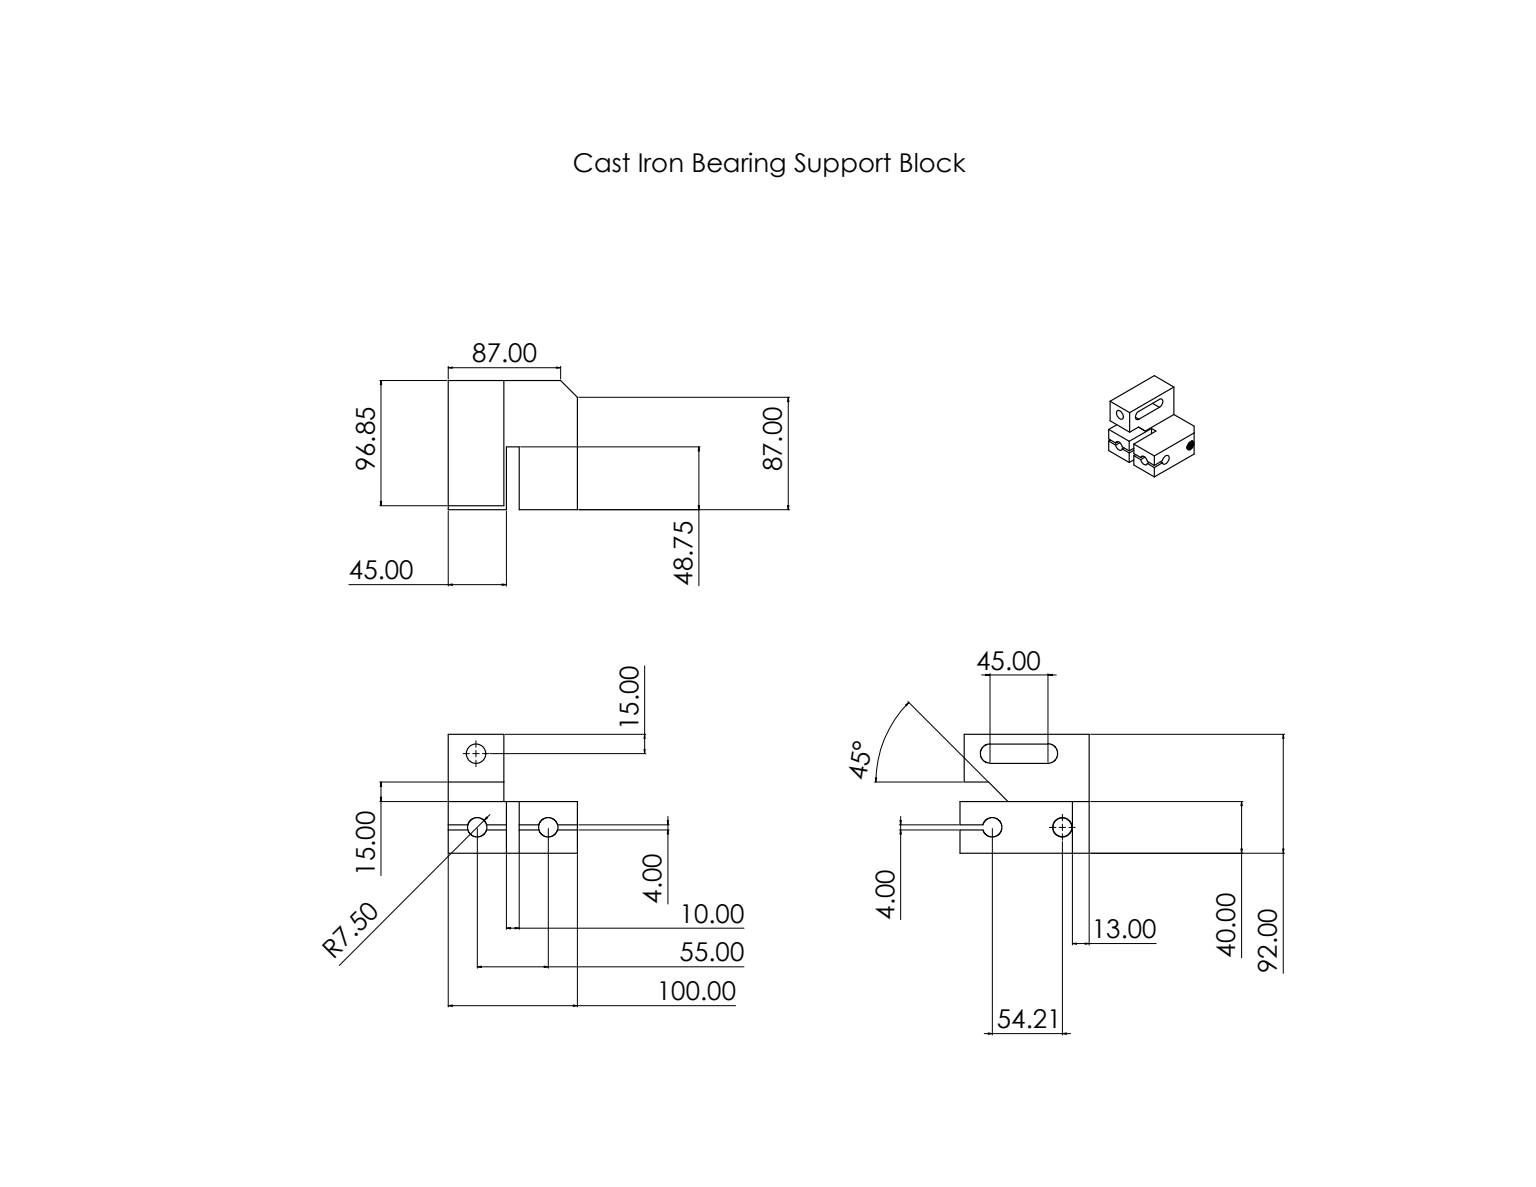
ISO-10303-21;
HEADER;
FILE_DESCRIPTION (('STEP AP214'),
    '1' );
FILE_NAME ('Cast Iron Bearing Support Block.step',
    '2026-10-19T17:36:30',
    ( '' ),
    ( '' ),
    'SwSTEP 2.0',
    'SolidWorks 2025',
    '' );
FILE_SCHEMA (( 'AUTOMOTIVE_DESIGN' ));
ENDSEC;

DATA;
#1=CARTESIAN_POINT ( 'NONE',  ( 38.97500000054622404, 24.28113015263587471, 84.90069139318163138 ) ) ;
#2=CARTESIAN_POINT ( 'NONE',  ( 27.17500000054621978, 26.19570976099943493, 86.29171490190961435 ) ) ;
#3=CARTESIAN_POINT ( 'NONE',  ( 23.09999999999998721, 22.43689772174679575, 83.29316153445363113 ) ) ;
#4=CARTESIAN_POINT ( 'NONE',  ( 19.93750000027310421, 20.00000000000000355, 98.18490835945361539 ) ) ;
#5=CARTESIAN_POINT ( 'NONE',  ( 32.97500000054622404, 24.28113015263587471, 84.90069139318163138 ) ) ;
#6=ORIENTED_EDGE ( 'NONE', *, *, #525, .T. ) ;
#10=VERTEX_POINT ( 'NONE', #4037 ) ;
#11=CARTESIAN_POINT ( 'NONE',  ( 49.45000000109246940, 24.40838939219354842, 96.86078899226572503 ) ) ;
#13=CARTESIAN_POINT ( 'NONE',  ( 43.29999999999999005, 26.37988106264029398, 86.15790661882942914 ) ) ;
#16=CARTESIAN_POINT ( 'NONE',  ( 43.67500000054621978, 24.28113015263587116, 96.68563167572563088 ) ) ;
#19=CARTESIAN_POINT ( 'NONE',  ( -50.00000000000001421, 18.00000000000000355, 188.4007504869563263 ) ) ;
#20=CARTESIAN_POINT ( 'NONE',  ( 46.77500000054622831, 17.63344945572770328, 83.50966788445364841 ) ) ;
#21=CARTESIAN_POINT ( 'NONE',  ( 48.49999999999999289, 12.11403331821300533, 90.79316153445363113 ) ) ;
#22=DIRECTION ( 'NONE',  ( -1.000000000000000000, -9.251858538542971828E-16, 0.000000000000000000 ) ) ;
#23=CARTESIAN_POINT ( 'NONE',  ( 44.29999999999999005, 13.62011893735970958, 95.42841645007781892 ) ) ;
#24=ORIENTED_EDGE ( 'NONE', *, *, #11626, .T. ) ;
#25=CARTESIAN_POINT ( 'NONE',  ( 31.75000000109246656, 17.56310227825320425, 98.29316153445363113 ) ) ;
#27=ORIENTED_EDGE ( 'NONE', *, *, #5795, .F. ) ;
#31=CARTESIAN_POINT ( 'NONE',  ( -27.49999999999999645, 20.00000000000000355, 169.9999999999999716 ) ) ;
#33=CARTESIAN_POINT ( 'NONE',  ( -2.000000000000015543, 20.00000000000000355, 83.29316153445364534 ) ) ;
#34=CARTESIAN_POINT ( 'NONE',  ( 36.27500000054623541, 12.34168156654572535, 90.79316153445363113 ) ) ;
#35=CARTESIAN_POINT ( 'NONE',  ( 34.77500000054622831, 17.63344945572770328, 83.50966788445364841 ) ) ;
#37=CARTESIAN_POINT ( 'NONE',  ( 35.55000000109245661, 22.43689772174678154, 98.29316153445364534 ) ) ;
#40=ORIENTED_EDGE ( 'NONE', *, *, #1850, .F. ) ;
#41=CARTESIAN_POINT ( 'NONE',  ( 48.57500000054622546, 13.80429023900056684, 86.29171490190961435 ) ) ;
#44=DIRECTION ( 'NONE',  ( 0.000000000000000000, 0.000000000000000000, -1.000000000000000000 ) ) ;
#45=DIRECTION ( 'NONE',  ( -1.000000000000000000, 0.000000000000000000, -0.000000000000000000 ) ) ;
#48=CARTESIAN_POINT ( 'NONE',  ( 43.05000000109246372, 27.13292387221364876, 88.47553407664153724 ) ) ;
#51=CARTESIAN_POINT ( 'NONE',  ( 6.614339767079327359, 27.50003396314175674, 91.05027562884485803 ) ) ;
#52=CARTESIAN_POINT ( 'NONE',  ( 37.79999999999998295, 24.40838939219354842, 96.86078899226572503 ) ) ;
#53=VECTOR ( 'NONE', #12398, 999.9999999999998863 ) ;
#54=CARTESIAN_POINT ( 'NONE',  ( 49.99999999999998579, 22.00000000000000000, 169.9999999999999716 ) ) ;
#58=VERTEX_POINT ( 'NONE', #304 ) ;
#59=CARTESIAN_POINT ( 'NONE',  ( 37.25000000109246656, 27.13292387221364876, 93.11078899226573924 ) ) ;
#61=CARTESIAN_POINT ( 'NONE',  ( 23.07500000054622546, 24.28113015263587471, 84.90069139318163138 ) ) ;
#62=CARTESIAN_POINT ( 'NONE',  ( 23.85000000109246443, 15.59161060780645691, 96.86078899226572503 ) ) ;
#63=VECTOR ( 'NONE', #11751, 1000.000000000000000 ) ;
#64=CARTESIAN_POINT ( 'NONE',  ( 37.57500000054622546, 24.28113015263587116, 96.68563167572563088 ) ) ;
#65=CARTESIAN_POINT ( 'NONE',  ( 21.57500000054622546, 26.19570976099943493, 95.29460816699764791 ) ) ;
#66=CARTESIAN_POINT ( 'NONE',  ( 21.49999999999998224, 27.88596668178699645, 90.79316153445363113 ) ) ;
#68=CARTESIAN_POINT ( 'NONE',  ( 31.47500000054623115, 26.19570976099943493, 95.29460816699764791 ) ) ;
#69=ORIENTED_EDGE ( 'NONE', *, *, #4429, .F. ) ;
#70=LINE ( 'NONE', #9907, #9738 ) ;
#73=EDGE_LOOP ( 'NONE', ( #2091, #4719, #3113, #69, #4677 ) ) ;
#77=DIRECTION ( 'NONE',  ( 1.000000000000000000, -0.000000000000000000, -0.000000000000000000 ) ) ;
#79=CARTESIAN_POINT ( 'NONE',  ( -2.000000000000015543, 20.00000000000000355, 90.79316153445363113 ) ) ;
#80=CARTESIAN_POINT ( 'NONE',  ( 44.17500000054621978, 13.80429023900056507, 95.29460816699764791 ) ) ;
#81=CARTESIAN_POINT ( 'NONE',  ( 39.95000000109245519, 13.62011893735970958, 95.42841645007781892 ) ) ;
#82=DIRECTION ( 'NONE',  ( 0.000000000000000000, 0.000000000000000000, -1.000000000000000000 ) ) ;
#83=CARTESIAN_POINT ( 'NONE',  ( 45.47500000054622404, 26.92701409722686634, 93.04388485072563242 ) ) ;
#84=CARTESIAN_POINT ( 'NONE',  ( 45.29999999999999005, 26.37988106264029398, 86.15790661882942914 ) ) ;
#87=CARTESIAN_POINT ( 'NONE',  ( 44.99999999999999289, 20.00000000000000355, 83.29316153445364534 ) ) ;
#88=CARTESIAN_POINT ( 'NONE',  ( 44.09999999999999432, 17.56310227825318648, 98.29316153445363113 ) ) ;
#91=CARTESIAN_POINT ( 'NONE',  ( 31.65000000109246514, 20.00000000000000355, 98.29316153445363113 ) ) ;
#92=DIRECTION ( 'NONE',  ( -1.000000000000000000, 0.000000000000000000, 0.000000000000000000 ) ) ;
#93=EDGE_LOOP ( 'NONE', ( #11616, #6758, #10652, #3781, #4940 ) ) ;
#94=EDGE_CURVE ( 'NONE', #11777, #315, #4411, .T. ) ;
#95=ORIENTED_EDGE ( 'NONE', *, *, #9864, .T. ) ;
#96=DIRECTION ( 'NONE',  ( 1.000000000000000000, -0.000000000000000000, -0.000000000000000000 ) ) ;
#101=CARTESIAN_POINT ( 'NONE',  ( 38.37500000054622973, 13.07298590277314432, 88.54243821818161564 ) ) ;
#102=CARTESIAN_POINT ( 'NONE',  ( 31.17500000054621978, 26.19570976099943493, 86.29171490190961435 ) ) ;
#103=CARTESIAN_POINT ( 'NONE',  ( 34.65000000109246514, 20.00000000000000355, 83.29316153445364534 ) ) ;
#107=CARTESIAN_POINT ( 'NONE',  ( 49.77500000054621410, 22.36655054427230027, 98.07665518445361386 ) ) ;
#109=LINE ( 'NONE', #11712, #6790 ) ;
#110=VERTEX_POINT ( 'NONE', #7455 ) ;
#111=CARTESIAN_POINT ( 'NONE',  ( 31.89339828220178674, 12.50000000000000888, 140.6066017177982133 ) ) ;
#113=VERTEX_POINT ( 'NONE', #8411 ) ;
#114=EDGE_LOOP ( 'NONE', ( #10765, #3378, #1409, #9629, #7659 ) ) ;
#116=CARTESIAN_POINT ( 'NONE',  ( -34.72841614740048044, 22.00000000000000000, 152.2284161474004520 ) ) ;
#118=CARTESIAN_POINT ( 'NONE',  ( 6.732665147703623454, 27.39438278699427087, 92.07235497779568334 ) ) ;
#123=CARTESIAN_POINT ( 'NONE',  ( 43.27500000054623541, 27.65831843345427998, 90.79316153445363113 ) ) ;
#125=CARTESIAN_POINT ( 'NONE',  ( 27.49999999999999645, 20.00000000000000355, 169.9999999999999716 ) ) ;
#129=CARTESIAN_POINT ( 'NONE',  ( 46.19999999999998863, 15.59161060780645691, 96.86078899226572503 ) ) ;
#131=CARTESIAN_POINT ( 'NONE',  ( 30.37500000054622973, 13.07298590277314432, 88.54243821818161564 ) ) ;
#132=CARTESIAN_POINT ( 'NONE',  ( 22.17500000054622333, 13.80429023900056507, 95.29460816699764791 ) ) ;
#133=CARTESIAN_POINT ( 'NONE',  ( 24.89999999999999147, 17.56310227825321135, 83.29316153445363113 ) ) ;
#135=CARTESIAN_POINT ( 'NONE',  ( 33.07500000054623257, 26.19570976099943493, 86.29171490190961435 ) ) ;
#136=VERTEX_POINT ( 'NONE', #11263 ) ;
#137=DIRECTION ( 'NONE',  ( 0.000000000000000000, -0.000000000000000000, 1.000000000000000000 ) ) ;
#140=DIRECTION ( 'NONE',  ( 1.000000000000000000, -0.000000000000000000, -0.000000000000000000 ) ) ;
#146=CARTESIAN_POINT ( 'NONE',  ( 38.17500000054622689, 13.80429023900056507, 95.29460816699764791 ) ) ;
#148=CARTESIAN_POINT ( 'NONE',  ( 26.79999999999998650, 15.59161060780646046, 84.72553407664153724 ) ) ;
#149=CARTESIAN_POINT ( 'NONE',  ( 42.07500000054622546, 15.71886984736413417, 96.68563167572563088 ) ) ;
#150=CARTESIAN_POINT ( 'NONE',  ( 43.89999999999999147, 22.43689772174679575, 98.29316153445363113 ) ) ;
#152=LINE ( 'NONE', #11692, #6762 ) ;
#154=ORIENTED_EDGE ( 'NONE', *, *, #8754, .F. ) ;
#155=CARTESIAN_POINT ( 'NONE',  ( 33.65000000109246514, 20.00000000000000355, 98.29316153445363113 ) ) ;
#159=CARTESIAN_POINT ( 'NONE',  ( 25.65000000109246514, 20.00000000000000355, 98.29316153445363113 ) ) ;
#162=DIRECTION ( 'NONE',  ( 1.000000000000000000, -0.000000000000000000, -0.000000000000000000 ) ) ;
#163=CARTESIAN_POINT ( 'NONE',  ( 48.09999999999999432, 17.56310227825322556, 98.29316153445364534 ) ) ;
#164=CARTESIAN_POINT ( 'NONE',  ( 32.87500000054622973, 22.36655054427230382, 83.50966788445364841 ) ) ;
#165=CARTESIAN_POINT ( 'NONE',  ( 29.87500000054622618, 20.00000000000000355, 98.07665518445361386 ) ) ;
#167=CARTESIAN_POINT ( 'NONE',  ( 44.05000000109246372, 12.86707612778636012, 93.11078899226572503 ) ) ;
#171=CARTESIAN_POINT ( 'NONE',  ( 21.99999999999998934, 20.00000000000000355, 98.29316153445363113 ) ) ;
#172=ORIENTED_EDGE ( 'NONE', *, *, #1724, .F. ) ;
#176=ORIENTED_EDGE ( 'NONE', *, *, #7484, .F. ) ;
#179=EDGE_CURVE ( 'NONE', #6763, #7138, #1054, .T. ) ;
#180=CARTESIAN_POINT ( 'NONE',  ( 9.920725400334921673, 21.28151498972171751, 98.18721253656565295 ) ) ;
#181=LINE ( 'NONE', #4040, #1401 ) ;
#186=CARTESIAN_POINT ( 'NONE',  ( 40.67500000054623399, 17.63344945572770328, 83.50966788445364841 ) ) ;
#187=DIRECTION ( 'NONE',  ( 0.000000000000000000, 0.000000000000000000, 1.000000000000000000 ) ) ;
#189=EDGE_CURVE ( 'NONE', #5728, #3198, #1007, .T. ) ;
#193=CARTESIAN_POINT ( 'NONE',  ( 20.47500000054622404, 13.07298590277314432, 88.54243821818161564 ) ) ;
#195=CARTESIAN_POINT ( 'NONE',  ( 32.57500000054623257, 15.71886984736413773, 84.90069139318163138 ) ) ;
#198=CARTESIAN_POINT ( 'NONE',  ( 23.79999999999998650, 24.40838939219354842, 96.86078899226572503 ) ) ;
#199=CARTESIAN_POINT ( 'NONE',  ( 4.999999999999997335, 20.00000000000000000, 145.0000000000000000 ) ) ;
#200=CARTESIAN_POINT ( 'NONE',  ( 32.27500000054622831, 12.34168156654572535, 90.79316153445363113 ) ) ;
#201=ORIENTED_EDGE ( 'NONE', *, *, #4123, .F. ) ;
#207=DIRECTION ( 'NONE',  ( 1.000000000000000000, 0.000000000000000000, 0.000000000000000000 ) ) ;
#210=CARTESIAN_POINT ( 'NONE',  ( 39.07500000054622546, 24.28113015263587471, 84.90069139318163138 ) ) ;
#211=CARTESIAN_POINT ( 'NONE',  ( 40.35000000109246088, 13.62011893735970958, 86.15790661882942914 ) ) ;
#212=ADVANCED_FACE ( 'NONE', ( #2945 ), #5804, .F. ) ;
#214=CARTESIAN_POINT ( 'NONE',  ( 42.17500000054623399, 13.80429023900056507, 95.29460816699764791 ) ) ;
#215=CARTESIAN_POINT ( 'NONE',  ( 43.79999999999999005, 24.40838939219354842, 96.86078899226572503 ) ) ;
#217=CARTESIAN_POINT ( 'NONE',  ( 39.59999999999998721, 27.13292387221364876, 93.11078899226573924 ) ) ;
#218=CARTESIAN_POINT ( 'NONE',  ( -20.00000000000000355, 15.60660171779822569, 137.5000000000000000 ) ) ;
#220=CARTESIAN_POINT ( 'NONE',  ( 30.85000000109246443, 24.40838939219355197, 84.72553407664153724 ) ) ;
#223=VERTEX_POINT ( 'NONE', #1985 ) ;
#225=CYLINDRICAL_SURFACE ( 'NONE', #7691, 7.499999999999992895 ) ;
#227=CARTESIAN_POINT ( 'NONE',  ( -34.72841614740048044, 22.00000000000000000, 169.9999999999999716 ) ) ;
#228=PLANE ( 'NONE',  #9406 ) ;
#229=CARTESIAN_POINT ( 'NONE',  ( 27.97500000054623115, 15.71886984736413417, 96.68563167572563088 ) ) ;
#230=CARTESIAN_POINT ( 'NONE',  ( 33.87500000054622262, 20.00000000000000355, 98.07665518445361386 ) ) ;
#232=CARTESIAN_POINT ( 'NONE',  ( 31.89339828220179385, 27.49999999999999645, 140.6066017177982133 ) ) ;
#234=AXIS2_PLACEMENT_3D ( 'NONE', #11522, #6698, #10625 ) ;
#236=CARTESIAN_POINT ( 'NONE',  ( 49.65000000109246514, 20.00000000000000355, 98.29316153445363113 ) ) ;
#237=LINE ( 'NONE', #8918, #9432 ) ;
#238=ORIENTED_EDGE ( 'NONE', *, *, #11054, .T. ) ;
#241=CARTESIAN_POINT ( 'NONE',  ( -27.49999999999999645, 12.50000000000001066, 145.0000000000000000 ) ) ;
#244=DIRECTION ( 'NONE',  ( 0.000000000000000000, 0.000000000000000000, 1.000000000000000000 ) ) ;
#246=CARTESIAN_POINT ( 'NONE',  ( 9.617918704988914769, 22.74817246778840385, 83.81039675207235007 ) ) ;
#249=DIRECTION ( 'NONE',  ( 1.000000000000000000, -0.000000000000000000, -0.000000000000000000 ) ) ;
#251=CARTESIAN_POINT ( 'NONE',  ( 44.67500000054623399, 17.63344945572770328, 83.50966788445364841 ) ) ;
#253=ORIENTED_EDGE ( 'NONE', *, *, #2837, .F. ) ;
#257=CARTESIAN_POINT ( 'NONE',  ( 21.87500000054622618, 20.00000000000000355, 98.07665518445361386 ) ) ;
#259=CARTESIAN_POINT ( 'NONE',  ( 31.27500000054622831, 27.65831843345427998, 90.79316153445363113 ) ) ;
#260=( BOUNDED_CURVE ( )  B_SPLINE_CURVE ( 2, ( #4396, #8213, #3321, #10235, #5421, #7127, #353, #8339, #12082, #5358, #12143 ),
 .UNSPECIFIED., .F., .F. ) 
 B_SPLINE_CURVE_WITH_KNOTS ( ( 3, 2, 2, 2, 2, 3 ),
 ( 0.4333333333333334592, 0.4400000000000000577, 0.4466666666666667118, 0.4533333333333333104, 0.4600000000000000200, 0.4666666666666666186 ),
 .UNSPECIFIED. ) 
 CURVE ( )  GEOMETRIC_REPRESENTATION_ITEM ( )  RATIONAL_B_SPLINE_CURVE ( ( 0.9999999999999992228, 0.9510565162951543083, 1.000000000000000000, 0.9510565162951535312, 1.000000000000000000, 0.9510565162951535312, 1.000000000000000000, 0.9510565162951535312, 1.000000000000000000, 0.9510565162951539753, 0.9999999999999995559 ) ) 
 REPRESENTATION_ITEM ( '' )  );
#261=EDGE_CURVE ( 'NONE', #12355, #6453, #10609, .T. ) ;
#262=CARTESIAN_POINT ( 'NONE',  ( 22.97500000054622049, 22.36655054427230382, 83.50966788445364841 ) ) ;
#263=CARTESIAN_POINT ( 'NONE',  ( 23.19999999999998863, 24.40838939219355197, 84.72553407664153724 ) ) ;
#264=LINE ( 'NONE', #9078, #7887 ) ;
#265=CARTESIAN_POINT ( 'NONE',  ( 24.47500000054623115, 13.80429023900056684, 86.29171490190961435 ) ) ;
#266=EDGE_LOOP ( 'NONE', ( #3910, #10160, #3333, #10971 ) ) ;
#271=DIRECTION ( 'NONE',  ( 0.000000000000000000, 1.000000000000000000, 0.000000000000000000 ) ) ;
#272=VECTOR ( 'NONE', #1470, 1000.000000000000000 ) ;
#273=CARTESIAN_POINT ( 'NONE',  ( 40.87500000054622262, 20.00000000000000355, 83.50966788445364841 ) ) ;
#274=DIRECTION ( 'NONE',  ( 0.000000000000000000, 0.000000000000000000, -1.000000000000000000 ) ) ;
#276=CARTESIAN_POINT ( 'NONE',  ( 41.69999999999998863, 26.37988106264029398, 95.42841645007781892 ) ) ;
#277=CARTESIAN_POINT ( 'NONE',  ( 45.77500000054622831, 20.00000000000000355, 98.07665518445361386 ) ) ;
#280=CARTESIAN_POINT ( 'NONE',  ( 28.65000000109246514, 20.00000000000000355, 83.29316153445364534 ) ) ;
#283=PLANE ( 'NONE',  #2263 ) ;
#288=VECTOR ( 'NONE', #6310, 1000.000000000000000 ) ;
#290=CARTESIAN_POINT ( 'NONE',  ( 31.57500000054622902, 24.28113015263587116, 96.68563167572563088 ) ) ;
#291=CARTESIAN_POINT ( 'NONE',  ( 28.77500000054622831, 17.63344945572770328, 83.50966788445364841 ) ) ;
#294=CARTESIAN_POINT ( 'NONE',  ( 20.00000000000003908, 20.00000000000000000, 137.5000000000000000 ) ) ;
#297=CARTESIAN_POINT ( 'NONE',  ( 48.77500000054623541, 17.63344945572770328, 83.50966788445364841 ) ) ;
#300=CARTESIAN_POINT ( 'NONE',  ( -50.00000000000001421, 84.49999999999998579, 146.8533255156881978 ) ) ;
#301=ORIENTED_EDGE ( 'NONE', *, *, #8138, .T. ) ;
#304=CARTESIAN_POINT ( 'NONE',  ( 30.65000000109246514, 20.00000000000000355, 83.29316153445364534 ) ) ;
#307=CARTESIAN_POINT ( 'NONE',  ( 8.247655429682051675, 25.65770512295588901, 95.72222997683927304 ) ) ;
#308=DIRECTION ( 'NONE',  ( 0.000000000000000000, 0.000000000000000000, -1.000000000000000000 ) ) ;
#309=( GEOMETRIC_REPRESENTATION_CONTEXT ( 3 ) GLOBAL_UNCERTAINTY_ASSIGNED_CONTEXT ( ( #9884 ) ) GLOBAL_UNIT_ASSIGNED_CONTEXT ( ( #2929, #7943, #11807 ) ) REPRESENTATION_CONTEXT ( 'NONE', 'WORKASPACE' ) );
#313=CARTESIAN_POINT ( 'NONE',  ( 45.37500000054622973, 26.92701409722686634, 93.04388485072563242 ) ) ;
#315=VERTEX_POINT ( 'NONE', #6684 ) ;
#320=CARTESIAN_POINT ( 'NONE',  ( 19.87500000054622262, 20.00000000000000355, 98.07665518445361386 ) ) ;
#321=CARTESIAN_POINT ( 'NONE',  ( 43.57500000054623257, 26.19570976099943493, 95.29460816699764791 ) ) ;
#322=CARTESIAN_POINT ( 'NONE',  ( 31.17500000054622689, 26.92701409722686634, 88.54243821818162985 ) ) ;
#323=CARTESIAN_POINT ( 'NONE',  ( 20.07500000054622546, 15.71886984736413417, 96.68563167572563088 ) ) ;
#326=CARTESIAN_POINT ( 'NONE',  ( 27.37500000054622973, 26.92701409722686634, 93.04388485072563242 ) ) ;
#327=ORIENTED_EDGE ( 'NONE', *, *, #6078, .F. ) ;
#330=ORIENTED_EDGE ( 'NONE', *, *, #8043, .T. ) ;
#331=CARTESIAN_POINT ( 'NONE',  ( 38.69999999999998863, 13.62011893735970958, 86.15790661882942914 ) ) ;
#336=( BOUNDED_CURVE ( )  B_SPLINE_CURVE ( 2, ( #10274, #1591, #10398, #642, #4505, #8380, #11296, #10334, #1651, #701, #4568 ),
 .UNSPECIFIED., .F., .F. ) 
 B_SPLINE_CURVE_WITH_KNOTS ( ( 3, 2, 2, 2, 2, 3 ),
 ( 0.7333333333333332815, 0.7399999999999999911, 0.7466666666666667007, 0.7533333333333331883, 0.7599999999999998979, 0.7666666666666666075 ),
 .UNSPECIFIED. ) 
 CURVE ( )  GEOMETRIC_REPRESENTATION_ITEM ( )  RATIONAL_B_SPLINE_CURVE ( ( 1.000000000000000000, 0.9510565162951535312, 1.000000000000000000, 0.9510565162951535312, 1.000000000000000000, 0.9510565162951535312, 1.000000000000000000, 0.9510565162951535312, 1.000000000000000000, 0.9510565162951543083, 0.9999999999999992228 ) ) 
 REPRESENTATION_ITEM ( '' )  );
#337=CARTESIAN_POINT ( 'NONE',  ( 39.27500000054622831, 26.92701409722686634, 88.54243821818162985 ) ) ;
#341=CARTESIAN_POINT ( 'NONE',  ( 38.17500000054622689, 13.80429023900056507, 95.29460816699764791 ) ) ;
#342=CARTESIAN_POINT ( 'NONE',  ( 41.09999999999999432, 22.43689772174679575, 83.29316153445363113 ) ) ;
#344=CARTESIAN_POINT ( 'NONE',  ( 48.27500000054622120, 12.34168156654572535, 90.79316153445363113 ) ) ;
#346=CARTESIAN_POINT ( 'NONE',  ( 23.15000000109246514, 27.88596668178699645, 90.79316153445363113 ) ) ;
#353=CARTESIAN_POINT ( 'NONE',  ( 36.05000000109246372, 12.86707612778636012, 93.11078899226572503 ) ) ;
#354=CARTESIAN_POINT ( 'NONE',  ( 48.19999999999998863, 15.59161060780645691, 96.86078899226572503 ) ) ;
#356=CARTESIAN_POINT ( 'NONE',  ( 30.47500000054622404, 13.80429023900056684, 86.29171490190961435 ) ) ;
#357=CARTESIAN_POINT ( 'NONE',  ( 29.27500000054622475, 26.92701409722686634, 88.54243821818162985 ) ) ;
#359=CARTESIAN_POINT ( 'NONE',  ( 21.85000000109246443, 15.59161060780645691, 96.86078899226572503 ) ) ;
#361=CARTESIAN_POINT ( 'NONE',  ( 45.95000000109245519, 13.62011893735971135, 95.42841645007781892 ) ) ;
#363=ORIENTED_EDGE ( 'NONE', *, *, #6657, .F. ) ;
#365=ADVANCED_FACE ( 'NONE', ( #7062 ), #4979, .F. ) ;
#372=ADVANCED_FACE ( 'NONE', ( #11955 ), #8150, .F. ) ;
#382=CARTESIAN_POINT ( 'NONE',  ( 44.77500000054622831, 17.63344945572770328, 83.50966788445364841 ) ) ;
#383=CARTESIAN_POINT ( 'NONE',  ( 33.77500000054622831, 20.00000000000000355, 98.07665518445361386 ) ) ;
#385=CARTESIAN_POINT ( 'NONE',  ( 8.252517838734652500, 14.33883749563042720, 95.73505295065133680 ) ) ;
#387=CYLINDRICAL_SURFACE ( 'NONE', #2812, 7.499999999999992895 ) ;
#388=CARTESIAN_POINT ( 'NONE',  ( 23.67500000054622333, 22.36655054427230027, 98.07665518445361386 ) ) ;
#390=AXIS2_PLACEMENT_3D ( 'NONE', #10424, #8591, #2756 ) ;
#391=EDGE_CURVE ( 'NONE', #3772, #2249, #5044, .T. ) ;
#392=DIRECTION ( 'NONE',  ( 0.000000000000000000, 0.000000000000000000, -1.000000000000000000 ) ) ;
#396=EDGE_CURVE ( 'NONE', #10590, #5728, #12016, .T. ) ;
#397=CARTESIAN_POINT ( 'NONE',  ( 39.77500000054621410, 22.36655054427230027, 98.07665518445361386 ) ) ;
#400=CARTESIAN_POINT ( 'NONE',  ( 37.77500000054622120, 22.36655054427230027, 98.07665518445361386 ) ) ;
#401=CARTESIAN_POINT ( 'NONE',  ( 34.29999999999996874, 13.62011893735971135, 95.42841645007781892 ) ) ;
#402=CARTESIAN_POINT ( 'NONE',  ( 47.77500000054622831, 20.00000000000000355, 98.07665518445361386 ) ) ;
#403=ORIENTED_EDGE ( 'NONE', *, *, #1195, .F. ) ;
#405=CARTESIAN_POINT ( 'NONE',  ( 25.45000000109246230, 24.40838939219354842, 96.86078899226572503 ) ) ;
#410=CARTESIAN_POINT ( 'NONE',  ( 25.05000000109246727, 27.13292387221364876, 88.47553407664153724 ) ) ;
#411=ADVANCED_FACE ( 'NONE', ( #5172 ), #225, .F. ) ;
#412=CARTESIAN_POINT ( 'NONE',  ( 41.45000000109246940, 24.40838939219354842, 96.86078899226572503 ) ) ;
#414=DIRECTION ( 'NONE',  ( -0.000000000000000000, -1.000000000000000000, -0.000000000000000000 ) ) ;
#415=CARTESIAN_POINT ( 'NONE',  ( 33.27500000054621410, 27.65831843345427998, 90.79316153445363113 ) ) ;
#416=CARTESIAN_POINT ( 'NONE',  ( 24.07500000054622546, 15.71886984736413417, 96.68563167572563088 ) ) ;
#418=EDGE_CURVE ( 'NONE', #8662, #3301, #11169, .T. ) ;
#419=CARTESIAN_POINT ( 'NONE',  ( -2.000000000000015543, 20.00000000000000355, 98.29316153445363113 ) ) ;
#421=CARTESIAN_POINT ( 'NONE',  ( 44.95000000109246940, 26.37988106264029398, 86.15790661882942914 ) ) ;
#423=ORIENTED_EDGE ( 'NONE', *, *, #10684, .T. ) ;
#424=CYLINDRICAL_SURFACE ( 'NONE', #1548, 7.499999999999992895 ) ;
#432=CARTESIAN_POINT ( 'NONE',  ( -50.00000000000001421, 77.00000000000000000, 101.8533255156881978 ) ) ;
#433=DIRECTION ( 'NONE',  ( 1.000000000000000000, -0.000000000000000000, -0.000000000000000000 ) ) ;
#434=CARTESIAN_POINT ( 'NONE',  ( 42.49999999999998579, 12.11403331821300533, 90.79316153445363113 ) ) ;
#437=CARTESIAN_POINT ( 'NONE',  ( 24.65000000109246514, 20.00000000000000355, 83.29316153445364534 ) ) ;
#439=VECTOR ( 'NONE', #5468, 1000.000000000000000 ) ;
#443=CARTESIAN_POINT ( 'NONE',  ( 45.17500000054621978, 26.19570976099943493, 86.29171490190961435 ) ) ;
#444=CARTESIAN_POINT ( 'NONE',  ( 25.07500000054622902, 26.19570976099943849, 86.29171490190961435 ) ) ;
#445=CARTESIAN_POINT ( 'NONE',  ( 9.148278039838693587, 15.95559529756309836, 84.47248762917537590 ) ) ;
#446=LINE ( 'NONE', #12178, #6529 ) ;
#449=CARTESIAN_POINT ( 'NONE',  ( 25.67500000054623044, 22.36655054427230027, 98.07665518445361386 ) ) ;
#450=EDGE_LOOP ( 'NONE', ( #10994, #8391, #10133, #605, #8071 ) ) ;
#451=CARTESIAN_POINT ( 'NONE',  ( 33.65000000109246514, 20.00000000000000355, 98.29316153445363113 ) ) ;
#452=ORIENTED_EDGE ( 'NONE', *, *, #9229, .T. ) ;
#453=( BOUNDED_CURVE ( )  B_SPLINE_CURVE ( 2, ( #5462, #5522, #10208, #12119, #6464, #693, #8432, #7289, #4309, #6522, #8188 ),
 .UNSPECIFIED., .F., .F. ) 
 B_SPLINE_CURVE_WITH_KNOTS ( ( 3, 2, 2, 2, 2, 3 ),
 ( 0.5333333333333333259, 0.5400000000000000355, 0.5466666666666666341, 0.5533333333333333437, 0.5600000000000000533, 0.5666666666666666519 ),
 .UNSPECIFIED. ) 
 CURVE ( )  GEOMETRIC_REPRESENTATION_ITEM ( )  RATIONAL_B_SPLINE_CURVE ( ( 1.000000000000000000, 0.9510565162951535312, 1.000000000000000000, 0.9510565162951535312, 1.000000000000000000, 0.9510565162951535312, 1.000000000000000000, 0.9510565162951535312, 1.000000000000000000, 0.9510565162951535312, 1.000000000000000000 ) ) 
 REPRESENTATION_ITEM ( '' )  );
#454=DIRECTION ( 'NONE',  ( 1.000000000000000000, -0.000000000000000000, -0.000000000000000000 ) ) ;
#456=EDGE_CURVE ( 'NONE', #3312, #5229, #7002, .T. ) ;
#458=CARTESIAN_POINT ( 'NONE',  ( 29.27500000054622475, 26.92701409722686634, 88.54243821818162985 ) ) ;
#460=CARTESIAN_POINT ( 'NONE',  ( 47.07500000054621836, 26.19570976099943849, 86.29171490190961435 ) ) ;
#461=CARTESIAN_POINT ( 'NONE',  ( 34.17500000054622689, 13.80429023900056507, 95.29460816699764791 ) ) ;
#462=CARTESIAN_POINT ( 'NONE',  ( 38.19999999999998863, 15.59161060780645691, 96.86078899226572503 ) ) ;
#463=CARTESIAN_POINT ( 'NONE',  ( 45.07500000054621836, 26.19570976099943493, 86.29171490190961435 ) ) ;
#464=ORIENTED_EDGE ( 'NONE', *, *, #8533, .T. ) ;
#465=CARTESIAN_POINT ( 'NONE',  ( 24.05000000109246372, 12.86707612778636012, 93.11078899226572503 ) ) ;
#476=CARTESIAN_POINT ( 'NONE',  ( 24.57500000054622902, 15.71886984736413773, 84.90069139318163138 ) ) ;
#477=CARTESIAN_POINT ( 'NONE',  ( 26.97500000054622049, 22.36655054427230382, 83.50966788445364841 ) ) ;
#480=LINE ( 'NONE', #419, #10100 ) ;
#482=EDGE_CURVE ( 'NONE', #3396, #3276, #2495, .T. ) ;
#483=CARTESIAN_POINT ( 'NONE',  ( 41.95000000109246230, 13.62011893735971135, 95.42841645007781892 ) ) ;
#485=EDGE_LOOP ( 'NONE', ( #8313, #8253, #1494, #12322 ) ) ;
#487=ORIENTED_EDGE ( 'NONE', *, *, #5188, .T. ) ;
#490=EDGE_CURVE ( 'NONE', #5212, #9224, #8457, .T. ) ;
#492=CARTESIAN_POINT ( 'NONE',  ( 29.49999999999998934, 27.88596668178699645, 90.79316153445363113 ) ) ;
#496=AXIS2_PLACEMENT_3D ( 'NONE', #5549, #658, #12392 ) ;
#503=ORIENTED_EDGE ( 'NONE', *, *, #3690, .F. ) ;
#508=CARTESIAN_POINT ( 'NONE',  ( 43.07500000054622546, 24.28113015263587471, 84.90069139318163138 ) ) ;
#509=CARTESIAN_POINT ( 'NONE',  ( 23.77500000054622831, 20.00000000000000355, 98.07665518445361386 ) ) ;
#511=DIRECTION ( 'NONE',  ( 0.000000000000000000, -1.000000000000000000, 0.000000000000000000 ) ) ;
#512=CARTESIAN_POINT ( 'NONE',  ( 35.79999999999998295, 24.40838939219354842, 96.86078899226572503 ) ) ;
#513=VERTEX_POINT ( 'NONE', #656 ) ;
#514=CYLINDRICAL_SURFACE ( 'NONE', #5694, 7.499999999999992895 ) ;
#515=ORIENTED_EDGE ( 'NONE', *, *, #5886, .T. ) ;
#519=CARTESIAN_POINT ( 'NONE',  ( 31.47500000054622404, 26.92701409722686634, 93.04388485072563242 ) ) ;
#521=CARTESIAN_POINT ( 'NONE',  ( 44.97500000054623115, 24.28113015263587471, 84.90069139318163138 ) ) ;
#522=CARTESIAN_POINT ( 'NONE',  ( 33.17500000054622689, 26.19570976099943493, 86.29171490190961435 ) ) ;
#523=CARTESIAN_POINT ( 'NONE',  ( 35.29999999999998295, 26.37988106264029398, 86.15790661882942914 ) ) ;
#525=EDGE_CURVE ( 'NONE', #6104, #2798, #9416, .T. ) ;
#526=CARTESIAN_POINT ( 'NONE',  ( 44.57500000054622546, 15.71886984736413773, 84.90069139318163138 ) ) ;
#527=VERTEX_POINT ( 'NONE', #11245 ) ;
#528=CARTESIAN_POINT ( 'NONE',  ( 25.05000000109246727, 27.13292387221364876, 88.47553407664153724 ) ) ;
#530=ORIENTED_EDGE ( 'NONE', *, *, #11604, .T. ) ;
#532=EDGE_LOOP ( 'NONE', ( #1378, #12293, #3921, #6914, #8507 ) ) ;
#533=PLANE ( 'NONE',  #4547 ) ;
#537=CARTESIAN_POINT ( 'NONE',  ( 22.07500000054622546, 13.80429023900056507, 95.29460816699764791 ) ) ;
#538=CARTESIAN_POINT ( 'NONE',  ( 24.87500000054622262, 20.00000000000000355, 83.50966788445364841 ) ) ;
#542=CARTESIAN_POINT ( 'NONE',  ( 46.85000000109246798, 24.40838939219355197, 84.72553407664153724 ) ) ;
#545=CARTESIAN_POINT ( 'NONE',  ( 29.85000000109246443, 15.59161060780645691, 96.86078899226572503 ) ) ;
#547=ORIENTED_EDGE ( 'NONE', *, *, #2008, .F. ) ;
#551=DIRECTION ( 'NONE',  ( 1.000000000000000000, 0.000000000000000000, 0.000000000000000000 ) ) ;
#554=CARTESIAN_POINT ( 'NONE',  ( 42.39999999999998437, 12.86707612778636012, 93.11078899226572503 ) ) ;
#556=DIRECTION ( 'NONE',  ( -1.000000000000000000, -0.000000000000000000, 0.000000000000000000 ) ) ;
#559=ORIENTED_EDGE ( 'NONE', *, *, #3887, .F. ) ;
#561=EDGE_CURVE ( 'NONE', #8548, #852, #3785, .T. ) ;
#563=LINE ( 'NONE', #626, #4184 ) ;
#564=CARTESIAN_POINT ( 'NONE',  ( 41.17500000054621978, 26.19570976099943493, 86.29171490190961435 ) ) ;
#565=CARTESIAN_POINT ( 'NONE',  ( 29.97500000054622760, 15.71886984736413417, 96.68563167572563088 ) ) ;
#566=CARTESIAN_POINT ( 'NONE',  ( 8.667493610547218452, 14.99723978859658935, 85.18566974208211207 ) ) ;
#567=CARTESIAN_POINT ( 'NONE',  ( 0.000000000000000000, 18.00000000000000355, 169.9999999999999716 ) ) ;
#569=CARTESIAN_POINT ( 'NONE',  ( -6.999999999999999112, 34.57333724215600768, 127.4266627578445679 ) ) ;
#571=AXIS2_PLACEMENT_3D ( 'NONE', #4157, #3457, #6315 ) ;
#572=ORIENTED_EDGE ( 'NONE', *, *, #5822, .T. ) ;
#574=VERTEX_POINT ( 'NONE', #3382 ) ;
#579=CARTESIAN_POINT ( 'NONE',  ( 31.87500000054622262, 20.00000000000000355, 98.07665518445361386 ) ) ;
#581=CARTESIAN_POINT ( 'NONE',  ( 45.37500000054622973, 26.92701409722686634, 93.04388485072563242 ) ) ;
#582=CARTESIAN_POINT ( 'NONE',  ( 31.47500000054622404, 26.92701409722686634, 93.04388485072563242 ) ) ;
#583=CARTESIAN_POINT ( 'NONE',  ( 33.19999999999998863, 24.40838939219355197, 84.72553407664153724 ) ) ;
#585=CARTESIAN_POINT ( 'NONE',  ( 40.87500000054623683, 22.36655054427230382, 83.50966788445364841 ) ) ;
#586=ORIENTED_EDGE ( 'NONE', *, *, #10084, .T. ) ;
#587=CARTESIAN_POINT ( 'NONE',  ( 46.07500000054623257, 13.80429023900056507, 95.29460816699764791 ) ) ;
#589=VERTEX_POINT ( 'NONE', #2552 ) ;
#596=DIRECTION ( 'NONE',  ( -1.000000000000000000, 0.000000000000000000, 0.000000000000000000 ) ) ;
#598=EDGE_CURVE ( 'NONE', #3966, #5275, #11124, .T. ) ;
#599=CARTESIAN_POINT ( 'NONE',  ( 32.05000000109247082, 12.86707612778636012, 93.11078899226572503 ) ) ;
#600=CARTESIAN_POINT ( 'NONE',  ( 21.47500000054622760, 26.19570976099943493, 95.29460816699764791 ) ) ;
#601=CARTESIAN_POINT ( 'NONE',  ( 27.37500000054622262, 27.65831843345427998, 90.79316153445363113 ) ) ;
#605=ORIENTED_EDGE ( 'NONE', *, *, #1416, .T. ) ;
#606=CARTESIAN_POINT ( 'NONE',  ( 42.25000000109246656, 12.86707612778636012, 88.47553407664152303 ) ) ;
#608=CARTESIAN_POINT ( 'NONE',  ( -2.000000000000015543, 20.00000000000000355, 90.79316153445363113 ) ) ;
#609=EDGE_LOOP ( 'NONE', ( #745, #2763, #10847, #363, #6595 ) ) ;
#613=FACE_OUTER_BOUND ( 'NONE', #1110, .T. ) ;
#615=ADVANCED_FACE ( 'NONE', ( #3449 ), #7315, .F. ) ;
#624=CIRCLE ( 'NONE', #3462, 7.500000000000000000 ) ;
#625=DIRECTION ( 'NONE',  ( 1.000000000000000000, 0.000000000000000000, 0.000000000000000000 ) ) ;
#626=CARTESIAN_POINT ( 'NONE',  ( -2.000000000000015543, 20.00000000000000355, 98.29316153445363113 ) ) ;
#627=CARTESIAN_POINT ( 'NONE',  ( 36.07500000054622546, 15.71886984736413417, 96.68563167572563088 ) ) ;
#628=CARTESIAN_POINT ( 'NONE',  ( 25.67500000054623044, 22.36655054427230027, 98.07665518445361386 ) ) ;
#629=CARTESIAN_POINT ( 'NONE',  ( 7.061248332739769040, 12.91833545835538288, 88.31103790290751476 ) ) ;
#632=DIRECTION ( 'NONE',  ( 0.000000000000000000, 0.000000000000000000, -1.000000000000000000 ) ) ;
#636=DIRECTION ( 'NONE',  ( 0.000000000000000000, 0.000000000000000000, -1.000000000000000000 ) ) ;
#638=FACE_BOUND ( 'NONE', #9288, .T. ) ;
#639=ADVANCED_FACE ( 'NONE', ( #11621 ), #4645, .F. ) ;
#641=CARTESIAN_POINT ( 'NONE',  ( 32.57500000054622546, 13.80429023900056684, 86.29171490190961435 ) ) ;
#642=CARTESIAN_POINT ( 'NONE',  ( 27.35000000109246443, 26.37988106264029398, 95.42841645007781892 ) ) ;
#643=CARTESIAN_POINT ( 'NONE',  ( 47.77500000054622831, 20.00000000000000355, 98.07665518445361386 ) ) ;
#644=CARTESIAN_POINT ( 'NONE',  ( 35.67500000054622689, 24.28113015263587116, 96.68563167572563088 ) ) ;
#645=CARTESIAN_POINT ( 'NONE',  ( 38.49999999999999289, 12.11403331821300533, 90.79316153445363113 ) ) ;
#647=EDGE_CURVE ( 'NONE', #5544, #10865, #2369, .T. ) ;
#648=CARTESIAN_POINT ( 'NONE',  ( 37.37500000054622973, 26.92701409722686634, 93.04388485072563242 ) ) ;
#650=CARTESIAN_POINT ( 'NONE',  ( 48.17500000054623399, 13.07298590277314254, 93.04388485072563242 ) ) ;
#652=VERTEX_POINT ( 'NONE', #11434 ) ;
#654=ORIENTED_EDGE ( 'NONE', *, *, #179, .T. ) ;
#655=CARTESIAN_POINT ( 'NONE',  ( 41.65000000109246514, 20.00000000000000355, 98.29316153445363113 ) ) ;
#656=CARTESIAN_POINT ( 'NONE',  ( 37.99999999999999289, 20.00000000000000355, 98.29316153445363113 ) ) ;
#658=DIRECTION ( 'NONE',  ( 1.000000000000000000, -0.000000000000000000, -0.000000000000000000 ) ) ;
#659=CARTESIAN_POINT ( 'NONE',  ( 23.27500000054622120, 27.65831843345427998, 90.79316153445363113 ) ) ;
#660=CARTESIAN_POINT ( 'NONE',  ( 25.57500000054621836, 26.19570976099943493, 95.29460816699764791 ) ) ;
#661=FACE_OUTER_BOUND ( 'NONE', #1808, .T. ) ;
#662=( BOUNDED_CURVE ( )  B_SPLINE_CURVE ( 2, ( #4095, #9942, #12155, #4408, #11197, #8286, #1618, #7453, #545, #5432, #11137 ),
 .UNSPECIFIED., .F., .F. ) 
 B_SPLINE_CURVE_WITH_KNOTS ( ( 3, 2, 2, 2, 2, 3 ),
 ( 0.6333333333333333037, 0.6400000000000000133, 0.6466666666666666119, 0.6533333333333333215, 0.6600000000000000311, 0.6666666666666666297 ),
 .UNSPECIFIED. ) 
 CURVE ( )  GEOMETRIC_REPRESENTATION_ITEM ( )  RATIONAL_B_SPLINE_CURVE ( ( 1.000000000000000000, 0.9510565162951535312, 1.000000000000000000, 0.9510565162951535312, 1.000000000000000000, 0.9510565162951535312, 1.000000000000000000, 0.9510565162951535312, 1.000000000000000000, 0.9510565162951535312, 1.000000000000000000 ) ) 
 REPRESENTATION_ITEM ( '' )  );
#663=CARTESIAN_POINT ( 'NONE',  ( 44.89999999999998437, 17.56310227825322912, 83.29316153445361692 ) ) ;
#664=ORIENTED_EDGE ( 'NONE', *, *, #6410, .F. ) ;
#665=CARTESIAN_POINT ( 'NONE',  ( 39.15000000109246514, 27.88596668178699645, 90.79316153445363113 ) ) ;
#668=DIRECTION ( 'NONE',  ( 1.000000000000000000, -0.000000000000000000, -0.000000000000000000 ) ) ;
#675=DIRECTION ( 'NONE',  ( 1.000000000000000000, -0.000000000000000000, -0.000000000000000000 ) ) ;
#678=CARTESIAN_POINT ( 'NONE',  ( 29.87500000054622618, 17.63344945572769973, 98.07665518445361386 ) ) ;
#680=LINE ( 'NONE', #5511, #2953 ) ;
#686=CARTESIAN_POINT ( 'NONE',  ( 34.97500000054623115, 24.28113015263587471, 84.90069139318163138 ) ) ;
#687=CARTESIAN_POINT ( 'NONE',  ( 38.57500000054622546, 13.80429023900056684, 86.29171490190961435 ) ) ;
#689=CARTESIAN_POINT ( 'NONE',  ( 26.77500000054622831, 20.00000000000000355, 83.50966788445364841 ) ) ;
#690=DIRECTION ( 'NONE',  ( 0.000000000000000000, 0.000000000000000000, 1.000000000000000000 ) ) ;
#692=CIRCLE ( 'NONE', #8795, 7.499999999999992895 ) ;
#693=CARTESIAN_POINT ( 'NONE',  ( 33.49999999999998579, 27.88596668178699645, 90.79316153445363113 ) ) ;
#696=CARTESIAN_POINT ( 'NONE',  ( 27.49999999999999645, 20.00000000000000355, 170.0000119999999697 ) ) ;
#700=CARTESIAN_POINT ( 'NONE',  ( 27.47500000054622404, 26.92701409722686634, 93.04388485072563242 ) ) ;
#701=CARTESIAN_POINT ( 'NONE',  ( 26.75000000109246656, 22.43689772174683128, 83.29316153445365956 ) ) ;
#702=CARTESIAN_POINT ( 'NONE',  ( 49.17500000054622689, 26.92701409722686634, 88.54243821818162985 ) ) ;
#703=CARTESIAN_POINT ( 'NONE',  ( 32.97500000054621694, 22.36655054427230382, 83.50966788445364841 ) ) ;
#704=CARTESIAN_POINT ( 'NONE',  ( 32.19999999999999574, 15.59161060780645691, 96.86078899226572503 ) ) ;
#706=CARTESIAN_POINT ( 'NONE',  ( 36.87500000054622973, 22.36655054427230382, 83.50966788445364841 ) ) ;
#707=VERTEX_POINT ( 'NONE', #11558 ) ;
#710=CARTESIAN_POINT ( 'NONE',  ( 47.87500000054622973, 17.63344945572769973, 98.07665518445361386 ) ) ;
#712=ORIENTED_EDGE ( 'NONE', *, *, #2572, .T. ) ;
#713=ADVANCED_FACE ( 'NONE', ( #12510 ), #10472, .F. ) ;
#715=ORIENTED_EDGE ( 'NONE', *, *, #4970, .T. ) ;
#719=DIRECTION ( 'NONE',  ( 0.000000000000000000, 0.000000000000000000, -1.000000000000000000 ) ) ;
#720=EDGE_CURVE ( 'NONE', #5074, #10184, #8439, .T. ) ;
#721=CARTESIAN_POINT ( 'NONE',  ( 23.57500000054622902, 24.28113015263587116, 96.68563167572563088 ) ) ;
#722=CARTESIAN_POINT ( 'NONE',  ( 49.29999999999998295, 26.37988106264029398, 86.15790661882942914 ) ) ;
#725=AXIS2_PLACEMENT_3D ( 'NONE', #3592, #2392, #3529 ) ;
#726=CARTESIAN_POINT ( 'NONE',  ( 34.95000000109246940, 26.37988106264029398, 86.15790661882942914 ) ) ;
#727=ORIENTED_EDGE ( 'NONE', *, *, #7144, .F. ) ;
#729=EDGE_CURVE ( 'NONE', #3966, #852, #8760, .T. ) ;
#734=( BOUNDED_CURVE ( )  B_SPLINE_CURVE ( 2, ( #10941, #6123, #9991, #1304, #5174, #9043, #7835, #11704, #354, #163, #11643 ),
 .UNSPECIFIED., .F., .F. ) 
 B_SPLINE_CURVE_WITH_KNOTS ( ( 3, 2, 2, 2, 2, 3 ),
 ( 0.03333333333333336063, 0.04000000000000003553, 0.04666666666666670349, 0.05333333333333337839, 0.06000000000000005329, 0.06666666666666672125 ),
 .UNSPECIFIED. ) 
 CURVE ( )  GEOMETRIC_REPRESENTATION_ITEM ( )  RATIONAL_B_SPLINE_CURVE ( ( 0.9999999999999998890, 0.9510565162951537532, 1.000000000000000000, 0.9510565162951535312, 1.000000000000000000, 0.9510565162951535312, 1.000000000000000000, 0.9510565162951535312, 1.000000000000000000, 0.9510565162951530871, 1.000000000000000444 ) ) 
 REPRESENTATION_ITEM ( '' )  );
#737=EDGE_CURVE ( 'NONE', #5428, #8208, #5928, .T. ) ;
#739=CARTESIAN_POINT ( 'NONE',  ( 48.15000000109246514, 12.11403331821300533, 90.79316153445363113 ) ) ;
#740=CARTESIAN_POINT ( 'NONE',  ( 20.37500000054622618, 13.07298590277314432, 88.54243821818161564 ) ) ;
#742=CARTESIAN_POINT ( 'NONE',  ( 47.55000000109247082, 22.43689772174681707, 98.29316153445361692 ) ) ;
#744=AXIS2_PLACEMENT_3D ( 'NONE', #12233, #8244, #11213 ) ;
#745=ORIENTED_EDGE ( 'NONE', *, *, #3310, .F. ) ;
#749=CARTESIAN_POINT ( 'NONE',  ( 36.77500000054622831, 17.63344945572770328, 83.50966788445364841 ) ) ;
#751=CARTESIAN_POINT ( 'NONE',  ( 22.37500000054622973, 13.07298590277314432, 88.54243821818161564 ) ) ;
#755=DIRECTION ( 'NONE',  ( 0.000000000000000000, 1.000000000000000000, 0.000000000000000000 ) ) ;
#756=ADVANCED_FACE ( 'NONE', ( #9914, #7944 ), #2238, .T. ) ;
#761=CARTESIAN_POINT ( 'NONE',  ( 39.27500000054622120, 27.65831843345427998, 90.79316153445363113 ) ) ;
#762=CARTESIAN_POINT ( 'NONE',  ( 28.47500000054622404, 13.07298590277314432, 88.54243821818161564 ) ) ;
#763=CARTESIAN_POINT ( 'NONE',  ( 29.49999999999998934, 27.88596668178699645, 90.79316153445363113 ) ) ;
#764=EDGE_CURVE ( 'NONE', #9148, #8716, #2992, .T. ) ;
#766=CARTESIAN_POINT ( 'NONE',  ( 39.37500000054622973, 26.92701409722686634, 93.04388485072563242 ) ) ;
#768=CARTESIAN_POINT ( 'NONE',  ( 21.55000000109246017, 22.43689772174679575, 98.29316153445363113 ) ) ;
#774=AXIS2_PLACEMENT_3D ( 'NONE', #1994, #5875, #10884 ) ;
#777=( BOUNDED_CURVE ( )  B_SPLINE_CURVE ( 2, ( #7759, #3949, #2936, #6801, #10668, #1977, #6866, #10730, #2042, #8250, #5333 ),
 .UNSPECIFIED., .F., .F. ) 
 B_SPLINE_CURVE_WITH_KNOTS ( ( 3, 2, 2, 2, 2, 3 ),
 ( 0.2999999999999999889, 0.3066666666666666430, 0.3133333333333333526, 0.3200000000000000622, 0.3266666666666667163, 0.3333333333333333703 ),
 .UNSPECIFIED. ) 
 CURVE ( )  GEOMETRIC_REPRESENTATION_ITEM ( )  RATIONAL_B_SPLINE_CURVE ( ( 1.000000000000000000, 0.9510565162951535312, 1.000000000000000000, 0.9510565162951535312, 1.000000000000000000, 0.9510565162951535312, 1.000000000000000000, 0.9510565162951535312, 1.000000000000000000, 0.9510565162951530871, 1.000000000000000444 ) ) 
 REPRESENTATION_ITEM ( '' )  );
#779=CARTESIAN_POINT ( 'NONE',  ( 42.57500000054622546, 13.80429023900056684, 86.29171490190961435 ) ) ;
#781=CARTESIAN_POINT ( 'NONE',  ( 45.67500000054621978, 24.28113015263587116, 96.68563167572563088 ) ) ;
#782=CARTESIAN_POINT ( 'NONE',  ( 47.79999999999999005, 24.40838939219354842, 96.86078899226572503 ) ) ;
#784=CARTESIAN_POINT ( 'NONE',  ( 39.45000000109246230, 24.40838939219354842, 96.86078899226572503 ) ) ;
#787=CARTESIAN_POINT ( 'NONE',  ( 37.95000000109246940, 13.62011893735971135, 95.42841645007781892 ) ) ;
#788=LINE ( 'NONE', #11445, #53 ) ;
#790=CARTESIAN_POINT ( 'NONE',  ( 49.99999999999998579, 0.000000000000000000, 69.99999999999998579 ) ) ;
#793=CARTESIAN_POINT ( 'NONE',  ( -2.000000000000015543, 20.00000000000000355, 90.79316153445363113 ) ) ;
#799=LINE ( 'NONE', #9557, #1526 ) ;
#800=DIRECTION ( 'NONE',  ( 1.000000000000000000, 0.000000000000000000, 0.000000000000000000 ) ) ;
#802=CARTESIAN_POINT ( 'NONE',  ( -50.00000000000001421, 18.00000000000000355, 188.4007504869563263 ) ) ;
#803=FACE_OUTER_BOUND ( 'NONE', #8940, .T. ) ;
#804=CARTESIAN_POINT ( 'NONE',  ( 48.37500000054621552, 12.34168156654572535, 90.79316153445363113 ) ) ;
#805=LINE ( 'NONE', #4675, #5389 ) ;
#811=CARTESIAN_POINT ( 'NONE',  ( 19.77500000054622831, 20.00000000000000355, 98.07665518445361386 ) ) ;
#813=LINE ( 'NONE', #7161, #2327 ) ;
#816=LINE ( 'NONE', #11223, #3260 ) ;
#821=CARTESIAN_POINT ( 'NONE',  ( 24.27500000054622475, 13.07298590277314254, 93.04388485072563242 ) ) ;
#823=CARTESIAN_POINT ( 'NONE',  ( 36.77500000054622831, 20.00000000000000355, 83.50966788445364841 ) ) ;
#824=CARTESIAN_POINT ( 'NONE',  ( 29.67500000054622333, 24.28113015263587116, 96.68563167572563088 ) ) ;
#825=CARTESIAN_POINT ( 'NONE',  ( 31.49999999999998224, 27.88596668178699645, 90.79316153445363113 ) ) ;
#827=CARTESIAN_POINT ( 'NONE',  ( 30.79999999999998650, 15.59161060780646046, 84.72553407664153724 ) ) ;
#828=CARTESIAN_POINT ( 'NONE',  ( 38.77500000054622831, 20.00000000000000355, 83.50966788445364841 ) ) ;
#830=CARTESIAN_POINT ( 'NONE',  ( 48.87500000054622262, 22.36655054427230382, 83.50966788445364841 ) ) ;
#831=DIRECTION ( 'NONE',  ( -1.000000000000000000, 0.000000000000000000, 0.000000000000000000 ) ) ;
#832=ORIENTED_EDGE ( 'NONE', *, *, #8899, .T. ) ;
#837=CARTESIAN_POINT ( 'NONE',  ( 42.05000000109246372, 12.86707612778636012, 93.11078899226572503 ) ) ;
#840=CARTESIAN_POINT ( 'NONE',  ( 42.07500000054622546, 15.71886984736413417, 96.68563167572563088 ) ) ;
#841=FACE_OUTER_BOUND ( 'NONE', #8965, .T. ) ;
#843=CARTESIAN_POINT ( 'NONE',  ( 44.67500000054621978, 15.71886984736413773, 84.90069139318163138 ) ) ;
#844=CARTESIAN_POINT ( 'NONE',  ( 20.07500000054622546, 15.71886984736413417, 96.68563167572563088 ) ) ;
#848=CARTESIAN_POINT ( 'NONE',  ( 34.85000000109246798, 24.40838939219355197, 84.72553407664153724 ) ) ;
#852=VERTEX_POINT ( 'NONE', #5027 ) ;
#853=DIRECTION ( 'NONE',  ( -1.000000000000000000, -0.000000000000000000, -0.000000000000000000 ) ) ;
#854=EDGE_CURVE ( 'NONE', #10832, #3939, #5915, .T. ) ;
#857=ADVANCED_FACE ( 'NONE', ( #1095 ), #4961, .F. ) ;
#862=CARTESIAN_POINT ( 'NONE',  ( 48.05000000109247082, 12.86707612778636012, 93.11078899226572503 ) ) ;
#863=CARTESIAN_POINT ( 'NONE',  ( 49.77500000054621410, 22.36655054427230027, 98.07665518445361386 ) ) ;
#865=LINE ( 'NONE', #4866, #9443 ) ;
#867=ORIENTED_EDGE ( 'NONE', *, *, #4196, .T. ) ;
#876=AXIS2_PLACEMENT_3D ( 'NONE', #7275, #9190, #4239 ) ;
#879=EDGE_CURVE ( 'NONE', #7138, #8662, #3257, .T. ) ;
#880=CARTESIAN_POINT ( 'NONE',  ( -21.00000000000001066, 77.00000000000000000, 154.3533255156881978 ) ) ;
#881=DIRECTION ( 'NONE',  ( 1.000000000000000000, 0.000000000000000000, 0.000000000000000000 ) ) ;
#883=CARTESIAN_POINT ( 'NONE',  ( 19.71250000081934672, 20.00000000000000355, 98.18490835945361539 ) ) ;
#886=VECTOR ( 'NONE', #11565, 1000.000000000000000 ) ;
#887=CARTESIAN_POINT ( 'NONE',  ( 26.77500000054622120, 17.63344945572770328, 83.50966788445364841 ) ) ;
#889=CARTESIAN_POINT ( 'NONE',  ( 42.17500000054622689, 13.07298590277314254, 93.04388485072563242 ) ) ;
#890=CARTESIAN_POINT ( 'NONE',  ( 24.77500000054622475, 17.63344945572770328, 83.50966788445364841 ) ) ;
#891=CARTESIAN_POINT ( 'NONE',  ( 32.09999999999998721, 17.56310227825320425, 98.29316153445363113 ) ) ;
#893=CARTESIAN_POINT ( 'NONE',  ( 34.69999999999998863, 13.62011893735970958, 86.15790661882942914 ) ) ;
#894=CARTESIAN_POINT ( 'NONE',  ( 34.07500000054622546, 13.80429023900056507, 95.29460816699764791 ) ) ;
#896=CARTESIAN_POINT ( 'NONE',  ( 42.37500000054622262, 13.07298590277314432, 88.54243821818161564 ) ) ;
#897=CARTESIAN_POINT ( 'NONE',  ( 28.05000000109246372, 12.86707612778636012, 93.11078899226572503 ) ) ;
#903=CARTESIAN_POINT ( 'NONE',  ( 32.69999999999999574, 13.62011893735970958, 86.15790661882942914 ) ) ;
#906=CARTESIAN_POINT ( 'NONE',  ( 46.47500000054622404, 13.07298590277314432, 88.54243821818161564 ) ) ;
#908=EDGE_CURVE ( 'NONE', #10212, #10832, #6331, .T. ) ;
#910=CARTESIAN_POINT ( 'NONE',  ( 46.47500000054622404, 13.07298590277314432, 88.54243821818161564 ) ) ;
#911=CARTESIAN_POINT ( 'NONE',  ( 46.79999999999999005, 15.59161060780646046, 84.72553407664153724 ) ) ;
#912=AXIS2_PLACEMENT_3D ( 'NONE', #4671, #10433, #1744 ) ;
#913=CARTESIAN_POINT ( 'NONE',  ( 41.99999999999998579, 20.00000000000000355, 98.29316153445363113 ) ) ;
#914=CARTESIAN_POINT ( 'NONE',  ( 49.67500000054621978, 22.36655054427230027, 98.07665518445361386 ) ) ;
#915=ORIENTED_EDGE ( 'NONE', *, *, #1713, .F. ) ;
#916=CARTESIAN_POINT ( 'NONE',  ( 38.25000000109246656, 12.86707612778636012, 88.47553407664152303 ) ) ;
#926=CARTESIAN_POINT ( 'NONE',  ( 37.87500000054622262, 17.63344945572769973, 98.07665518445361386 ) ) ;
#928=LINE ( 'NONE', #8541, #7268 ) ;
#931=LINE ( 'NONE', #802, #8606 ) ;
#933=CARTESIAN_POINT ( 'NONE',  ( 21.17500000054623044, 26.92701409722686634, 88.54243821818162985 ) ) ;
#935=CARTESIAN_POINT ( 'NONE',  ( -31.89339828220177964, 27.49999999999999645, 140.6066017177982133 ) ) ;
#939=EDGE_CURVE ( 'NONE', #7259, #10526, #4687, .T. ) ;
#940=VECTOR ( 'NONE', #3877, 1000.000000000000000 ) ;
#943=CARTESIAN_POINT ( 'NONE',  ( 20.99999999999998579, 20.00000000000000355, 83.29316153445364534 ) ) ;
#947=AXIS2_PLACEMENT_3D ( 'NONE', #5391, #1577, #1335 ) ;
#949=VERTEX_POINT ( 'NONE', #12428 ) ;
#952=EDGE_CURVE ( 'NONE', #3847, #6680, #3726, .T. ) ;
#955=CARTESIAN_POINT ( 'NONE',  ( 24.97500000054622049, 22.36655054427230382, 83.50966788445364841 ) ) ;
#956=CARTESIAN_POINT ( 'NONE',  ( 47.67500000054622689, 24.28113015263587116, 96.68563167572563088 ) ) ;
#957=CARTESIAN_POINT ( 'NONE',  ( 41.97500000054623115, 15.71886984736413417, 96.68563167572563088 ) ) ;
#959=CARTESIAN_POINT ( 'NONE',  ( 29.77500000054622120, 22.36655054427230027, 98.07665518445361386 ) ) ;
#960=CARTESIAN_POINT ( 'NONE',  ( 27.59999999999999076, 27.13292387221364876, 93.11078899226573924 ) ) ;
#961=CARTESIAN_POINT ( 'NONE',  ( 34.49999999999998579, 12.11403331821300533, 90.79316153445363113 ) ) ;
#962=CARTESIAN_POINT ( 'NONE',  ( 31.97500000054623470, 15.71886984736413417, 96.68563167572563088 ) ) ;
#964=LINE ( 'NONE', #12503, #10330 ) ;
#965=VECTOR ( 'NONE', #5995, 1000.000000000000000 ) ;
#969=CARTESIAN_POINT ( 'NONE',  ( 43.79999999999999005, 24.40838939219354842, 96.86078899226572503 ) ) ;
#972=CARTESIAN_POINT ( 'NONE',  ( 47.47500000054622404, 26.92701409722686634, 93.04388485072563242 ) ) ;
#973=DIRECTION ( 'NONE',  ( 0.000000000000000000, 0.000000000000000000, -1.000000000000000000 ) ) ;
#975=FACE_OUTER_BOUND ( 'NONE', #8889, .T. ) ;
#976=CARTESIAN_POINT ( 'NONE',  ( 43.77500000054622120, 22.36655054427230027, 98.07665518445361386 ) ) ;
#977=CARTESIAN_POINT ( 'NONE',  ( 21.37500000054622262, 27.65831843345427998, 90.79316153445363113 ) ) ;
#981=CARTESIAN_POINT ( 'NONE',  ( 28.95000000109246585, 26.37988106264029398, 86.15790661882942914 ) ) ;
#984=EDGE_LOOP ( 'NONE', ( #6494, #547, #3522, #403 ) ) ;
#990=CARTESIAN_POINT ( 'NONE',  ( 39.07500000054621836, 26.19570976099943493, 86.29171490190961435 ) ) ;
#991=CARTESIAN_POINT ( 'NONE',  ( 35.77500000054622831, 22.36655054427230027, 98.07665518445361386 ) ) ;
#994=CARTESIAN_POINT ( 'NONE',  ( 34.99999999999998579, 20.00000000000000000, 137.5000000000000000 ) ) ;
#997=LINE ( 'NONE', #6568, #10826 ) ;
#999=ORIENTED_EDGE ( 'NONE', *, *, #11054, .F. ) ;
#1003=ORIENTED_EDGE ( 'NONE', *, *, #6685, .F. ) ;
#1005=STYLED_ITEM('',(#12584),#6058);
#1007=CIRCLE ( 'NONE', #1208, 7.500000000000000000 ) ;
#1009=CARTESIAN_POINT ( 'NONE',  ( 43.55000000109247082, 22.43689772174677088, 98.29316153445365956 ) ) ;
#1011=CARTESIAN_POINT ( 'NONE',  ( -50.00000000000001421, 22.00000000000000000, 152.2284161474004520 ) ) ;
#1022=AXIS2_PLACEMENT_3D ( 'NONE', #1034, #7809, #4955 ) ;
#1024=CARTESIAN_POINT ( 'NONE',  ( 20.57500000054622191, 13.80429023900056684, 86.29171490190961435 ) ) ;
#1025=CARTESIAN_POINT ( 'NONE',  ( 49.37500000054622973, 27.65831843345427998, 90.79316153445363113 ) ) ;
#1026=CARTESIAN_POINT ( 'NONE',  ( 37.37500000054622973, 26.92701409722686634, 93.04388485072563242 ) ) ;
#1027=CARTESIAN_POINT ( 'NONE',  ( 27.77500000054622475, 22.36655054427230027, 98.07665518445361386 ) ) ;
#1028=CARTESIAN_POINT ( 'NONE',  ( 26.49999999999998934, 12.11403331821300533, 90.79316153445363113 ) ) ;
#1030=CARTESIAN_POINT ( 'NONE',  ( 32.87500000054622973, 22.36655054427230382, 83.50966788445364841 ) ) ;
#1034=CARTESIAN_POINT ( 'NONE',  ( -5.000000000000000888, -3.000000000000002665, 218.7511230907454944 ) ) ;
#1035=VERTEX_POINT ( 'NONE', #3161 ) ;
#1037=ORIENTED_EDGE ( 'NONE', *, *, #3690, .T. ) ;
#1039=CARTESIAN_POINT ( 'NONE',  ( -2.000000000000015543, 20.00000000000000355, 83.29316153445364534 ) ) ;
#1041=VECTOR ( 'NONE', #11538, 1000.000000000000000 ) ;
#1042=CARTESIAN_POINT ( 'NONE',  ( 46.17500000054622689, 13.80429023900056507, 95.29460816699764791 ) ) ;
#1043=FACE_OUTER_BOUND ( 'NONE', #6289, .T. ) ;
#1045=CARTESIAN_POINT ( 'NONE',  ( 46.87500000054622262, 20.00000000000000355, 83.50966788445364841 ) ) ;
#1046=CARTESIAN_POINT ( 'NONE',  ( 43.09999999999998721, 22.43689772174679575, 83.29316153445363113 ) ) ;
#1047=CARTESIAN_POINT ( 'NONE',  ( 39.99999999999998579, 20.00000000000000355, 98.29316153445363113 ) ) ;
#1048=CARTESIAN_POINT ( 'NONE',  ( 43.99999999999999289, 20.00000000000000355, 98.29316153445363113 ) ) ;
#1049=ORIENTED_EDGE ( 'NONE', *, *, #3891, .T. ) ;
#1050=CARTESIAN_POINT ( 'NONE',  ( 29.95000000109246585, 13.62011893735971135, 95.42841645007781892 ) ) ;
#1052=ORIENTED_EDGE ( 'NONE', *, *, #3804, .T. ) ;
#1053=ORIENTED_EDGE ( 'NONE', *, *, #1765, .F. ) ;
#1054=LINE ( 'NONE', #12403, #3624 ) ;
#1057=CARTESIAN_POINT ( 'NONE',  ( 39.47500000054623115, 26.19570976099943493, 95.29460816699764791 ) ) ;
#1058=CARTESIAN_POINT ( 'NONE',  ( 31.37500000054622618, 27.65831843345427998, 90.79316153445363113 ) ) ;
#1060=CARTESIAN_POINT ( 'NONE',  ( 33.79382810696422013, 25.37779564132841159, 151.2938281069642130 ) ) ;
#1063=ORIENTED_EDGE ( 'NONE', *, *, #1474, .F. ) ;
#1064=CARTESIAN_POINT ( 'NONE',  ( -50.00000000000001421, 22.00000000000000000, 169.9999999999999716 ) ) ;
#1069=CARTESIAN_POINT ( 'NONE',  ( 7.054895033614133837, 27.09199502823383909, 88.30591582403000928 ) ) ;
#1073=( BOUNDED_SURFACE ( )  B_SPLINE_SURFACE ( 1, 2, ( 
 ( #236, #3902, #1190, #5055, #11837, #9940, #1248, #7780, #6822, #7905, #1997, #11711, #4093, #7014, #2197, #5119, #8984, #10748, #9750, #8851, #5939, #4159, #4029, #11774, #3079, #7197, #7135, #1313, #542, #8160, #1492, #2264, #11073, #7260, #1559, #9301, #11009, #361, #8346, #10128, #5369, #4405, #9114, #2440, #5242, #4467, #3392, #421, #2323, #12027, #11134, #3331, #6317, #3514, #2503, #10185, #6131, #5182, #5429, #2379, #6377, #4283, #1375, #6189, #6250, #5307, #8222, #11964, #10244, #10064, #1438, #3274, #9175, #9050, #606, #12212, #8283, #483, #7323, #4349, #3459, #12090, #9239, #7386, #12152, #4227, #10002, #8099, #3760, #5495, #12397, #11505, #3697, #6614, #7577, #2562, #1735, #9364, #4595, #2814, #5740, #1616, #6678, #8588, #3635, #665, #10547, #9550, #9487, #9608, #4531, #2691, #11383, #5614, #916, #12458, #12337, #787, #8466, #6434, #2754, #7513, #8406, #4784, #8649, #11321, #7640, #6495, #11255, #8525, #5555, #4656, #6555, #10298, #12521, #3826, #1858, #1795, #12278, #3575, #7450, #2628, #10359, #1673, #11444, #9425, #10484, #726, #848, #10422, #5680, #4717, #10671, #6928, #11569, #10604, #11758, #1980, #7763, #4911, #155, #8772, #4012, #8966, #7954, #3066, #7701, #6741, #6995, #3954, #4076, #9734, #6805, #11636, #7828, #10733, #1108, #4847, #11820, #25, #91, #8713, #5864, #1917, #3128, #2178, #9861, #3888, #220, #6870, #8902, #11696, #4974, #9923, #7889, #5800, #1232, #1050, #10866, #9672, #8836, #6050, #10797, #2110, #5987, #2877, #2045, #981, #3002, #5101, #280, #2940, #5925, #5037, #9797, #1175, #3443, #2423, #2365, #2483, #9984, #8144, #4268, #11058, #11180, #5350, #5227, #7181, #1360, #11888, #8206, #9097, #1294, #6360, #10227, #4209, #1477, #11950, #4143, #1421, #10995, #6236, #405, #8017, #1540, #5413, #528, #7245, #5167, #9222, #3194, #4388, #8266, #9034, #9160, #7055, #465, #9284, #6300, #10933, #12135, #2247, #7121, #3375, #6114, #346, #12074, #10050, #11117, #8082, #12010, #4328, #7307, #3254, #2305, #6174, #3314, #10110, #10170, #5289, #7433, #768, #3560, #2796, #1718, #10282, #12383, #9347, #11304, #10405, #3617, #4578, #4513, #3742, #4637, #4700, #1659, #6418, #11428, #9407, #8572 ),
 ( #2610, #7497, #10342, #11486, #8449, #5540, #1599, #8508, #6479, #830, #12318, #10528, #3681, #9532, #6596, #5598, #650, #7369, #12443, #710, #10464, #5480, #8389, #11367, #2674, #6537, #9470, #12258, #7559, #2739, #1775, #5659, #7623, #6659, #3497, #1840, #5722, #587, #4453, #8331, #12197, #11238, #2546, #4177, #313, #8632, #7859, #5072, #10020, #1141, #11855, #251, #4107, #9001, #3162, #11788, #1329, #2143, #9589, #11919, #1263, #8938, #9829, #3093, #10763, #123, #9957, #6145, #6019, #7027, #5134, #7088, #8053, #3227, #896, #7987, #10969, #2277, #4767, #3982, #10901, #2216, #11730, #3033, #6086, #6898, #2074, #5954, #5005, #8870, #9892, #186, #4045, #7922, #6961, #10830, #10615, #9743, #3961, #12234, #10381, #1636, #7473, #1057, #2586, #9681, #8781, #990, #3896, #4856, #3537, #11579, #6458, #1866, #101, #3010, #11279, #7837, #5871, #926, #10319, #11706, #6816, #6750, #6878, #5516, #12529, #8659, #2887, #10742, #4919, #9619, #1927, #5748, #7410, #34, #4794, #9384, #2053, #5933, #8427, #9806, #3597, #8365, #5808, #2653, #8721, #3837, #686, #1117, #4553, #12297, #11644, #11347, #6516, #7711, #7773, #2951, #10679, #1990, #8844, #9993, #10122, #7129, #2375, #415, #6244, #7961, #4220, #164, #7897, #9045, #10878, #8092, #4983, #1241, #1306, #4276, #12020, #9870, #3073, #11068, #290, #11958, #11003, #11829, #5176, #3137, #7191, #6125, #7008, #5049, #2189, #356, #6060, #3267, #4022, #5236, #2315, #11767, #6936, #8154, #5112, #1370, #9933, #4086, #8910, #8976, #8028, #10943, #2120, #9108, #1183, #4153, #5997, #11899, #10804, #3324, #229, #6184, #3204, #10059, #7066, #2256, #11190, #7379, #3630, #6430, #4342, #7507, #12146, #10178, #4400, #11249, #4462, #5424, #5362, #4588, #5490, #5550, #2496, #7254, #12271, #10238, #9419, #8461, #1486, #2684, #12330, #9359, #11128, #6490, #476, #10353, #11315, #2434, #10292, #5300, #1610, #6549, #3569, #11379, #721, #1433, #8277, #659, #9169, #8216, #4524, #7318, #8400, #12085, #1551, #7445, #3387, #6312, #9233, #537, #3454, #9295, #2622, #1668, #6371, #600, #8341, #12207, #2556, #3508, #5315, #12099, #7330, #7269, #11201, #3584, #2571, #10250, #2330, #1382, #1622, #6323, #11265 ) ),
 .UNSPECIFIED., .F., .F., .F. ) 
 B_SPLINE_SURFACE_WITH_KNOTS ( ( 2, 2 ),
 ( 3, 2, 2, 2, 2, 2, 2, 2, 2, 2, 2, 2, 2, 2, 2, 2, 2, 2, 2, 2, 2, 2, 2, 2, 2, 2, 2, 2, 2, 2, 2, 2, 2, 2, 2, 2, 2, 2, 2, 2, 2, 2, 2, 2, 2, 2, 2, 2, 2, 2, 2, 2, 2, 2, 2, 2, 2, 2, 2, 2, 2, 2, 2, 2, 2, 2, 2, 2, 2, 2, 2, 2, 2, 2, 2, 2, 2, 2, 2, 2, 2, 2, 2, 2, 2, 2, 2, 2, 2, 2, 2, 2, 2, 2, 2, 2, 2, 2, 2, 2, 2, 2, 2, 2, 2, 2, 2, 2, 2, 2, 2, 2, 2, 2, 2, 2, 2, 2, 2, 2, 2, 2, 2, 2, 2, 2, 2, 2, 2, 2, 2, 2, 2, 2, 2, 2, 2, 2, 2, 2, 2, 2, 2, 2, 2, 2, 2, 2, 2, 2, 3 ),
 ( 0.000000000000000000, 1.000000000000000000 ),
 ( 0.000000000000000000, 0.006666666666666667095, 0.01333333333333333419, 0.02000000000000000042, 0.02666666666666666838, 0.03333333333333333287, 0.04000000000000000083, 0.04666666666666666879, 0.05333333333333333676, 0.05999999999999999778, 0.06666666666666666574, 0.07333333333333333370, 0.08000000000000000167, 0.08666666666666666963, 0.09333333333333333759, 0.1000000000000000056, 0.1066666666666666735, 0.1133333333333333276, 0.1199999999999999956, 0.1266666666666666774, 0.1333333333333333315, 0.1400000000000000133, 0.1466666666666666674, 0.1533333333333333215, 0.1600000000000000033, 0.1666666666666666574, 0.1733333333333333393, 0.1799999999999999933, 0.1866666666666666752, 0.1933333333333333293, 0.2000000000000000111, 0.2066666666666666652, 0.2133333333333333470, 0.2200000000000000011, 0.2266666666666666552, 0.2333333333333333370, 0.2399999999999999911, 0.2466666666666666730, 0.2533333333333333548, 0.2600000000000000089, 0.2666666666666666630, 0.2733333333333333171, 0.2800000000000000266, 0.2866666666666666807, 0.2933333333333333348, 0.2999999999999999889, 0.3066666666666666430, 0.3133333333333333526, 0.3200000000000000067, 0.3266666666666666607, 0.3333333333333333148, 0.3400000000000000244, 0.3466666666666666785, 0.3533333333333333326, 0.3599999999999999867, 0.3666666666666666408, 0.3733333333333333504, 0.3800000000000000044, 0.3866666666666666585, 0.3933333333333333126, 0.4000000000000000222, 0.4066666666666666763, 0.4133333333333333304, 0.4199999999999999845, 0.4266666666666666941, 0.4333333333333333481, 0.4400000000000000022, 0.4466666666666666563, 0.4533333333333333104, 0.4600000000000000200, 0.4666666666666666741, 0.4733333333333333282, 0.4799999999999999822, 0.4866666666666666918, 0.4933333333333333459, 0.5000000000000000000, 0.5066666666666667096, 0.5133333333333333082, 0.5200000000000000178, 0.5266666666666666163, 0.5333333333333333259, 0.5400000000000000355, 0.5466666666666666341, 0.5533333333333333437, 0.5600000000000000533, 0.5666666666666666519, 0.5733333333333333615, 0.5799999999999999600, 0.5866666666666666696, 0.5933333333333333792, 0.5999999999999999778, 0.6066666666666666874, 0.6133333333333332860, 0.6199999999999999956, 0.6266666666666667052, 0.6333333333333333037, 0.6400000000000000133, 0.6466666666666666119, 0.6533333333333333215, 0.6600000000000000311, 0.6666666666666666297, 0.6733333333333333393, 0.6800000000000000488, 0.6866666666666666474, 0.6933333333333333570, 0.6999999999999999556, 0.7066666666666666652, 0.7133333333333333748, 0.7199999999999999734, 0.7266666666666666829, 0.7333333333333332815, 0.7399999999999999911, 0.7466666666666667007, 0.7533333333333332993, 0.7600000000000000089, 0.7666666666666667185, 0.7733333333333333171, 0.7800000000000000266, 0.7866666666666666252, 0.7933333333333333348, 0.8000000000000000444, 0.8066666666666666430, 0.8133333333333333526, 0.8199999999999999512, 0.8266666666666666607, 0.8333333333333333703, 0.8399999999999999689, 0.8466666666666666785, 0.8533333333333333881, 0.8599999999999999867, 0.8666666666666666963, 0.8733333333333332948, 0.8800000000000000044, 0.8866666666666667140, 0.8933333333333333126, 0.9000000000000000222, 0.9066666666666666208, 0.9133333333333333304, 0.9200000000000000400, 0.9266666666666666385, 0.9333333333333333481, 0.9399999999999999467, 0.9466666666666666563, 0.9533333333333333659, 0.9599999999999999645, 0.9666666666666666741, 0.9733333333333333837, 0.9799999999999999822, 0.9866666666666666918, 0.9933333333333332904, 1.000000000000000000 ),
 .UNSPECIFIED. ) 
 GEOMETRIC_REPRESENTATION_ITEM ( )  RATIONAL_B_SPLINE_SURFACE ( (
 ( 1.000000000000000000, 0.9510565162951535312, 1.000000000000000000, 0.9510565162951535312, 1.000000000000000000, 0.9510565162951535312, 1.000000000000000000, 0.9510565162951535312, 1.000000000000000000, 0.9510565162951535312, 1.000000000000000000, 0.9510565162951535312, 1.000000000000000000, 0.9510565162951535312, 1.000000000000000000, 0.9510565162951535312, 1.000000000000000000, 0.9510565162951535312, 1.000000000000000000, 0.9510565162951535312, 1.000000000000000000, 0.9510565162951535312, 1.000000000000000000, 0.9510565162951535312, 1.000000000000000000, 0.9510565162951535312, 1.000000000000000000, 0.9510565162951535312, 1.000000000000000000, 0.9510565162951535312, 1.000000000000000000, 0.9510565162951535312, 1.000000000000000000, 0.9510565162951535312, 1.000000000000000000, 0.9510565162951535312, 1.000000000000000000, 0.9510565162951535312, 1.000000000000000000, 0.9510565162951535312, 1.000000000000000000, 0.9510565162951535312, 1.000000000000000000, 0.9510565162951535312, 1.000000000000000000, 0.9510565162951535312, 1.000000000000000000, 0.9510565162951535312, 1.000000000000000000, 0.9510565162951535312, 1.000000000000000000, 0.9510565162951535312, 1.000000000000000000, 0.9510565162951535312, 1.000000000000000000, 0.9510565162951535312, 1.000000000000000000, 0.9510565162951535312, 1.000000000000000000, 0.9510565162951535312, 1.000000000000000000, 0.9510565162951535312, 1.000000000000000000, 0.9510565162951535312, 1.000000000000000000, 0.9510565162951535312, 1.000000000000000000, 0.9510565162951535312, 1.000000000000000000, 0.9510565162951535312, 1.000000000000000000, 0.9510565162951535312, 1.000000000000000000, 0.9510565162951535312, 1.000000000000000000, 0.9510565162951535312, 1.000000000000000000, 0.9510565162951535312, 1.000000000000000000, 0.9510565162951535312, 1.000000000000000000, 0.9510565162951535312, 1.000000000000000000, 0.9510565162951535312, 1.000000000000000000, 0.9510565162951535312, 1.000000000000000000, 0.9510565162951535312, 1.000000000000000000, 0.9510565162951535312, 1.000000000000000000, 0.9510565162951535312, 1.000000000000000000, 0.9510565162951535312, 1.000000000000000000, 0.9510565162951535312, 1.000000000000000000, 0.9510565162951535312, 1.000000000000000000, 0.9510565162951535312, 1.000000000000000000, 0.9510565162951535312, 1.000000000000000000, 0.9510565162951535312, 1.000000000000000000, 0.9510565162951535312, 1.000000000000000000, 0.9510565162951535312, 1.000000000000000000, 0.9510565162951535312, 1.000000000000000000, 0.9510565162951535312, 1.000000000000000000, 0.9510565162951535312, 1.000000000000000000, 0.9510565162951535312, 1.000000000000000000, 0.9510565162951535312, 1.000000000000000000, 0.9510565162951535312, 1.000000000000000000, 0.9510565162951535312, 1.000000000000000000, 0.9510565162951535312, 1.000000000000000000, 0.9510565162951535312, 1.000000000000000000, 0.9510565162951535312, 1.000000000000000000, 0.9510565162951535312, 1.000000000000000000, 0.9510565162951535312, 1.000000000000000000, 0.9510565162951535312, 1.000000000000000000, 0.9510565162951535312, 1.000000000000000000, 0.9510565162951535312, 1.000000000000000000, 0.9510565162951535312, 1.000000000000000000, 0.9510565162951535312, 1.000000000000000000, 0.9510565162951535312, 1.000000000000000000, 0.9510565162951535312, 1.000000000000000000, 0.9510565162951535312, 1.000000000000000000, 0.9510565162951535312, 1.000000000000000000, 0.9510565162951535312, 1.000000000000000000, 0.9510565162951535312, 1.000000000000000000, 0.9510565162951535312, 1.000000000000000000, 0.9510565162951535312, 1.000000000000000000, 0.9510565162951535312, 1.000000000000000000, 0.9510565162951535312, 1.000000000000000000, 0.9510565162951535312, 1.000000000000000000, 0.9510565162951535312, 1.000000000000000000, 0.9510565162951535312, 1.000000000000000000, 0.9510565162951535312, 1.000000000000000000, 0.9510565162951535312, 1.000000000000000000, 0.9510565162951535312, 1.000000000000000000, 0.9510565162951535312, 1.000000000000000000, 0.9510565162951535312, 1.000000000000000000, 0.9510565162951535312, 1.000000000000000000, 0.9510565162951535312, 1.000000000000000000, 0.9510565162951535312, 1.000000000000000000, 0.9510565162951535312, 1.000000000000000000, 0.9510565162951535312, 1.000000000000000000, 0.9510565162951535312, 1.000000000000000000, 0.9510565162951535312, 1.000000000000000000, 0.9510565162951535312, 1.000000000000000000, 0.9510565162951535312, 1.000000000000000000, 0.9510565162951535312, 1.000000000000000000, 0.9510565162951535312, 1.000000000000000000, 0.9510565162951535312, 1.000000000000000000, 0.9510565162951535312, 1.000000000000000000, 0.9510565162951535312, 1.000000000000000000, 0.9510565162951535312, 1.000000000000000000, 0.9510565162951535312, 1.000000000000000000, 0.9510565162951535312, 1.000000000000000000, 0.9510565162951535312, 1.000000000000000000, 0.9510565162951535312, 1.000000000000000000, 0.9510565162951535312, 1.000000000000000000, 0.9510565162951535312, 1.000000000000000000, 0.9510565162951535312, 1.000000000000000000, 0.9510565162951535312, 1.000000000000000000, 0.9510565162951535312, 1.000000000000000000, 0.9510565162951535312, 1.000000000000000000, 0.9510565162951535312, 1.000000000000000000, 0.9510565162951535312, 1.000000000000000000, 0.9510565162951535312, 1.000000000000000000, 0.9510565162951535312, 1.000000000000000000, 0.9510565162951535312, 1.000000000000000000, 0.9510565162951535312, 1.000000000000000000, 0.9510565162951535312, 1.000000000000000000, 0.9510565162951535312, 1.000000000000000000, 0.9510565162951535312, 1.000000000000000000, 0.9510565162951535312, 1.000000000000000000, 0.9510565162951535312, 1.000000000000000000, 0.9510565162951535312, 1.000000000000000000, 0.9510565162951535312, 1.000000000000000000, 0.9510565162951535312, 1.000000000000000000, 0.9510565162951535312, 1.000000000000000000, 0.9510565162951535312, 1.000000000000000000, 0.9510565162951535312, 1.000000000000000000, 0.9510565162951535312, 1.000000000000000000, 0.9510565162951535312, 1.000000000000000000, 0.9510565162951535312, 1.000000000000000000, 0.9510565162951535312, 1.000000000000000000, 0.9510565162951535312, 1.000000000000000000, 0.9510565162951535312, 1.000000000000000000, 0.9510565162951535312, 1.000000000000000000, 0.9510565162951535312, 1.000000000000000000, 0.9510565162951535312, 1.000000000000000000, 0.9510565162951535312, 1.000000000000000000, 0.9510565162951535312, 1.000000000000000000, 0.9510565162951535312, 1.000000000000000000, 0.9510565162951535312, 1.000000000000000000, 0.9510565162951535312, 1.000000000000000000, 0.9510565162951535312, 1.000000000000000000, 0.9510565162951535312, 1.000000000000000000, 0.9510565162951535312, 1.000000000000000000, 0.9510565162951535312, 1.000000000000000000, 0.9510565162951535312, 1.000000000000000000),
 ( 1.000000000000000000, 0.9510565162951535312, 1.000000000000000000, 0.9510565162951535312, 1.000000000000000000, 0.9510565162951535312, 1.000000000000000000, 0.9510565162951535312, 1.000000000000000000, 0.9510565162951535312, 1.000000000000000000, 0.9510565162951535312, 1.000000000000000000, 0.9510565162951535312, 1.000000000000000000, 0.9510565162951535312, 1.000000000000000000, 0.9510565162951535312, 1.000000000000000000, 0.9510565162951535312, 1.000000000000000000, 0.9510565162951535312, 1.000000000000000000, 0.9510565162951535312, 1.000000000000000000, 0.9510565162951535312, 1.000000000000000000, 0.9510565162951535312, 1.000000000000000000, 0.9510565162951535312, 1.000000000000000000, 0.9510565162951535312, 1.000000000000000000, 0.9510565162951535312, 1.000000000000000000, 0.9510565162951535312, 1.000000000000000000, 0.9510565162951535312, 1.000000000000000000, 0.9510565162951535312, 1.000000000000000000, 0.9510565162951535312, 1.000000000000000000, 0.9510565162951535312, 1.000000000000000000, 0.9510565162951535312, 1.000000000000000000, 0.9510565162951535312, 1.000000000000000000, 0.9510565162951535312, 1.000000000000000000, 0.9510565162951535312, 1.000000000000000000, 0.9510565162951535312, 1.000000000000000000, 0.9510565162951535312, 1.000000000000000000, 0.9510565162951535312, 1.000000000000000000, 0.9510565162951535312, 1.000000000000000000, 0.9510565162951535312, 1.000000000000000000, 0.9510565162951535312, 1.000000000000000000, 0.9510565162951535312, 1.000000000000000000, 0.9510565162951535312, 1.000000000000000000, 0.9510565162951535312, 1.000000000000000000, 0.9510565162951535312, 1.000000000000000000, 0.9510565162951535312, 1.000000000000000000, 0.9510565162951535312, 1.000000000000000000, 0.9510565162951535312, 1.000000000000000000, 0.9510565162951535312, 1.000000000000000000, 0.9510565162951535312, 1.000000000000000000, 0.9510565162951535312, 1.000000000000000000, 0.9510565162951535312, 1.000000000000000000, 0.9510565162951535312, 1.000000000000000000, 0.9510565162951535312, 1.000000000000000000, 0.9510565162951535312, 1.000000000000000000, 0.9510565162951535312, 1.000000000000000000, 0.9510565162951535312, 1.000000000000000000, 0.9510565162951535312, 1.000000000000000000, 0.9510565162951535312, 1.000000000000000000, 0.9510565162951535312, 1.000000000000000000, 0.9510565162951535312, 1.000000000000000000, 0.9510565162951535312, 1.000000000000000000, 0.9510565162951535312, 1.000000000000000000, 0.9510565162951535312, 1.000000000000000000, 0.9510565162951535312, 1.000000000000000000, 0.9510565162951535312, 1.000000000000000000, 0.9510565162951535312, 1.000000000000000000, 0.9510565162951535312, 1.000000000000000000, 0.9510565162951535312, 1.000000000000000000, 0.9510565162951535312, 1.000000000000000000, 0.9510565162951535312, 1.000000000000000000, 0.9510565162951535312, 1.000000000000000000, 0.9510565162951535312, 1.000000000000000000, 0.9510565162951535312, 1.000000000000000000, 0.9510565162951535312, 1.000000000000000000, 0.9510565162951535312, 1.000000000000000000, 0.9510565162951535312, 1.000000000000000000, 0.9510565162951535312, 1.000000000000000000, 0.9510565162951535312, 1.000000000000000000, 0.9510565162951535312, 1.000000000000000000, 0.9510565162951535312, 1.000000000000000000, 0.9510565162951535312, 1.000000000000000000, 0.9510565162951535312, 1.000000000000000000, 0.9510565162951535312, 1.000000000000000000, 0.9510565162951535312, 1.000000000000000000, 0.9510565162951535312, 1.000000000000000000, 0.9510565162951535312, 1.000000000000000000, 0.9510565162951535312, 1.000000000000000000, 0.9510565162951535312, 1.000000000000000000, 0.9510565162951535312, 1.000000000000000000, 0.9510565162951535312, 1.000000000000000000, 0.9510565162951535312, 1.000000000000000000, 0.9510565162951535312, 1.000000000000000000, 0.9510565162951535312, 1.000000000000000000, 0.9510565162951535312, 1.000000000000000000, 0.9510565162951535312, 1.000000000000000000, 0.9510565162951535312, 1.000000000000000000, 0.9510565162951535312, 1.000000000000000000, 0.9510565162951535312, 1.000000000000000000, 0.9510565162951535312, 1.000000000000000000, 0.9510565162951535312, 1.000000000000000000, 0.9510565162951535312, 1.000000000000000000, 0.9510565162951535312, 1.000000000000000000, 0.9510565162951535312, 1.000000000000000000, 0.9510565162951535312, 1.000000000000000000, 0.9510565162951535312, 1.000000000000000000, 0.9510565162951535312, 1.000000000000000000, 0.9510565162951535312, 1.000000000000000000, 0.9510565162951535312, 1.000000000000000000, 0.9510565162951535312, 1.000000000000000000, 0.9510565162951535312, 1.000000000000000000, 0.9510565162951535312, 1.000000000000000000, 0.9510565162951535312, 1.000000000000000000, 0.9510565162951535312, 1.000000000000000000, 0.9510565162951535312, 1.000000000000000000, 0.9510565162951535312, 1.000000000000000000, 0.9510565162951535312, 1.000000000000000000, 0.9510565162951535312, 1.000000000000000000, 0.9510565162951535312, 1.000000000000000000, 0.9510565162951535312, 1.000000000000000000, 0.9510565162951535312, 1.000000000000000000, 0.9510565162951535312, 1.000000000000000000, 0.9510565162951535312, 1.000000000000000000, 0.9510565162951535312, 1.000000000000000000, 0.9510565162951535312, 1.000000000000000000, 0.9510565162951535312, 1.000000000000000000, 0.9510565162951535312, 1.000000000000000000, 0.9510565162951535312, 1.000000000000000000, 0.9510565162951535312, 1.000000000000000000, 0.9510565162951535312, 1.000000000000000000, 0.9510565162951535312, 1.000000000000000000, 0.9510565162951535312, 1.000000000000000000, 0.9510565162951535312, 1.000000000000000000, 0.9510565162951535312, 1.000000000000000000, 0.9510565162951535312, 1.000000000000000000, 0.9510565162951535312, 1.000000000000000000, 0.9510565162951535312, 1.000000000000000000, 0.9510565162951535312, 1.000000000000000000, 0.9510565162951535312, 1.000000000000000000, 0.9510565162951535312, 1.000000000000000000, 0.9510565162951535312, 1.000000000000000000, 0.9510565162951535312, 1.000000000000000000, 0.9510565162951535312, 1.000000000000000000, 0.9510565162951535312, 1.000000000000000000, 0.9510565162951535312, 1.000000000000000000, 0.9510565162951535312, 1.000000000000000000, 0.9510565162951535312, 1.000000000000000000, 0.9510565162951535312, 1.000000000000000000, 0.9510565162951535312, 1.000000000000000000, 0.9510565162951535312, 1.000000000000000000, 0.9510565162951535312, 1.000000000000000000, 0.9510565162951535312, 1.000000000000000000, 0.9510565162951535312, 1.000000000000000000, 0.9510565162951535312, 1.000000000000000000, 0.9510565162951535312, 1.000000000000000000, 0.9510565162951535312, 1.000000000000000000, 0.9510565162951535312, 1.000000000000000000, 0.9510565162951535312, 1.000000000000000000, 0.9510565162951535312, 1.000000000000000000) ) ) 
 REPRESENTATION_ITEM ( '' )  SURFACE ( )  );
#1076=DIRECTION ( 'NONE',  ( 0.000000000000000000, 0.000000000000000000, -1.000000000000000000 ) ) ;
#1080=CARTESIAN_POINT ( 'NONE',  ( 46.39999999999999147, 12.86707612778636012, 93.11078899226572503 ) ) ;
#1081=CARTESIAN_POINT ( 'NONE',  ( 23.95000000109246585, 13.62011893735970958, 95.42841645007781892 ) ) ;
#1083=CARTESIAN_POINT ( 'NONE',  ( 31.47500000054623115, 26.19570976099943849, 95.29460816699764791 ) ) ;
#1085=CARTESIAN_POINT ( 'NONE',  ( 20.69999999999998508, 13.62011893735971135, 86.15790661882942914 ) ) ;
#1087=CARTESIAN_POINT ( 'NONE',  ( 30.07500000054622546, 13.80429023900056507, 95.29460816699764791 ) ) ;
#1088=VERTEX_POINT ( 'NONE', #6960 ) ;
#1089=EDGE_CURVE ( 'NONE', #6104, #315, #2142, .T. ) ;
#1093=ORIENTED_EDGE ( 'NONE', *, *, #3973, .F. ) ;
#1095=FACE_OUTER_BOUND ( 'NONE', #9405, .T. ) ;
#1098=CARTESIAN_POINT ( 'NONE',  ( 36.47500000054622404, 13.07298590277314432, 88.54243821818161564 ) ) ;
#1099=DIRECTION ( 'NONE',  ( 0.000000000000000000, -1.000000000000000000, -0.000000000000000000 ) ) ;
#1100=CARTESIAN_POINT ( 'NONE',  ( 19.75000000109246301, 17.56310227825320425, 98.29316153445363113 ) ) ;
#1101=CARTESIAN_POINT ( 'NONE',  ( 37.67500000054621978, 24.28113015263587116, 96.68563167572563088 ) ) ;
#1102=CARTESIAN_POINT ( 'NONE',  ( 43.29999999999999716, 26.37988106264029398, 86.15790661882942914 ) ) ;
#1103=CARTESIAN_POINT ( 'NONE',  ( 39.19999999999998153, 24.40838939219355197, 84.72553407664153724 ) ) ;
#1108=CARTESIAN_POINT ( 'NONE',  ( 32.05000000109247082, 12.86707612778636012, 93.11078899226572503 ) ) ;
#1110=EDGE_LOOP ( 'NONE', ( #11355, #6664, #6554, #8560 ) ) ;
#1115=AXIS2_PLACEMENT_3D ( 'NONE', #11557, #8638, #1781 ) ;
#1117=CARTESIAN_POINT ( 'NONE',  ( 34.87500000054623683, 22.36655054427230382, 83.50966788445364841 ) ) ;
#1118=CARTESIAN_POINT ( 'NONE',  ( 31.67500000054622333, 24.28113015263587116, 96.68563167572563088 ) ) ;
#1120=EDGE_CURVE ( 'NONE', #1690, #3559, #7466, .T. ) ;
#1124=CARTESIAN_POINT ( 'NONE',  ( 48.87500000054622262, 20.00000000000000355, 83.50966788445364841 ) ) ;
#1127=VERTEX_POINT ( 'NONE', #7402 ) ;
#1132=ORIENTED_EDGE ( 'NONE', *, *, #3887, .T. ) ;
#1134=EDGE_CURVE ( 'NONE', #2251, #8953, #680, .T. ) ;
#1135=DIRECTION ( 'NONE',  ( 0.000000000000000000, 1.000000000000000000, 0.000000000000000000 ) ) ;
#1136=CARTESIAN_POINT ( 'NONE',  ( 23.99529484836403626, 27.49999999999999645, 148.5047051516359318 ) ) ;
#1141=CARTESIAN_POINT ( 'NONE',  ( 44.87500000054623683, 22.36655054427230382, 83.50966788445364841 ) ) ;
#1146=ADVANCED_FACE ( 'NONE', ( #4546 ), #8482, .F. ) ;
#1148=CARTESIAN_POINT ( 'NONE',  ( 20.97500000054622049, 22.36655054427230382, 83.50966788445364841 ) ) ;
#1150=CARTESIAN_POINT ( 'NONE',  ( 32.27500000054622831, 12.34168156654572357, 90.79316153445363113 ) ) ;
#1151=( BOUNDED_CURVE ( )  B_SPLINE_CURVE ( 2, ( #11518, #9500, #4799, #3842, #1745, #739, #862, #2643, #2704, #10562, #9376 ),
 .UNSPECIFIED., .F., .F. ) 
 B_SPLINE_CURVE_WITH_KNOTS ( ( 3, 2, 2, 2, 2, 3 ),
 ( 0.03333333333333336063, 0.04000000000000003553, 0.04666666666666670349, 0.05333333333333337839, 0.06000000000000005329, 0.06666666666666672125 ),
 .UNSPECIFIED. ) 
 CURVE ( )  GEOMETRIC_REPRESENTATION_ITEM ( )  RATIONAL_B_SPLINE_CURVE ( ( 0.9999999999999998890, 0.9510565162951537532, 1.000000000000000000, 0.9510565162951535312, 1.000000000000000000, 0.9510565162951535312, 1.000000000000000000, 0.9510565162951535312, 1.000000000000000000, 0.9510565162951530871, 1.000000000000000444 ) ) 
 REPRESENTATION_ITEM ( '' )  );
#1153=CARTESIAN_POINT ( 'NONE',  ( 22.29999999999999005, 13.62011893735971135, 95.42841645007781892 ) ) ;
#1154=DIRECTION ( 'NONE',  ( 1.000000000000000000, -0.000000000000000000, -0.000000000000000000 ) ) ;
#1155=CARTESIAN_POINT ( 'NONE',  ( 36.27500000054623541, 12.34168156654572535, 90.79316153445363113 ) ) ;
#1160=CARTESIAN_POINT ( 'NONE',  ( 48.85000000109246088, 24.40838939219355197, 84.72553407664153724 ) ) ;
#1162=VECTOR ( 'NONE', #6011, 1000.000000000000000 ) ;
#1163=DIRECTION ( 'NONE',  ( 1.000000000000000000, -0.000000000000000000, 0.000000000000000000 ) ) ;
#1165=CARTESIAN_POINT ( 'NONE',  ( 36.17500000054622689, 13.80429023900056507, 95.29460816699764791 ) ) ;
#1166=CARTESIAN_POINT ( 'NONE',  ( 40.05000000109246372, 12.86707612778636012, 93.11078899226572503 ) ) ;
#1168=CARTESIAN_POINT ( 'NONE',  ( 49.37500000054622973, 26.92701409722686634, 93.04388485072563242 ) ) ;
#1169=CARTESIAN_POINT ( 'NONE',  ( 40.77500000054622831, 17.63344945572770328, 83.50966788445364841 ) ) ;
#1170=CARTESIAN_POINT ( 'NONE',  ( 41.19999999999998863, 24.40838939219355197, 84.72553407664153724 ) ) ;
#1175=CARTESIAN_POINT ( 'NONE',  ( 28.15000000109246159, 12.11403331821300533, 90.79316153445363113 ) ) ;
#1177=ORIENTED_EDGE ( 'NONE', *, *, #1850, .T. ) ;
#1179=CARTESIAN_POINT ( 'NONE',  ( 25.15000000109246159, 27.88596668178699645, 90.79316153445363113 ) ) ;
#1183=CARTESIAN_POINT ( 'NONE',  ( 28.57500000054622902, 15.71886984736413773, 84.90069139318163138 ) ) ;
#1184=CARTESIAN_POINT ( 'NONE',  ( 30.87500000054622618, 20.00000000000000355, 83.50966788445364841 ) ) ;
#1186=CYLINDRICAL_SURFACE ( 'NONE', #5029, 7.500000000000000000 ) ;
#1189=EDGE_CURVE ( 'NONE', #5465, #2989, #8238, .T. ) ;
#1190=CARTESIAN_POINT ( 'NONE',  ( 49.45000000109246940, 24.40838939219354842, 96.86078899226572503 ) ) ;
#1191=ORIENTED_EDGE ( 'NONE', *, *, #7359, .F. ) ;
#1192=ORIENTED_EDGE ( 'NONE', *, *, #9696, .T. ) ;
#1195=EDGE_CURVE ( 'NONE', #12457, #8906, #10198, .T. ) ;
#1197=VECTOR ( 'NONE', #6338, 1000.000000000000000 ) ;
#1200=CARTESIAN_POINT ( 'NONE',  ( 8.865759858943656369, 24.63049972072609961, 84.88850774032545132 ) ) ;
#1205=AXIS2_PLACEMENT_3D ( 'NONE', #8995, #2139, #308 ) ;
#1206=CARTESIAN_POINT ( 'NONE',  ( 20.27158385259951956, 18.00000000000000355, 152.2284161474004520 ) ) ;
#1207=EDGE_LOOP ( 'NONE', ( #11253, #4786, #1003, #11710 ) ) ;
#1208=AXIS2_PLACEMENT_3D ( 'NONE', #31, #11575, #11640 ) ;
#1212=CARTESIAN_POINT ( 'NONE',  ( 23.17500000054622333, 26.19570976099943849, 86.29171490190961435 ) ) ;
#1213=CARTESIAN_POINT ( 'NONE',  ( 49.87500000054622262, 20.00000000000000355, 98.07665518445361386 ) ) ;
#1214=CARTESIAN_POINT ( 'NONE',  ( 31.77500000054622831, 20.00000000000000355, 98.07665518445361386 ) ) ;
#1215=CARTESIAN_POINT ( 'NONE',  ( 23.47500000054622404, 26.92701409722686634, 93.04388485072563242 ) ) ;
#1216=CARTESIAN_POINT ( 'NONE',  ( 21.19999999999998508, 24.40838939219355197, 84.72553407664153724 ) ) ;
#1217=CARTESIAN_POINT ( 'NONE',  ( -2.000000000000015543, 20.00000000000000355, 90.79316153445363113 ) ) ;
#1218=CARTESIAN_POINT ( 'NONE',  ( 28.77500000054622831, 20.00000000000000355, 83.50966788445364841 ) ) ;
#1219=ORIENTED_EDGE ( 'NONE', *, *, #5683, .F. ) ;
#1220=CARTESIAN_POINT ( 'NONE',  ( 23.25000000109246656, 27.13292387221364876, 93.11078899226573924 ) ) ;
#1225=CARTESIAN_POINT ( 'NONE',  ( 35.47500000054622404, 26.92701409722686634, 93.04388485072563242 ) ) ;
#1227=CARTESIAN_POINT ( 'NONE',  ( 39.27500000054622831, 26.92701409722686634, 88.54243821818162985 ) ) ;
#1228=CARTESIAN_POINT ( 'NONE',  ( 41.29999999999999716, 26.37988106264029398, 86.15790661882942914 ) ) ;
#1230=CARTESIAN_POINT ( 'NONE',  ( 48.97500000054622404, 24.28113015263587471, 84.90069139318163138 ) ) ;
#1232=CARTESIAN_POINT ( 'NONE',  ( 30.05000000109246727, 12.86707612778636012, 93.11078899226572503 ) ) ;
#1237=VECTOR ( 'NONE', #4254, 1000.000000000000000 ) ;
#1240=LINE ( 'NONE', #4151, #2913 ) ;
#1241=CARTESIAN_POINT ( 'NONE',  ( 32.27500000054622831, 12.34168156654572535, 90.79316153445363113 ) ) ;
#1242=CARTESIAN_POINT ( 'NONE',  ( 28.87500000054622262, 20.00000000000000355, 83.50966788445364841 ) ) ;
#1243=CARTESIAN_POINT ( 'NONE',  ( 43.85000000109246798, 15.59161060780645691, 96.86078899226572503 ) ) ;
#1246=AXIS2_PLACEMENT_3D ( 'NONE', #11104, #3428, #2411 ) ;
#1247=CARTESIAN_POINT ( 'NONE',  ( 47.67500000054622689, 24.28113015263587116, 96.68563167572563088 ) ) ;
#1248=CARTESIAN_POINT ( 'NONE',  ( 49.05000000109246372, 27.13292387221364876, 88.47553407664153724 ) ) ;
#1249=CARTESIAN_POINT ( 'NONE',  ( -27.49999999999999645, 20.00000000000000355, 99.99999999999997158 ) ) ;
#1251=CARTESIAN_POINT ( 'NONE',  ( -36.00000000000000711, 81.39339828220178674, 154.3533255156881694 ) ) ;
#1252=ADVANCED_FACE ( 'NONE', ( #3777 ), #6759, .F. ) ;
#1255=DIRECTION ( 'NONE',  ( -0.000000000000000000, 0.000000000000000000, 1.000000000000000000 ) ) ;
#1257=CARTESIAN_POINT ( 'NONE',  ( 8.561724788085411930, 25.17060510151400976, 85.35530319090553064 ) ) ;
#1261=CARTESIAN_POINT ( 'NONE',  ( -50.00000000000001421, 92.00000000000000000, 166.8533255156881694 ) ) ;
#1262=EDGE_CURVE ( 'NONE', #8484, #223, #865, .T. ) ;
#1263=CARTESIAN_POINT ( 'NONE',  ( 43.77500000054622831, 20.00000000000000355, 98.07665518445361386 ) ) ;
#1268=( BOUNDED_CURVE ( )  B_SPLINE_CURVE ( 2, ( #6445, #1569, #3524, #11021, #5442, #9313, #11268, #9061, #8108, #11978, #9122 ),
 .UNSPECIFIED., .F., .F. ) 
 B_SPLINE_CURVE_WITH_KNOTS ( ( 3, 2, 2, 2, 2, 3 ),
 ( 0.3666666666666666963, 0.3733333333333334059, 0.3800000000000000600, 0.3866666666666667695, 0.3933333333333334236, 0.4000000000000001332 ),
 .UNSPECIFIED. ) 
 CURVE ( )  GEOMETRIC_REPRESENTATION_ITEM ( )  RATIONAL_B_SPLINE_CURVE ( ( 0.9999999999999995559, 0.9510565162951539753, 1.000000000000000000, 0.9510565162951535312, 1.000000000000000000, 0.9510565162951535312, 1.000000000000000000, 0.9510565162951535312, 1.000000000000000000, 0.9510565162951527540, 1.000000000000000888 ) ) 
 REPRESENTATION_ITEM ( '' )  );
#1269=EDGE_CURVE ( 'NONE', #11196, #1420, #9006, .T. ) ;
#1270=CARTESIAN_POINT ( 'NONE',  ( 20.17500000054622333, 13.80429023900056507, 95.29460816699764791 ) ) ;
#1271=CARTESIAN_POINT ( 'NONE',  ( 46.97500000054621694, 22.36655054427230382, 83.50966788445364841 ) ) ;
#1272=CARTESIAN_POINT ( 'NONE',  ( 33.57500000054623257, 24.28113015263587116, 96.68563167572563088 ) ) ;
#1273=CARTESIAN_POINT ( 'NONE',  ( 20.57500000054622546, 13.80429023900056684, 86.29171490190961435 ) ) ;
#1274=DIRECTION ( 'NONE',  ( 1.000000000000000000, -0.000000000000000000, -0.000000000000000000 ) ) ;
#1275=CARTESIAN_POINT ( 'NONE',  ( -111.8465843842649292, 77.00000000000000000, 94.35332551568819781 ) ) ;
#1276=CARTESIAN_POINT ( 'NONE',  ( 28.37500000054622618, 13.07298590277314432, 88.54243821818161564 ) ) ;
#1277=ORIENTED_EDGE ( 'NONE', *, *, #10927, .F. ) ;
#1278=CARTESIAN_POINT ( 'NONE',  ( 32.95000000109246230, 26.37988106264029398, 86.15790661882942914 ) ) ;
#1281=CARTESIAN_POINT ( 'NONE',  ( 49.93750000027311131, 20.00000000000000355, 98.18490835945361539 ) ) ;
#1282=ORIENTED_EDGE ( 'NONE', *, *, #4134, .T. ) ;
#1286=CARTESIAN_POINT ( 'NONE',  ( 40.17500000054622689, 13.80429023900056507, 95.29460816699764791 ) ) ;
#1288=CARTESIAN_POINT ( 'NONE',  ( 19.85000000109246443, 15.59161060780645691, 96.86078899226572503 ) ) ;
#1289=CARTESIAN_POINT ( 'NONE',  ( 40.87500000054622262, 20.00000000000000355, 83.50966788445364841 ) ) ;
#1290=CARTESIAN_POINT ( 'NONE',  ( 41.99999999999998579, 20.00000000000000355, 98.29316153445363113 ) ) ;
#1291=CARTESIAN_POINT ( 'NONE',  ( 44.47500000054622404, 13.80429023900056684, 86.29171490190961435 ) ) ;
#1294=CARTESIAN_POINT ( 'NONE',  ( 26.45000000109246585, 15.59161060780646046, 84.72553407664153724 ) ) ;
#1298=CARTESIAN_POINT ( 'NONE',  ( 26.37500000054622618, 12.34168156654572357, 90.79316153445363113 ) ) ;
#1301=CARTESIAN_POINT ( 'NONE',  ( 25.25000000109246301, 27.13292387221364876, 93.11078899226573924 ) ) ;
#1302=CARTESIAN_POINT ( 'NONE',  ( 41.35000000109245377, 26.37988106264029398, 95.42841645007781892 ) ) ;
#1304=CARTESIAN_POINT ( 'NONE',  ( 48.69999999999998153, 13.62011893735970958, 86.15790661882942914 ) ) ;
#1306=CARTESIAN_POINT ( 'NONE',  ( 32.17500000054622689, 13.07298590277314254, 93.04388485072563242 ) ) ;
#1307=CARTESIAN_POINT ( 'NONE',  ( 32.67500000054622689, 15.71886984736413773, 84.90069139318163138 ) ) ;
#1308=AXIS2_PLACEMENT_3D ( 'NONE', #4527, #11251, #10481 ) ;
#1309=CARTESIAN_POINT ( 'NONE',  ( -50.00000000000001421, 20.00000000000000000, 145.0000000000000000 ) ) ;
#1311=CARTESIAN_POINT ( 'NONE',  ( 22.25000000109246656, 12.86707612778636012, 88.47553407664152303 ) ) ;
#1312=ORIENTED_EDGE ( 'NONE', *, *, #12502, .F. ) ;
#1313=CARTESIAN_POINT ( 'NONE',  ( 46.95000000109246940, 26.37988106264029398, 86.15790661882942914 ) ) ;
#1315=ORIENTED_EDGE ( 'NONE', *, *, #5224, .F. ) ;
#1317=VERTEX_POINT ( 'NONE', #7783 ) ;
#1323=CARTESIAN_POINT ( 'NONE',  ( 22.79999999999998650, 15.59161060780646046, 84.72553407664153724 ) ) ;
#1325=LINE ( 'NONE', #4174, #9796 ) ;
#1329=CARTESIAN_POINT ( 'NONE',  ( 44.17500000054622689, 13.07298590277314254, 93.04388485072563242 ) ) ;
#1332=VERTEX_POINT ( 'NONE', #1064 ) ;
#1335=DIRECTION ( 'NONE',  ( -1.000000000000000000, 0.000000000000000000, 0.000000000000000000 ) ) ;
#1336=CARTESIAN_POINT ( 'NONE',  ( 46.57500000054623257, 13.80429023900056684, 86.29171490190961435 ) ) ;
#1337=CARTESIAN_POINT ( 'NONE',  ( 30.67500000054622689, 17.63344945572770328, 83.50966788445364841 ) ) ;
#1338=CARTESIAN_POINT ( 'NONE',  ( 20.27500000054622475, 13.07298590277314254, 93.04388485072563242 ) ) ;
#1339=CARTESIAN_POINT ( 'NONE',  ( -2.000000000000015543, 20.00000000000000355, 83.29316153445364534 ) ) ;
#1340=VECTOR ( 'NONE', #10577, 1000.000000000000000 ) ;
#1341=FACE_OUTER_BOUND ( 'NONE', #9704, .T. ) ;
#1342=CARTESIAN_POINT ( 'NONE',  ( 25.37500000054622973, 26.92701409722686634, 93.04388485072563242 ) ) ;
#1345=VECTOR ( 'NONE', #9054, 1000.000000000000114 ) ;
#1350=EDGE_LOOP ( 'NONE', ( #3303, #487, #9055, #3936, #12305, #464 ) ) ;
#1352=EDGE_CURVE ( 'NONE', #11822, #3847, #7629, .T. ) ;
#1353=CARTESIAN_POINT ( 'NONE',  ( 36.07500000054622546, 15.71886984736413417, 96.68563167572563088 ) ) ;
#1354=CARTESIAN_POINT ( 'NONE',  ( 36.89999999999999147, 17.56310227825322912, 83.29316153445363113 ) ) ;
#1355=CARTESIAN_POINT ( 'NONE',  ( -2.000000000000015543, 20.00000000000000355, 90.79316153445363113 ) ) ;
#1356=CARTESIAN_POINT ( 'NONE',  ( 40.37500000054621552, 12.34168156654572535, 90.79316153445363113 ) ) ;
#1357=CARTESIAN_POINT ( 'NONE',  ( 36.19999999999998863, 15.59161060780645691, 96.86078899226572503 ) ) ;
#1358=CARTESIAN_POINT ( 'NONE',  ( 44.17500000054622689, 13.07298590277314254, 93.04388485072563242 ) ) ;
#1360=CARTESIAN_POINT ( 'NONE',  ( 26.85000000109246443, 24.40838939219355197, 84.72553407664153724 ) ) ;
#1365=ORIENTED_EDGE ( 'NONE', *, *, #1416, .F. ) ;
#1370=CARTESIAN_POINT ( 'NONE',  ( 29.47500000054622404, 26.19570976099943493, 95.29460816699764791 ) ) ;
#1371=CARTESIAN_POINT ( 'NONE',  ( 25.77500000054622831, 22.36655054427230027, 98.07665518445361386 ) ) ;
#1374=ORIENTED_EDGE ( 'NONE', *, *, #12157, .T. ) ;
#1375=CARTESIAN_POINT ( 'NONE',  ( 43.45000000109246230, 24.40838939219354842, 96.86078899226572503 ) ) ;
#1378=ORIENTED_EDGE ( 'NONE', *, *, #7422, .T. ) ;
#1382=CARTESIAN_POINT ( 'NONE',  ( 20.07500000054622546, 13.80429023900056507, 95.29460816699764791 ) ) ;
#1385=CARTESIAN_POINT ( 'NONE',  ( 22.49999999999998934, 12.11403331821300533, 90.79316153445363113 ) ) ;
#1388=EDGE_CURVE ( 'NONE', #2031, #9944, #805, .T. ) ;
#1396=CARTESIAN_POINT ( 'NONE',  ( 25.99999999999998934, 20.00000000000000355, 98.29316153445363113 ) ) ;
#1397=CYLINDRICAL_SURFACE ( 'NONE', #947, 10.00000000000000355 ) ;
#1398=CARTESIAN_POINT ( 'NONE',  ( 42.97500000054622404, 22.36655054427230382, 83.50966788445364841 ) ) ;
#1399=EDGE_CURVE ( 'NONE', #11822, #707, #1556, .T. ) ;
#1400=CARTESIAN_POINT ( 'NONE',  ( 24.77500000054622831, 20.00000000000000355, 83.50966788445364841 ) ) ;
#1401=VECTOR ( 'NONE', #11784, 1000.000000000000000 ) ;
#1403=LINE ( 'NONE', #1339, #9996 ) ;
#1404=DIRECTION ( 'NONE',  ( 0.000000000000000000, 0.000000000000000000, 1.000000000000000000 ) ) ;
#1405=CARTESIAN_POINT ( 'NONE',  ( 31.99999999999998579, 20.00000000000000355, 98.29316153445363113 ) ) ;
#1406=CARTESIAN_POINT ( 'NONE',  ( 26.67500000054622689, 17.63344945572770328, 83.50966788445364841 ) ) ;
#1408=DIRECTION ( 'NONE',  ( 1.000000000000000000, -0.000000000000000000, -0.000000000000000000 ) ) ;
#1409=ORIENTED_EDGE ( 'NONE', *, *, #9208, .F. ) ;
#1410=CARTESIAN_POINT ( 'NONE',  ( 38.39999999999999147, 12.86707612778636012, 93.11078899226572503 ) ) ;
#1411=VERTEX_POINT ( 'NONE', #10067 ) ;
#1414=CARTESIAN_POINT ( 'NONE',  ( 33.67500000054622689, 24.28113015263587116, 96.68563167572563088 ) ) ;
#1416=EDGE_CURVE ( 'NONE', #5416, #3740, #10814, .T. ) ;
#1417=CARTESIAN_POINT ( 'NONE',  ( 43.37500000054622973, 26.92701409722686634, 93.04388485072563242 ) ) ;
#1418=CARTESIAN_POINT ( 'NONE',  ( 33.79999999999999005, 24.40838939219354842, 96.86078899226572503 ) ) ;
#1419=CARTESIAN_POINT ( 'NONE',  ( 45.27500000054622831, 27.65831843345427998, 90.79316153445363113 ) ) ;
#1420=VERTEX_POINT ( 'NONE', #10005 ) ;
#1421=CARTESIAN_POINT ( 'NONE',  ( 25.75000000109246301, 17.56310227825320425, 98.29316153445363113 ) ) ;
#1423=ORIENTED_EDGE ( 'NONE', *, *, #2963, .T. ) ;
#1424=EDGE_CURVE ( 'NONE', #8002, #7325, #4223, .T. ) ;
#1425=CARTESIAN_POINT ( 'NONE',  ( -2.000000000000015543, 20.00000000000000355, 90.79316153445363113 ) ) ;
#1428=CARTESIAN_POINT ( 'NONE',  ( 20.85000000109246443, 24.40838939219355197, 84.72553407664153724 ) ) ;
#1431=CARTESIAN_POINT ( 'NONE',  ( 24.99999999999998579, 20.00000000000000355, 83.29316153445364534 ) ) ;
#1433=CARTESIAN_POINT ( 'NONE',  ( 23.47500000054623115, 26.19570976099943493, 95.29460816699764791 ) ) ;
#1434=CARTESIAN_POINT ( 'NONE',  ( 25.07500000054622191, 24.28113015263587471, 84.90069139318163138 ) ) ;
#1436=CARTESIAN_POINT ( 'NONE',  ( 21.65000000109246514, 20.00000000000000355, 98.29316153445363113 ) ) ;
#1437=EDGE_LOOP ( 'NONE', ( #2533, #1177, #7690, #11506, #832, #5613, #11042, #9817, #1192 ) ) ;
#1438=CARTESIAN_POINT ( 'NONE',  ( 42.65000000109246514, 20.00000000000000355, 83.29316153445364534 ) ) ;
#1449=CARTESIAN_POINT ( 'NONE',  ( 22.29999999999998295, 13.62011893735970958, 95.42841645007781892 ) ) ;
#1451=LINE ( 'NONE', #10077, #8378 ) ;
#1452=CARTESIAN_POINT ( 'NONE',  ( 4.999999999999999112, -3.000000000000002665, 121.2488769092545198 ) ) ;
#1459=CARTESIAN_POINT ( 'NONE',  ( 49.71250000081935383, 20.00000000000000355, 98.18490835945361539 ) ) ;
#1460=CARTESIAN_POINT ( 'NONE',  ( 41.47500000054623115, 26.92701409722686634, 93.04388485072563242 ) ) ;
#1461=CARTESIAN_POINT ( 'NONE',  ( 24.07500000054622902, 13.80429023900056507, 95.29460816699764791 ) ) ;
#1462=CARTESIAN_POINT ( 'NONE',  ( 7.146477089513696868, 13.00393516148637651, 88.07960685825688074 ) ) ;
#1463=CARTESIAN_POINT ( 'NONE',  ( -50.00000000000001421, 0.000000000000000000, 69.99999999999998579 ) ) ;
#1464=CARTESIAN_POINT ( 'NONE',  ( -50.00000000000001421, 55.00000000000000000, 147.8533255156883399 ) ) ;
#1466=EDGE_LOOP ( 'NONE', ( #3319, #10629, #3956, #11590, #9721, #3647, #7782, #8853, #9846 ) ) ;
#1469=CARTESIAN_POINT ( 'NONE',  ( 32.27500000054622831, 13.07298590277314254, 93.04388485072563242 ) ) ;
#1470=DIRECTION ( 'NONE',  ( 1.000000000000000000, -0.000000000000000000, -0.000000000000000000 ) ) ;
#1471=CARTESIAN_POINT ( 'NONE',  ( 45.57500000054622546, 24.28113015263587116, 96.68563167572563088 ) ) ;
#1472=CARTESIAN_POINT ( 'NONE',  ( 32.17500000054621978, 13.80429023900056507, 95.29460816699764791 ) ) ;
#1473=CARTESIAN_POINT ( 'NONE',  ( 38.29999999999997584, 13.62011893735971135, 95.42841645007781892 ) ) ;
#1474=EDGE_CURVE ( 'NONE', #10, #3463, #8986, .T. ) ;
#1475=CARTESIAN_POINT ( 'NONE',  ( 45.87500000054622973, 17.63344945572769973, 98.07665518445361386 ) ) ;
#1476=ORIENTED_EDGE ( 'NONE', *, *, #1195, .T. ) ;
#1477=CARTESIAN_POINT ( 'NONE',  ( 26.05000000109246727, 12.86707612778636012, 93.11078899226572503 ) ) ;
#1481=ORIENTED_EDGE ( 'NONE', *, *, #5689, .T. ) ;
#1486=CARTESIAN_POINT ( 'NONE',  ( 25.17500000054623044, 26.92701409722686634, 88.54243821818162985 ) ) ;
#1487=CARTESIAN_POINT ( 'NONE',  ( 24.97500000054622049, 22.36655054427230382, 83.50966788445364841 ) ) ;
#1492=CARTESIAN_POINT ( 'NONE',  ( 46.65000000109246514, 20.00000000000000355, 83.29316153445364534 ) ) ;
#1494=ORIENTED_EDGE ( 'NONE', *, *, #7603, .F. ) ;
#1495=CARTESIAN_POINT ( 'NONE',  ( -20.27158385259951956, 18.00000000000000355, 170.0000119999999697 ) ) ;
#1508=DIRECTION ( 'NONE',  ( -0.000000000000000000, 1.000000000000000000, -0.000000000000000000 ) ) ;
#1510=CARTESIAN_POINT ( 'NONE',  ( 23.79999999999998650, 24.40838939219354842, 96.86078899226572503 ) ) ;
#1512=DIRECTION ( 'NONE',  ( 0.000000000000000000, 0.000000000000000000, -1.000000000000000000 ) ) ;
#1515=CARTESIAN_POINT ( 'NONE',  ( 42.27500000054622120, 13.07298590277314254, 93.04388485072563242 ) ) ;
#1516=CARTESIAN_POINT ( 'NONE',  ( 27.87500000054622618, 17.63344945572769973, 98.07665518445361386 ) ) ;
#1517=CARTESIAN_POINT ( 'NONE',  ( 9.480548647978427113, 16.81007977654359919, 84.00085956564031164 ) ) ;
#1518=DIRECTION ( 'NONE',  ( -0.7071067811865460184, -0.000000000000000000, 0.7071067811865490160 ) ) ;
#1522=DIRECTION ( 'NONE',  ( 0.000000000000000000, 0.000000000000000000, -1.000000000000000000 ) ) ;
#1525=FACE_OUTER_BOUND ( 'NONE', #6316, .T. ) ;
#1526=VECTOR ( 'NONE', #11390, 1000.000000000000000 ) ;
#1530=CARTESIAN_POINT ( 'NONE',  ( 34.27500000054622120, 13.07298590277314254, 93.04388485072563242 ) ) ;
#1533=CARTESIAN_POINT ( 'NONE',  ( 43.17500000054622689, 26.92701409722686634, 88.54243821818162985 ) ) ;
#1534=CARTESIAN_POINT ( 'NONE',  ( 36.17500000054623399, 13.80429023900056507, 95.29460816699764791 ) ) ;
#1535=CARTESIAN_POINT ( 'NONE',  ( 35.79999999999998295, 24.40838939219354842, 96.86078899226572503 ) ) ;
#1538=CARTESIAN_POINT ( 'NONE',  ( 42.37500000054622262, 13.07298590277314432, 88.54243821818161564 ) ) ;
#1539=ORIENTED_EDGE ( 'NONE', *, *, #7218, .F. ) ;
#1540=CARTESIAN_POINT ( 'NONE',  ( 25.25000000109246301, 27.13292387221364876, 93.11078899226573924 ) ) ;
#1545=CYLINDRICAL_SURFACE ( 'NONE', #2118, 7.499999999999992895 ) ;
#1546=DIRECTION ( 'NONE',  ( 0.000000000000000000, 0.000000000000000000, -1.000000000000000000 ) ) ;
#1547=ADVANCED_FACE ( 'NONE', ( #6007 ), #10954, .F. ) ;
#1548=AXIS2_PLACEMENT_3D ( 'NONE', #608, #10188, #9117 ) ;
#1549=DIRECTION ( 'NONE',  ( 1.000000000000000000, -0.000000000000000000, -0.000000000000000000 ) ) ;
#1550=CARTESIAN_POINT ( 'NONE',  ( 25.69999999999998153, 26.37988106264029398, 95.42841645007781892 ) ) ;
#1551=CARTESIAN_POINT ( 'NONE',  ( 22.57500000054622902, 15.71886984736413773, 84.90069139318163138 ) ) ;
#1552=CARTESIAN_POINT ( 'NONE',  ( 26.17500000054622689, 13.80429023900056507, 95.29460816699764791 ) ) ;
#1554=VECTOR ( 'NONE', #244, 1000.000000000000000 ) ;
#1556=( BOUNDED_CURVE ( )  B_SPLINE_CURVE ( 3, ( #9627, #935, #4993, #3145 ),
 .UNSPECIFIED., .F., .F. ) 
 B_SPLINE_CURVE_WITH_KNOTS ( ( 4, 4 ),
 ( 1.570796326794896558, 3.141592653589793560 ),
 .UNSPECIFIED. ) 
 CURVE ( )  GEOMETRIC_REPRESENTATION_ITEM ( )  RATIONAL_B_SPLINE_CURVE ( ( 1.000000000000000000, 0.8047378541243649375, 0.8047378541243649375, 1.000000000000000000 ) ) 
 REPRESENTATION_ITEM ( '' )  );
#1558=ORIENTED_EDGE ( 'NONE', *, *, #10326, .F. ) ;
#1559=CARTESIAN_POINT ( 'NONE',  ( 46.25000000109246656, 12.86707612778636012, 88.47553407664152303 ) ) ;
#1562=ORIENTED_EDGE ( 'NONE', *, *, #7766, .T. ) ;
#1567=CARTESIAN_POINT ( 'NONE',  ( 29.79999999999998650, 24.40838939219354842, 96.86078899226572503 ) ) ;
#1568=EDGE_CURVE ( 'NONE', #3396, #2741, #2022, .T. ) ;
#1569=CARTESIAN_POINT ( 'NONE',  ( 38.55000000109247082, 17.56310227825319359, 83.29316153445364534 ) ) ;
#1571=CARTESIAN_POINT ( 'NONE',  ( -50.00000000000001421, 20.00000000000000000, 145.0000000000000000 ) ) ;
#1573=CARTESIAN_POINT ( 'NONE',  ( 47.25000000109246656, 27.13292387221364876, 93.11078899226573924 ) ) ;
#1574=ORIENTED_EDGE ( 'NONE', *, *, #1120, .F. ) ;
#1576=CARTESIAN_POINT ( 'NONE',  ( -34.99999999999999289, 20.00000000000000355, 99.99999999999997158 ) ) ;
#1577=DIRECTION ( 'NONE',  ( 0.000000000000000000, 0.000000000000000000, -1.000000000000000000 ) ) ;
#1578=CARTESIAN_POINT ( 'NONE',  ( 40.27500000054622120, 13.07298590277314254, 93.04388485072563242 ) ) ;
#1579=CARTESIAN_POINT ( 'NONE',  ( 27.57500000054622902, 24.28113015263587116, 96.68563167572563088 ) ) ;
#1580=CARTESIAN_POINT ( 'NONE',  ( 6.688794870772565737, 12.56618450651110308, 89.76590532369878872 ) ) ;
#1585=VERTEX_POINT ( 'NONE', #3081 ) ;
#1590=CARTESIAN_POINT ( 'NONE',  ( 29.97500000054622404, 17.63344945572769973, 98.07665518445361386 ) ) ;
#1591=CARTESIAN_POINT ( 'NONE',  ( 27.55000000109246017, 22.43689772174679575, 98.29316153445363113 ) ) ;
#1592=CARTESIAN_POINT ( 'NONE',  ( 47.17500000054623399, 26.92701409722686634, 88.54243821818162985 ) ) ;
#1594=CARTESIAN_POINT ( 'NONE',  ( 31.87500000054622262, 20.00000000000000355, 98.07665518445361386 ) ) ;
#1595=CARTESIAN_POINT ( 'NONE',  ( 36.39999999999999147, 12.86707612778636012, 93.11078899226572503 ) ) ;
#1597=CARTESIAN_POINT ( 'NONE',  ( 38.37500000054622973, 13.07298590277314432, 88.54243821818161564 ) ) ;
#1599=CARTESIAN_POINT ( 'NONE',  ( 49.17500000054622689, 26.92701409722686634, 88.54243821818162985 ) ) ;
#1606=CARTESIAN_POINT ( 'NONE',  ( 21.05000000109246727, 27.13292387221364876, 88.47553407664153724 ) ) ;
#1610=CARTESIAN_POINT ( 'NONE',  ( 23.97500000054623115, 15.71886984736413417, 96.68563167572563088 ) ) ;
#1611=CARTESIAN_POINT ( 'NONE',  ( 24.57500000054622191, 13.80429023900056684, 86.29171490190961435 ) ) ;
#1614=CARTESIAN_POINT ( 'NONE',  ( 44.99999999999999289, 20.00000000000000355, 83.29316153445364534 ) ) ;
#1615=ORIENTED_EDGE ( 'NONE', *, *, #7849, .T. ) ;
#1616=CARTESIAN_POINT ( 'NONE',  ( 39.55000000109246372, 22.43689772174679575, 98.29316153445363113 ) ) ;
#1617=ORIENTED_EDGE ( 'NONE', *, *, #9229, .F. ) ;
#1618=CARTESIAN_POINT ( 'NONE',  ( 30.05000000109246727, 12.86707612778636012, 93.11078899226572503 ) ) ;
#1619=ORIENTED_EDGE ( 'NONE', *, *, #5676, .F. ) ;
#1622=CARTESIAN_POINT ( 'NONE',  ( 19.97500000054623115, 15.71886984736413417, 96.68563167572563088 ) ) ;
#1623=( BOUNDED_CURVE ( )  B_SPLINE_CURVE ( 2, ( #3041, #8876, #8946, #2153, #1894, #4947, #8690, #1081, #62, #8811, #10645 ),
 .UNSPECIFIED., .F., .F. ) 
 B_SPLINE_CURVE_WITH_KNOTS ( ( 3, 2, 2, 2, 2, 3 ),
 ( 0.8333333333333333703, 0.8399999999999999689, 0.8466666666666666785, 0.8533333333333333881, 0.8599999999999999867, 0.8666666666666666963 ),
 .UNSPECIFIED. ) 
 CURVE ( )  GEOMETRIC_REPRESENTATION_ITEM ( )  RATIONAL_B_SPLINE_CURVE ( ( 1.000000000000000000, 0.9510565162951535312, 1.000000000000000000, 0.9510565162951535312, 1.000000000000000000, 0.9510565162951535312, 1.000000000000000000, 0.9510565162951535312, 1.000000000000000000, 0.9510565162951535312, 1.000000000000000000 ) ) 
 REPRESENTATION_ITEM ( '' )  );
#1625=CARTESIAN_POINT ( 'NONE',  ( 27.49999999999998579, 27.88596668178699645, 90.79316153445363113 ) ) ;
#1627=EDGE_CURVE ( 'NONE', #58, #10066, #662, .T. ) ;
#1629=DIRECTION ( 'NONE',  ( -0.000000000000000000, -0.000000000000000000, -1.000000000000000000 ) ) ;
#1630=CARTESIAN_POINT ( 'NONE',  ( 26.97500000054622760, 24.28113015263587471, 84.90069139318163138 ) ) ;
#1632=CARTESIAN_POINT ( 'NONE',  ( 47.65000000109246514, 20.00000000000000355, 98.29316153445363113 ) ) ;
#1634=DIRECTION ( 'NONE',  ( 0.000000000000000000, 0.000000000000000000, -1.000000000000000000 ) ) ;
#1636=CARTESIAN_POINT ( 'NONE',  ( 39.67500000054623399, 22.36655054427230027, 98.07665518445361386 ) ) ;
#1637=CARTESIAN_POINT ( 'NONE',  ( 39.27500000054622831, 26.92701409722686634, 88.54243821818162985 ) ) ;
#1638=CARTESIAN_POINT ( 'NONE',  ( 28.77500000054622831, 20.00000000000000355, 83.50966788445364841 ) ) ;
#1639=CARTESIAN_POINT ( 'NONE',  ( -27.49999999999999645, 20.00000000000000355, 99.99999999999997158 ) ) ;
#1642=CARTESIAN_POINT ( 'NONE',  ( 4.999999999999998224, 18.00000000000000355, 152.2284161474004520 ) ) ;
#1644=ORIENTED_EDGE ( 'NONE', *, *, #6426, .F. ) ;
#1649=ADVANCED_FACE ( 'NONE', ( #9304 ), #424, .F. ) ;
#1650=CARTESIAN_POINT ( 'NONE',  ( 29.67500000054622333, 24.28113015263587116, 96.68563167572563088 ) ) ;
#1651=CARTESIAN_POINT ( 'NONE',  ( 26.85000000109246443, 24.40838939219355197, 84.72553407664153724 ) ) ;
#1652=CARTESIAN_POINT ( 'NONE',  ( 48.87500000054622262, 22.36655054427230382, 83.50966788445364841 ) ) ;
#1653=EDGE_CURVE ( 'NONE', #12416, #3301, #8224, .T. ) ;
#1654=CARTESIAN_POINT ( 'NONE',  ( 33.77500000054623541, 22.36655054427230027, 98.07665518445361386 ) ) ;
#1655=CARTESIAN_POINT ( 'NONE',  ( 29.79999999999998650, 24.40838939219354842, 96.86078899226572503 ) ) ;
#1657=CARTESIAN_POINT ( 'NONE',  ( 38.17500000054622689, 13.07298590277314254, 93.04388485072563242 ) ) ;
#1658=ORIENTED_EDGE ( 'NONE', *, *, #1399, .F. ) ;
#1659=CARTESIAN_POINT ( 'NONE',  ( 20.05000000109246372, 12.86707612778636012, 93.11078899226572503 ) ) ;
#1661=ORIENTED_EDGE ( 'NONE', *, *, #6688, .T. ) ;
#1663=ORIENTED_EDGE ( 'NONE', *, *, #10791, .F. ) ;
#1667=DIRECTION ( 'NONE',  ( 0.000000000000000000, 0.000000000000000000, -1.000000000000000000 ) ) ;
#1668=CARTESIAN_POINT ( 'NONE',  ( 21.67500000054622689, 22.36655054427230027, 98.07665518445361386 ) ) ;
#1669=CARTESIAN_POINT ( 'NONE',  ( 49.99999999999998579, 20.00000000000000355, 98.29316153445363113 ) ) ;
#1671=DIRECTION ( 'NONE',  ( -1.000000000000000000, 0.000000000000000000, 0.000000000000000000 ) ) ;
#1673=CARTESIAN_POINT ( 'NONE',  ( 35.35000000109246798, 26.37988106264029398, 95.42841645007781892 ) ) ;
#1686=CARTESIAN_POINT ( 'NONE',  ( 21.87500000054622973, 17.63344945572769973, 98.07665518445361386 ) ) ;
#1690=VERTEX_POINT ( 'NONE', #7326 ) ;
#1692=DIRECTION ( 'NONE',  ( 0.000000000000000000, 0.000000000000000000, 1.000000000000000000 ) ) ;
#1694=CARTESIAN_POINT ( 'NONE',  ( 29.65000000109246514, 20.00000000000000355, 98.29316153445363113 ) ) ;
#1695=CARTESIAN_POINT ( 'NONE',  ( 39.97500000054623115, 17.63344945572769973, 98.07665518445361386 ) ) ;
#1696=VECTOR ( 'NONE', #4340, 1000.000000000000000 ) ;
#1697=CARTESIAN_POINT ( 'NONE',  ( 23.27500000054622475, 27.65831843345427998, 90.79316153445363113 ) ) ;
#1698=CARTESIAN_POINT ( 'NONE',  ( 9.796481954667255465, 17.97777750360451066, 98.01975852014066959 ) ) ;
#1701=EDGE_CURVE ( 'NONE', #3198, #4057, #5498, .T. ) ;
#1703=DIRECTION ( 'NONE',  ( 0.000000000000000000, 0.000000000000000000, 1.000000000000000000 ) ) ;
#1706=LINE ( 'NONE', #883, #10755 ) ;
#1708=VECTOR ( 'NONE', #10819, 1000.000000000000000 ) ;
#1709=CARTESIAN_POINT ( 'NONE',  ( 28.27500000054622475, 13.07298590277314254, 93.04388485072563242 ) ) ;
#1710=CARTESIAN_POINT ( 'NONE',  ( 36.87500000054622973, 22.36655054427230382, 83.50966788445364841 ) ) ;
#1711=CARTESIAN_POINT ( 'NONE',  ( 25.87500000054622618, 20.00000000000000355, 98.07665518445361386 ) ) ;
#1712=CARTESIAN_POINT ( 'NONE',  ( 30.09999999999999076, 17.56310227825320425, 98.29316153445363113 ) ) ;
#1713=EDGE_CURVE ( 'NONE', #9005, #7706, #9367, .T. ) ;
#1715=CARTESIAN_POINT ( 'NONE',  ( 42.07500000054623257, 13.80429023900056507, 95.29460816699764791 ) ) ;
#1716=VERTEX_POINT ( 'NONE', #8163 ) ;
#1718=CARTESIAN_POINT ( 'NONE',  ( 21.25000000109246301, 27.13292387221364876, 93.11078899226573924 ) ) ;
#1719=CARTESIAN_POINT ( 'NONE',  ( 27.95000000109246585, 13.62011893735970958, 95.42841645007781892 ) ) ;
#1720=ORIENTED_EDGE ( 'NONE', *, *, #9869, .T. ) ;
#1724=EDGE_CURVE ( 'NONE', #110, #2004, #4550, .T. ) ;
#1727=DIRECTION ( 'NONE',  ( 0.000000000000000000, 0.000000000000000000, -1.000000000000000000 ) ) ;
#1728=CARTESIAN_POINT ( 'NONE',  ( 42.77500000054622120, 17.63344945572770328, 83.50966788445364841 ) ) ;
#1729=CARTESIAN_POINT ( 'NONE',  ( -27.49999999999999645, 20.00000000000000355, 170.0000119999999697 ) ) ;
#1730=CARTESIAN_POINT ( 'NONE',  ( 43.97500000054622404, 17.63344945572769973, 98.07665518445361386 ) ) ;
#1731=CARTESIAN_POINT ( 'NONE',  ( 46.29999999999999005, 13.62011893735971135, 95.42841645007781892 ) ) ;
#1735=CARTESIAN_POINT ( 'NONE',  ( 40.05000000109246372, 12.86707612778636012, 93.11078899226572503 ) ) ;
#1737=ORIENTED_EDGE ( 'NONE', *, *, #11608, .T. ) ;
#1743=CARTESIAN_POINT ( 'NONE',  ( 0.000000000000000000, 20.00000000000000355, 109.9999999999999858 ) ) ;
#1744=DIRECTION ( 'NONE',  ( 0.000000000000000000, -0.000000000000000000, 1.000000000000000000 ) ) ;
#1745=CARTESIAN_POINT ( 'NONE',  ( 48.25000000109246656, 12.86707612778636012, 88.47553407664152303 ) ) ;
#1746=CARTESIAN_POINT ( 'NONE',  ( 49.57500000054621836, 26.19570976099943493, 95.29460816699764791 ) ) ;
#1751=CARTESIAN_POINT ( 'NONE',  ( 43.15000000109247225, 27.88596668178699645, 90.79316153445363113 ) ) ;
#1753=CARTESIAN_POINT ( 'NONE',  ( 40.77500000054622831, 17.63344945572770328, 83.50966788445364841 ) ) ;
#1754=CARTESIAN_POINT ( 'NONE',  ( 22.87500000054622973, 22.36655054427230382, 83.50966788445364841 ) ) ;
#1758=CARTESIAN_POINT ( 'NONE',  ( -111.8465843842649292, 84.49999999999998579, 146.8533255156881978 ) ) ;
#1761=ORIENTED_EDGE ( 'NONE', *, *, #10783, .F. ) ;
#1765=EDGE_CURVE ( 'NONE', #10983, #11823, #10301, .T. ) ;
#1766=CARTESIAN_POINT ( 'NONE',  ( 28.37500000054622262, 12.34168156654572357, 90.79316153445363113 ) ) ;
#1767=CARTESIAN_POINT ( 'NONE',  ( 29.45000000109246230, 24.40838939219354842, 96.86078899226572503 ) ) ;
#1768=CARTESIAN_POINT ( 'NONE',  ( 37.17500000054622689, 26.92701409722686634, 88.54243821818162985 ) ) ;
#1769=CARTESIAN_POINT ( 'NONE',  ( 24.97500000054622049, 22.36655054427230382, 83.50966788445364841 ) ) ;
#1770=CARTESIAN_POINT ( 'NONE',  ( 31.69999999999999218, 26.37988106264029398, 95.42841645007781892 ) ) ;
#1771=CARTESIAN_POINT ( 'NONE',  ( 49.99999999999998579, 20.00000000000000355, 98.29316153445363113 ) ) ;
#1772=CARTESIAN_POINT ( 'NONE',  ( 42.27500000054622831, 12.34168156654572535, 90.79316153445363113 ) ) ;
#1775=CARTESIAN_POINT ( 'NONE',  ( 46.77500000054622831, 20.00000000000000355, 83.50966788445364841 ) ) ;
#1781=DIRECTION ( 'NONE',  ( 0.000000000000000000, 0.000000000000000000, -1.000000000000000000 ) ) ;
#1783=CARTESIAN_POINT ( 'NONE',  ( 20.00000000000001421, 24.39339828220178674, 137.5000000000000000 ) ) ;
#1786=CARTESIAN_POINT ( 'NONE',  ( 43.87500000054622973, 20.00000000000000355, 98.07665518445361386 ) ) ;
#1789=CARTESIAN_POINT ( 'NONE',  ( 48.09999999999998721, 17.56310227825320425, 98.29316153445363113 ) ) ;
#1790=CARTESIAN_POINT ( 'NONE',  ( 41.69999999999998863, 26.37988106264029398, 95.42841645007781892 ) ) ;
#1795=CARTESIAN_POINT ( 'NONE',  ( 35.95000000109247651, 13.62011893735971135, 95.42841645007781892 ) ) ;
#1796=CARTESIAN_POINT ( 'NONE',  ( 24.89999999999998792, 17.56310227825320425, 83.29316153445363113 ) ) ;
#1797=ORIENTED_EDGE ( 'NONE', *, *, #6355, .F. ) ;
#1798=CARTESIAN_POINT ( 'NONE',  ( -27.49999999999999645, 20.00000000000000355, 170.0000119999999697 ) ) ;
#1799=VERTEX_POINT ( 'NONE', #12340 ) ;
#1801=EDGE_CURVE ( 'NONE', #3463, #5434, #2880, .T. ) ;
#1802=DIRECTION ( 'NONE',  ( 1.000000000000000000, -0.000000000000000000, -0.000000000000000000 ) ) ;
#1804=CARTESIAN_POINT ( 'NONE',  ( -5.000000000000000888, 40.00000000000000000, 121.2488769092545198 ) ) ;
#1805=AXIS2_PLACEMENT_3D ( 'NONE', #8515, #77, #7631 ) ;
#1807=CARTESIAN_POINT ( 'NONE',  ( 27.39999999999998792, 27.13292387221364876, 88.47553407664153724 ) ) ;
#1808=EDGE_LOOP ( 'NONE', ( #6497, #12280, #6021, #8100, #4860, #11044 ) ) ;
#1809=PLANE ( 'NONE',  #912 ) ;
#1811=CARTESIAN_POINT ( 'NONE',  ( 20.17500000054622689, 13.07298590277314254, 93.04388485072563242 ) ) ;
#1814=ORIENTED_EDGE ( 'NONE', *, *, #4472, .F. ) ;
#1816=CARTESIAN_POINT ( 'NONE',  ( 21.69999999999998508, 26.37988106264029398, 95.42841645007781892 ) ) ;
#1817=VECTOR ( 'NONE', #6496, 1000.000000000000000 ) ;
#1819=CARTESIAN_POINT ( 'NONE',  ( 20.17500000054622689, 13.07298590277314254, 93.04388485072563242 ) ) ;
#1823=CARTESIAN_POINT ( 'NONE',  ( 26.65000000109246514, 20.00000000000000355, 83.29316153445364534 ) ) ;
#1828=ADVANCED_FACE ( 'NONE', ( #3110 ), #8528, .F. ) ;
#1831=CARTESIAN_POINT ( 'NONE',  ( 28.87500000054622262, 20.00000000000000355, 83.50966788445364841 ) ) ;
#1832=CARTESIAN_POINT ( 'NONE',  ( -2.000000000000015543, 20.00000000000000355, 98.29316153445363113 ) ) ;
#1833=CARTESIAN_POINT ( 'NONE',  ( 40.87500000054622973, 22.36655054427230382, 83.50966788445364841 ) ) ;
#1834=CARTESIAN_POINT ( 'NONE',  ( 28.17500000054621978, 13.80429023900056507, 95.29460816699764791 ) ) ;
#1835=CARTESIAN_POINT ( 'NONE',  ( 26.59999999999998721, 12.86707612778636012, 88.47553407664152303 ) ) ;
#1837=CARTESIAN_POINT ( 'NONE',  ( 30.69999999999998863, 13.62011893735970958, 86.15790661882942914 ) ) ;
#1838=CARTESIAN_POINT ( 'NONE',  ( 36.07500000054622546, 13.80429023900056507, 95.29460816699764791 ) ) ;
#1840=CARTESIAN_POINT ( 'NONE',  ( 46.27500000054622120, 12.34168156654572535, 90.79316153445363113 ) ) ;
#1841=CARTESIAN_POINT ( 'NONE',  ( 27.75000000109246301, 17.56310227825320425, 98.29316153445363113 ) ) ;
#1845=CARTESIAN_POINT ( 'NONE',  ( -2.000000000000015543, 20.00000000000000355, 83.29316153445364534 ) ) ;
#1846=CARTESIAN_POINT ( 'NONE',  ( 32.59999999999998721, 12.86707612778636012, 88.47553407664152303 ) ) ;
#1848=CARTESIAN_POINT ( 'NONE',  ( 46.97500000054621694, 22.36655054427230382, 83.50966788445364841 ) ) ;
#1849=DIRECTION ( 'NONE',  ( 0.000000000000000000, 0.000000000000000000, -1.000000000000000000 ) ) ;
#1850=EDGE_CURVE ( 'NONE', #9812, #2033, #12400, .T. ) ;
#1852=CARTESIAN_POINT ( 'NONE',  ( 42.47500000054623115, 13.07298590277314432, 88.54243821818161564 ) ) ;
#1853=CARTESIAN_POINT ( 'NONE',  ( 49.19999999999998863, 24.40838939219355197, 84.72553407664153724 ) ) ;
#1854=CARTESIAN_POINT ( 'NONE',  ( 41.59999999999998721, 27.13292387221364876, 93.11078899226573924 ) ) ;
#1855=DIRECTION ( 'NONE',  ( 0.000000000000000000, 0.000000000000000000, 1.000000000000000000 ) ) ;
#1858=CARTESIAN_POINT ( 'NONE',  ( 36.05000000109246372, 12.86707612778636012, 93.11078899226572503 ) ) ;
#1860=ORIENTED_EDGE ( 'NONE', *, *, #8899, .F. ) ;
#1866=CARTESIAN_POINT ( 'NONE',  ( 38.47500000054621694, 13.80429023900056684, 86.29171490190961435 ) ) ;
#1868=CARTESIAN_POINT ( 'NONE',  ( 4.999999999999999112, 0.000000000000000000, 169.9999999999999716 ) ) ;
#1869=ORIENTED_EDGE ( 'NONE', *, *, #2322, .T. ) ;
#1873=CARTESIAN_POINT ( 'NONE',  ( 49.27500000054622120, 26.92701409722686634, 88.54243821818162985 ) ) ;
#1874=ORIENTED_EDGE ( 'NONE', *, *, #2151, .T. ) ;
#1875=CARTESIAN_POINT ( 'NONE',  ( -21.20617189303577987, 25.37779564132841159, 151.2938281069642130 ) ) ;
#1881=DIRECTION ( 'NONE',  ( 0.000000000000000000, 0.000000000000000000, -1.000000000000000000 ) ) ;
#1884=CARTESIAN_POINT ( 'NONE',  ( 21.07500000054622546, 26.19570976099943849, 86.29171490190961435 ) ) ;
#1885=CARTESIAN_POINT ( 'NONE',  ( 9.960637755725160858, 18.97835903059869622, 98.24092394347138679 ) ) ;
#1890=ORIENTED_EDGE ( 'NONE', *, *, #7052, .F. ) ;
#1891=CARTESIAN_POINT ( 'NONE',  ( 37.55000000109244951, 22.43689772174683128, 98.29316153445361692 ) ) ;
#1894=CARTESIAN_POINT ( 'NONE',  ( 24.25000000109246301, 12.86707612778636012, 88.47553407664152303 ) ) ;
#1895=CARTESIAN_POINT ( 'NONE',  ( 38.67500000054623399, 17.63344945572770328, 83.50966788445364841 ) ) ;
#1896=CARTESIAN_POINT ( 'NONE',  ( 26.47500000054622404, 13.07298590277314432, 88.54243821818161564 ) ) ;
#1897=CARTESIAN_POINT ( 'NONE',  ( 31.29999999999998650, 26.37988106264029398, 86.15790661882942914 ) ) ;
#1898=ADVANCED_FACE ( 'NONE', ( #3762 ), #5558, .F. ) ;
#1899=CARTESIAN_POINT ( 'NONE',  ( 30.37500000054622973, 13.07298590277314432, 88.54243821818161564 ) ) ;
#1900=ORIENTED_EDGE ( 'NONE', *, *, #11408, .T. ) ;
#1904=ORIENTED_EDGE ( 'NONE', *, *, #9414, .T. ) ;
#1906=CARTESIAN_POINT ( 'NONE',  ( 27.50000000000000355, 27.49999999999999645, 145.0000000000000000 ) ) ;
#1908=CARTESIAN_POINT ( 'NONE',  ( 45.37500000054622973, 27.65831843345427998, 90.79316153445363113 ) ) ;
#1910=CARTESIAN_POINT ( 'NONE',  ( -50.00000000000001421, 69.50000000000000000, 101.8533255156881978 ) ) ;
#1911=CARTESIAN_POINT ( 'NONE',  ( 47.17500000054622689, 26.19570976099943493, 86.29171490190961435 ) ) ;
#1912=CARTESIAN_POINT ( 'NONE',  ( 21.17500000054622689, 26.19570976099943493, 86.29171490190961435 ) ) ;
#1913=CARTESIAN_POINT ( 'NONE',  ( 45.09999999999998721, 22.43689772174682417, 83.29316153445364534 ) ) ;
#1916=EDGE_LOOP ( 'NONE', ( #1063, #4190, #6240, #9780 ) ) ;
#1917=CARTESIAN_POINT ( 'NONE',  ( 31.35000000109246088, 26.37988106264029398, 95.42841645007781892 ) ) ;
#1919=ORIENTED_EDGE ( 'NONE', *, *, #7603, .T. ) ;
#1920=ADVANCED_FACE ( 'NONE', ( #2694, #4787 ), #12523, .T. ) ;
#1921=ORIENTED_EDGE ( 'NONE', *, *, #10279, .T. ) ;
#1925=CARTESIAN_POINT ( 'NONE',  ( -50.00000000000001421, 40.00000000000000000, 132.8533255156884820 ) ) ;
#1927=CARTESIAN_POINT ( 'NONE',  ( 36.57500000054622546, 15.71886984736413773, 84.90069139318163138 ) ) ;
#1930=CARTESIAN_POINT ( 'NONE',  ( 44.65000000109246514, 20.00000000000000355, 83.29316153445364534 ) ) ;
#1931=CARTESIAN_POINT ( 'NONE',  ( 33.85000000109246798, 15.59161060780645691, 96.86078899226572503 ) ) ;
#1935=CARTESIAN_POINT ( 'NONE',  ( 21.37500000054622618, 26.92701409722686634, 93.04388485072563242 ) ) ;
#1937=CARTESIAN_POINT ( 'NONE',  ( 46.05000000109246372, 12.86707612778636012, 93.11078899226572503 ) ) ;
#1939=EDGE_CURVE ( 'NONE', #10127, #9490, #8790, .T. ) ;
#1941=EDGE_LOOP ( 'NONE', ( #7827, #5400, #1312, #11371 ) ) ;
#1942=VERTEX_POINT ( 'NONE', #171 ) ;
#1943=CARTESIAN_POINT ( 'NONE',  ( 21.59999999999998721, 27.13292387221364876, 93.11078899226573924 ) ) ;
#1944=EDGE_CURVE ( 'NONE', #8208, #113, #237, .T. ) ;
#1949=DIRECTION ( 'NONE',  ( 0.000000000000000000, -0.000000000000000000, 1.000000000000000000 ) ) ;
#1951=( BOUNDED_CURVE ( )  B_SPLINE_CURVE ( 2, ( #2547, #7560, #8332, #6660, #9348, #10529, #897, #1719, #10343, #1841, #9590 ),
 .UNSPECIFIED., .F., .F. ) 
 B_SPLINE_CURVE_WITH_KNOTS ( ( 3, 2, 2, 2, 2, 3 ),
 ( 0.6999999999999999556, 0.7066666666666666652, 0.7133333333333333748, 0.7199999999999999734, 0.7266666666666666829, 0.7333333333333332815 ),
 .UNSPECIFIED. ) 
 CURVE ( )  GEOMETRIC_REPRESENTATION_ITEM ( )  RATIONAL_B_SPLINE_CURVE ( ( 1.000000000000000000, 0.9510565162951535312, 1.000000000000000000, 0.9510565162951535312, 1.000000000000000000, 0.9510565162951535312, 1.000000000000000000, 0.9510565162951535312, 1.000000000000000000, 0.9510565162951535312, 1.000000000000000000 ) ) 
 REPRESENTATION_ITEM ( '' )  );
#1952=EDGE_CURVE ( 'NONE', #9442, #5929, #11048, .T. ) ;
#1960=CARTESIAN_POINT ( 'NONE',  ( 39.57500000054622546, 24.28113015263587116, 96.68563167572563088 ) ) ;
#1961=CARTESIAN_POINT ( 'NONE',  ( 28.97500000054622404, 22.36655054427230382, 83.50966788445364841 ) ) ;
#1962=CARTESIAN_POINT ( 'NONE',  ( 25.59999999999998721, 27.13292387221364876, 93.11078899226573924 ) ) ;
#1963=CARTESIAN_POINT ( 'NONE',  ( 34.19999999999998863, 15.59161060780645691, 96.86078899226572503 ) ) ;
#1964=CARTESIAN_POINT ( 'NONE',  ( 34.97500000054623115, 24.28113015263587471, 84.90069139318163138 ) ) ;
#1971=CARTESIAN_POINT ( 'NONE',  ( -50.00000000000001421, 77.00000000000000000, 94.35332551568819781 ) ) ;
#1972=CARTESIAN_POINT ( 'NONE',  ( 47.57500000054621836, 26.19570976099943849, 95.29460816699764791 ) ) ;
#1973=DIRECTION ( 'NONE',  ( 0.000000000000000000, 1.000000000000000000, 0.000000000000000000 ) ) ;
#1974=DIRECTION ( 'NONE',  ( 0.000000000000000000, 0.000000000000000000, -1.000000000000000000 ) ) ;
#1975=CARTESIAN_POINT ( 'NONE',  ( 44.47500000054622404, 13.07298590277314432, 88.54243821818161564 ) ) ;
#1976=CARTESIAN_POINT ( 'NONE',  ( 39.69999999999997442, 26.37988106264029398, 95.42841645007781892 ) ) ;
#1977=CARTESIAN_POINT ( 'NONE',  ( 40.49999999999998579, 12.11403331821300533, 90.79316153445363113 ) ) ;
#1978=LINE ( 'NONE', #9732, #5852 ) ;
#1980=CARTESIAN_POINT ( 'NONE',  ( 33.95000000109246940, 13.62011893735971135, 95.42841645007781892 ) ) ;
#1981=FACE_BOUND ( 'NONE', #10869, .T. ) ;
#1982=EDGE_LOOP ( 'NONE', ( #9506, #9877, #7134, #2757, #7198 ) ) ;
#1984=ORIENTED_EDGE ( 'NONE', *, *, #1388, .T. ) ;
#1985=CARTESIAN_POINT ( 'NONE',  ( -34.72841614740048044, 22.00000000000000000, 152.2284161474004520 ) ) ;
#1990=CARTESIAN_POINT ( 'NONE',  ( 33.87500000054621552, 17.63344945572769973, 98.07665518445361386 ) ) ;
#1991=CARTESIAN_POINT ( 'NONE',  ( 40.67500000054622689, 15.71886984736413773, 84.90069139318163138 ) ) ;
#1992=CARTESIAN_POINT ( 'NONE',  ( 34.75000000109243814, 22.43689772174679575, 83.29316153445363113 ) ) ;
#1994=CARTESIAN_POINT ( 'NONE',  ( -2.000000000000015543, 20.00000000000000355, 90.79316153445363113 ) ) ;
#1996=VERTEX_POINT ( 'NONE', #1998 ) ;
#1997=CARTESIAN_POINT ( 'NONE',  ( 48.65000000109246514, 20.00000000000000355, 83.29316153445364534 ) ) ;
#1998=CARTESIAN_POINT ( 'NONE',  ( 28.99999999999998934, 20.00000000000000355, 83.29316153445364534 ) ) ;
#1999=ORIENTED_EDGE ( 'NONE', *, *, #6207, .F. ) ;
#2002=ORIENTED_EDGE ( 'NONE', *, *, #1262, .F. ) ;
#2004=VERTEX_POINT ( 'NONE', #5878 ) ;
#2006=CARTESIAN_POINT ( 'NONE',  ( 21.49999999999998934, 27.88596668178699645, 90.79316153445363113 ) ) ;
#2008=EDGE_CURVE ( 'NONE', #11777, #5465, #109, .T. ) ;
#2009=CARTESIAN_POINT ( 'NONE',  ( 9.919782953541179893, 21.28887143972310625, 83.40037394667403703 ) ) ;
#2019=CARTESIAN_POINT ( 'NONE',  ( 24.17500000054622333, 13.80429023900056507, 95.29460816699764791 ) ) ;
#2020=CARTESIAN_POINT ( 'NONE',  ( 49.77500000054621410, 22.36655054427230027, 98.07665518445361386 ) ) ;
#2021=CARTESIAN_POINT ( 'NONE',  ( 34.07500000054622546, 13.80429023900056507, 95.29460816699764791 ) ) ;
#2022=( BOUNDED_CURVE ( )  B_SPLINE_CURVE ( 3, ( #2325, #111, #11776, #3970 ),
 .UNSPECIFIED., .F., .F. ) 
 B_SPLINE_CURVE_WITH_KNOTS ( ( 4, 4 ),
 ( 4.712388980384689674, 6.283185307179585344 ),
 .UNSPECIFIED. ) 
 CURVE ( )  GEOMETRIC_REPRESENTATION_ITEM ( )  RATIONAL_B_SPLINE_CURVE ( ( 1.000000000000000000, 0.8047378541243649375, 0.8047378541243649375, 1.000000000000000000 ) ) 
 REPRESENTATION_ITEM ( '' )  );
#2024=CARTESIAN_POINT ( 'NONE',  ( 25.39999999999998792, 27.13292387221364876, 88.47553407664153724 ) ) ;
#2025=CARTESIAN_POINT ( 'NONE',  ( 49.49999999999997868, 27.88596668178699645, 90.79316153445363113 ) ) ;
#2026=CARTESIAN_POINT ( 'NONE',  ( 30.87500000054622618, 22.36655054427230382, 83.50966788445364841 ) ) ;
#2027=ORIENTED_EDGE ( 'NONE', *, *, #456, .F. ) ;
#2030=DIRECTION ( 'NONE',  ( -0.000000000000000000, -0.000000000000000000, -1.000000000000000000 ) ) ;
#2031=VERTEX_POINT ( 'NONE', #10186 ) ;
#2032=CARTESIAN_POINT ( 'NONE',  ( 48.95000000109246940, 26.37988106264029398, 86.15790661882942914 ) ) ;
#2033=VERTEX_POINT ( 'NONE', #8347 ) ;
#2035=CARTESIAN_POINT ( 'NONE',  ( -2.000000000000015543, 20.00000000000000355, 98.29316153445363113 ) ) ;
#2037=CARTESIAN_POINT ( 'NONE',  ( 37.27500000054622831, 26.92701409722686634, 88.54243821818162985 ) ) ;
#2039=CARTESIAN_POINT ( 'NONE',  ( -34.72841614740047333, 18.00000000000000355, 152.2284161474004520 ) ) ;
#2040=CARTESIAN_POINT ( 'NONE',  ( 37.47500000054622404, 26.92701409722686634, 93.04388485072563242 ) ) ;
#2041=CARTESIAN_POINT ( 'NONE',  ( 39.79999999999999005, 24.40838939219354842, 96.86078899226572503 ) ) ;
#2042=CARTESIAN_POINT ( 'NONE',  ( 40.19999999999998863, 15.59161060780645691, 96.86078899226572503 ) ) ;
#2045=CARTESIAN_POINT ( 'NONE',  ( 29.05000000109246727, 27.13292387221364876, 88.47553407664153724 ) ) ;
#2047=ORIENTED_EDGE ( 'NONE', *, *, #94, .F. ) ;
#2053=CARTESIAN_POINT ( 'NONE',  ( 35.97500000054623115, 15.71886984736413417, 96.68563167572563088 ) ) ;
#2054=CARTESIAN_POINT ( 'NONE',  ( 31.97500000054622760, 17.63344945572769973, 98.07665518445361386 ) ) ;
#2057=DIRECTION ( 'NONE',  ( 1.000000000000000000, 0.000000000000000000, 0.000000000000000000 ) ) ;
#2059=CARTESIAN_POINT ( 'NONE',  ( 49.47500000054623115, 26.92701409722686634, 93.04388485072563242 ) ) ;
#2068=CARTESIAN_POINT ( 'NONE',  ( -31.00470515163596019, 27.49999999999999645, 148.5047051516359318 ) ) ;
#2069=CARTESIAN_POINT ( 'NONE',  ( 7.928408809296215054, 26.09658529048988740, 95.16773376593604894 ) ) ;
#2070=CARTESIAN_POINT ( 'NONE',  ( 43.99999999999999289, 20.00000000000000355, 98.29316153445363113 ) ) ;
#2071=DIRECTION ( 'NONE',  ( 1.000000000000000000, -0.000000000000000000, -0.000000000000000000 ) ) ;
#2072=LINE ( 'NONE', #5003, #10396 ) ;
#2074=CARTESIAN_POINT ( 'NONE',  ( 41.17500000054623399, 26.92701409722686634, 88.54243821818162985 ) ) ;
#2084=CARTESIAN_POINT ( 'NONE',  ( 48.27500000054622831, 13.07298590277314254, 93.04388485072563242 ) ) ;
#2086=CARTESIAN_POINT ( 'NONE',  ( 35.17500000054622689, 26.92701409722686634, 88.54243821818162985 ) ) ;
#2087=CARTESIAN_POINT ( 'NONE',  ( 20.47500000054622404, 13.07298590277314432, 88.54243821818161564 ) ) ;
#2088=CARTESIAN_POINT ( 'NONE',  ( 24.99999999999998579, 20.00000000000000355, 83.29316153445364534 ) ) ;
#2089=CARTESIAN_POINT ( 'NONE',  ( 49.79999999999999005, 24.40838939219354842, 96.86078899226572503 ) ) ;
#2090=CARTESIAN_POINT ( 'NONE',  ( 30.47500000054622404, 13.80429023900056684, 86.29171490190961435 ) ) ;
#2091=ORIENTED_EDGE ( 'NONE', *, *, #6451, .T. ) ;
#2099=CARTESIAN_POINT ( 'NONE',  ( 40.27500000054622120, 13.07298590277314254, 93.04388485072563242 ) ) ;
#2102=CARTESIAN_POINT ( 'NONE',  ( 49.67500000054621978, 22.36655054427230027, 98.07665518445361386 ) ) ;
#2103=CARTESIAN_POINT ( 'NONE',  ( 41.17500000054621978, 26.19570976099943493, 86.29171490190961435 ) ) ;
#2104=CARTESIAN_POINT ( 'NONE',  ( 44.09999999999998010, 17.56310227825320425, 98.29316153445363113 ) ) ;
#2105=VECTOR ( 'NONE', #12328, 1000.000000000000000 ) ;
#2110=CARTESIAN_POINT ( 'NONE',  ( 29.35000000109245732, 26.37988106264029398, 95.42841645007781892 ) ) ;
#2113=EDGE_CURVE ( 'NONE', #8906, #11777, #788, .T. ) ;
#2114=EDGE_CURVE ( 'NONE', #6763, #2160, #5850, .T. ) ;
#2115=ORIENTED_EDGE ( 'NONE', *, *, #908, .T. ) ;
#2118=AXIS2_PLACEMENT_3D ( 'NONE', #11844, #5419, #9289 ) ;
#2119=CARTESIAN_POINT ( 'NONE',  ( -50.00000000000001421, 0.000000000000000000, 69.99999999999998579 ) ) ;
#2120=CARTESIAN_POINT ( 'NONE',  ( 28.77500000054622831, 20.00000000000000355, 83.50966788445364841 ) ) ;
#2121=CARTESIAN_POINT ( 'NONE',  ( 32.57500000054621836, 13.80429023900056684, 86.29171490190961435 ) ) ;
#2122=CARTESIAN_POINT ( 'NONE',  ( 44.25000000109246656, 12.86707612778636012, 88.47553407664152303 ) ) ;
#2125=CARTESIAN_POINT ( 'NONE',  ( 49.37500000054622262, 27.65831843345427998, 90.79316153445363113 ) ) ;
#2135=CARTESIAN_POINT ( 'NONE',  ( 27.49999999999999645, 20.00000000000000355, 170.0000119999999697 ) ) ;
#2139=DIRECTION ( 'NONE',  ( 1.000000000000000000, -0.000000000000000000, -0.000000000000000000 ) ) ;
#2142=LINE ( 'NONE', #1261, #9038 ) ;
#2143=CARTESIAN_POINT ( 'NONE',  ( 44.07500000054623968, 13.80429023900056507, 95.29460816699764791 ) ) ;
#2149=( BOUNDED_CURVE ( )  B_SPLINE_CURVE ( 3, ( #6892, #8992, #3913, #10631 ),
 .UNSPECIFIED., .F., .F. ) 
 B_SPLINE_CURVE_WITH_KNOTS ( ( 4, 4 ),
 ( 3.141592653589793560, 4.712388980384689674 ),
 .UNSPECIFIED. ) 
 CURVE ( )  GEOMETRIC_REPRESENTATION_ITEM ( )  RATIONAL_B_SPLINE_CURVE ( ( 1.000000000000000000, 0.8047378541243650485, 0.8047378541243650485, 1.000000000000000000 ) ) 
 REPRESENTATION_ITEM ( '' )  );
#2151=EDGE_CURVE ( 'NONE', #1332, #8919, #2692, .T. ) ;
#2152=CARTESIAN_POINT ( 'NONE',  ( 20.67500000054622689, 15.71886984736413773, 84.90069139318163138 ) ) ;
#2153=CARTESIAN_POINT ( 'NONE',  ( 24.35000000109246798, 13.62011893735970958, 86.15790661882942914 ) ) ;
#2155=CARTESIAN_POINT ( 'NONE',  ( 34.37500000054622973, 13.07298590277314432, 88.54243821818161564 ) ) ;
#2156=CARTESIAN_POINT ( 'NONE',  ( 21.77500000054622831, 22.36655054427230027, 98.07665518445361386 ) ) ;
#2157=CARTESIAN_POINT ( 'NONE',  ( 26.09999999999998721, 17.56310227825320425, 98.29316153445363113 ) ) ;
#2159=CARTESIAN_POINT ( 'NONE',  ( 29.17500000054623044, 26.92701409722686634, 88.54243821818162985 ) ) ;
#2160=VERTEX_POINT ( 'NONE', #4596 ) ;
#2168=CARTESIAN_POINT ( 'NONE',  ( 37.57500000054622546, 26.19570976099943849, 95.29460816699764791 ) ) ;
#2169=DIRECTION ( 'NONE',  ( 0.000000000000000000, -0.000000000000000000, 1.000000000000000000 ) ) ;
#2170=CARTESIAN_POINT ( 'NONE',  ( 26.09999999999998366, 17.56310227825320425, 98.29316153445363113 ) ) ;
#2171=CARTESIAN_POINT ( 'NONE',  ( 40.97500000054622404, 22.36655054427230382, 83.50966788445364841 ) ) ;
#2172=CARTESIAN_POINT ( 'NONE',  ( 39.99999999999998579, 20.00000000000000355, 98.29316153445363113 ) ) ;
#2175=DIRECTION ( 'NONE',  ( -1.000000000000000000, 0.000000000000000000, 0.000000000000000000 ) ) ;
#2178=CARTESIAN_POINT ( 'NONE',  ( 31.15000000109245804, 27.88596668178699645, 90.79316153445363113 ) ) ;
#2179=CARTESIAN_POINT ( 'NONE',  ( 40.65000000109246514, 20.00000000000000355, 83.29316153445364534 ) ) ;
#2187=PRODUCT_DEFINITION_CONTEXT ( 'detailed design', #7150, 'design' ) ;
#2189=CARTESIAN_POINT ( 'NONE',  ( 30.57500000054622902, 15.71886984736413773, 84.90069139318163138 ) ) ;
#2190=CARTESIAN_POINT ( 'NONE',  ( 29.97500000054622404, 17.63344945572769973, 98.07665518445361386 ) ) ;
#2196=CARTESIAN_POINT ( 'NONE',  ( 48.07500000054622546, 15.71886984736413417, 96.68563167572563088 ) ) ;
#2197=CARTESIAN_POINT ( 'NONE',  ( 48.25000000109246656, 12.86707612778636012, 88.47553407664152303 ) ) ;
#2200=DIRECTION ( 'NONE',  ( 0.000000000000000000, -0.000000000000000000, 1.000000000000000000 ) ) ;
#2203=CARTESIAN_POINT ( 'NONE',  ( -31.00470515163596019, 12.50000000000001066, 148.5047051516359318 ) ) ;
#2207=CARTESIAN_POINT ( 'NONE',  ( 49.77500000054622831, 20.00000000000000355, 98.07665518445361386 ) ) ;
#2209=CARTESIAN_POINT ( 'NONE',  ( 9.241050560303825989, 23.84658578115114480, 97.24969729302414123 ) ) ;
#2214=CIRCLE ( 'NONE', #4035, 10.00000000000000355 ) ;
#2216=CARTESIAN_POINT ( 'NONE',  ( 41.67500000054622689, 22.36655054427230027, 98.07665518445361386 ) ) ;
#2222=CARTESIAN_POINT ( 'NONE',  ( 20.77500000054622120, 17.63344945572770328, 83.50966788445364841 ) ) ;
#2223=CARTESIAN_POINT ( 'NONE',  ( 47.37500000054622973, 27.65831843345427998, 90.79316153445363113 ) ) ;
#2224=CARTESIAN_POINT ( 'NONE',  ( 34.67500000054621268, 17.63344945572770328, 83.50966788445364841 ) ) ;
#2225=VECTOR ( 'NONE', #4273, 1000.000000000000000 ) ;
#2226=CARTESIAN_POINT ( 'NONE',  ( 20.87500000054622262, 20.00000000000000355, 83.50966788445364841 ) ) ;
#2227=CARTESIAN_POINT ( 'NONE',  ( 25.99999999999998934, 20.00000000000000355, 98.29316153445363113 ) ) ;
#2229=CARTESIAN_POINT ( 'NONE',  ( 28.27500000054622475, 12.34168156654572535, 90.79316153445363113 ) ) ;
#2230=ORIENTED_EDGE ( 'NONE', *, *, #11650, .F. ) ;
#2237=ORIENTED_EDGE ( 'NONE', *, *, #7463, .T. ) ;
#2238=PLANE ( 'NONE',  #7415 ) ;
#2239=CARTESIAN_POINT ( 'NONE',  ( 39.37500000054622262, 27.65831843345427998, 90.79316153445363113 ) ) ;
#2240=DIRECTION ( 'NONE',  ( 1.000000000000000000, -0.000000000000000000, -0.000000000000000000 ) ) ;
#2241=DIRECTION ( 'NONE',  ( 1.000000000000000000, -0.000000000000000000, -0.000000000000000000 ) ) ;
#2242=CARTESIAN_POINT ( 'NONE',  ( 38.37500000054622973, 12.34168156654572535, 90.79316153445363113 ) ) ;
#2243=CARTESIAN_POINT ( 'NONE',  ( 41.79999999999999005, 24.40838939219354842, 96.86078899226572503 ) ) ;
#2244=VECTOR ( 'NONE', #2740, 1000.000000000000000 ) ;
#2245=CARTESIAN_POINT ( 'NONE',  ( 47.07500000054622546, 26.19570976099943493, 86.29171490190961435 ) ) ;
#2247=CARTESIAN_POINT ( 'NONE',  ( 23.55000000109246017, 22.43689772174679575, 98.29316153445363113 ) ) ;
#2249=VERTEX_POINT ( 'NONE', #2179 ) ;
#2250=DIRECTION ( 'NONE',  ( -1.000000000000000000, 0.000000000000000000, -0.000000000000000000 ) ) ;
#2251=VERTEX_POINT ( 'NONE', #10605 ) ;
#2252=CIRCLE ( 'NONE', #4058, 7.499999999999992895 ) ;
#2253=DIRECTION ( 'NONE',  ( 0.000000000000000000, 0.000000000000000000, -1.000000000000000000 ) ) ;
#2255=ADVANCED_FACE ( 'NONE', ( #1981, #4013 ), #5038, .F. ) ;
#2256=CARTESIAN_POINT ( 'NONE',  ( 27.47500000054622404, 26.19570976099943493, 95.29460816699764791 ) ) ;
#2257=CARTESIAN_POINT ( 'NONE',  ( 33.77500000054623541, 22.36655054427230027, 98.07665518445361386 ) ) ;
#2259=PLANE ( 'NONE',  #4747 ) ;
#2260=CARTESIAN_POINT ( 'NONE',  ( -5.000000000000000888, 0.000000000000000000, 169.9999999999999716 ) ) ;
#2261=CARTESIAN_POINT ( 'NONE',  ( 37.65000000109246514, 20.00000000000000355, 98.29316153445363113 ) ) ;
#2263=AXIS2_PLACEMENT_3D ( 'NONE', #7059, #11461, #2250 ) ;
#2264=CARTESIAN_POINT ( 'NONE',  ( 46.55000000109245661, 17.56310227825321135, 83.29316153445363113 ) ) ;
#2266=CARTESIAN_POINT ( 'NONE',  ( -32.89339828220179385, 84.49999999999998579, 151.2467237978899846 ) ) ;
#2267=ORIENTED_EDGE ( 'NONE', *, *, #2996, .T. ) ;
#2272=CARTESIAN_POINT ( 'NONE',  ( 9.842430534136942910, 21.78601360974349532, 83.50449544991025164 ) ) ;
#2273=CARTESIAN_POINT ( 'NONE',  ( 22.99999999999998934, 20.00000000000000355, 83.29316153445364534 ) ) ;
#2277=CARTESIAN_POINT ( 'NONE',  ( 42.07500000054623257, 13.80429023900056507, 95.29460816699764791 ) ) ;
#2282=CARTESIAN_POINT ( 'NONE',  ( 46.89999999999999858, 17.56310227825318648, 83.29316153445365956 ) ) ;
#2283=CARTESIAN_POINT ( 'NONE',  ( 46.17500000054622689, 13.80429023900056507, 95.29460816699764791 ) ) ;
#2284=CARTESIAN_POINT ( 'NONE',  ( 30.97500000054622760, 24.28113015263587471, 84.90069139318163138 ) ) ;
#2285=CARTESIAN_POINT ( 'NONE',  ( 21.87500000054622618, 20.00000000000000355, 98.07665518445361386 ) ) ;
#2287=CARTESIAN_POINT ( 'NONE',  ( 28.47500000054622404, 13.80429023900056684, 86.29171490190961435 ) ) ;
#2289=CARTESIAN_POINT ( 'NONE',  ( -19.99999999999999645, 20.00000000000000355, 170.0000119999999697 ) ) ;
#2291=ORIENTED_EDGE ( 'NONE', *, *, #11576, .T. ) ;
#2292=CARTESIAN_POINT ( 'NONE',  ( 38.10000000000000142, 17.56310227825315451, 98.29316153445357429 ) ) ;
#2296=CARTESIAN_POINT ( 'NONE',  ( 36.67500000054622689, 15.71886984736413773, 84.90069139318163138 ) ) ;
#2300=CARTESIAN_POINT ( 'NONE',  ( 42.37500000054621552, 12.34168156654572535, 90.79316153445363113 ) ) ;
#2301=CARTESIAN_POINT ( 'NONE',  ( 37.19999999999998863, 24.40838939219355197, 84.72553407664153724 ) ) ;
#2302=CARTESIAN_POINT ( 'NONE',  ( 47.67500000054622689, 22.36655054427230027, 98.07665518445361386 ) ) ;
#2303=EDGE_LOOP ( 'NONE', ( #8019, #1900, #4267, #4455 ) ) ;
#2305=CARTESIAN_POINT ( 'NONE',  ( 22.25000000109246656, 12.86707612778636012, 88.47553407664152303 ) ) ;
#2310=CARTESIAN_POINT ( 'NONE',  ( 24.75000000109246301, 22.43689772174679575, 83.29316153445363113 ) ) ;
#2311=CARTESIAN_POINT ( 'NONE',  ( 40.85000000109246088, 24.40838939219355197, 84.72553407664153724 ) ) ;
#2315=CARTESIAN_POINT ( 'NONE',  ( 29.97500000054622760, 15.71886984736413417, 96.68563167572563088 ) ) ;
#2316=CARTESIAN_POINT ( 'NONE',  ( 31.77500000054622475, 22.36655054427230027, 98.07665518445361386 ) ) ;
#2322=EDGE_CURVE ( 'NONE', #8906, #5150, #11889, .T. ) ;
#2323=CARTESIAN_POINT ( 'NONE',  ( 44.85000000109246798, 24.40838939219355197, 84.72553407664153724 ) ) ;
#2325=CARTESIAN_POINT ( 'NONE',  ( 27.50000000000000355, 12.50000000000001066, 145.0000000000000000 ) ) ;
#2327=VECTOR ( 'NONE', #6640, 1000.000000000000000 ) ;
#2330=CARTESIAN_POINT ( 'NONE',  ( 20.17500000054622689, 13.07298590277314254, 93.04388485072563242 ) ) ;
#2332=CARTESIAN_POINT ( 'NONE',  ( 31.99999999999998579, 20.00000000000000355, 98.29316153445363113 ) ) ;
#2344=CARTESIAN_POINT ( 'NONE',  ( 46.67500000054622689, 15.71886984736413773, 84.90069139318163138 ) ) ;
#2345=CARTESIAN_POINT ( 'NONE',  ( 25.57500000054622546, 24.28113015263587116, 96.68563167572563088 ) ) ;
#2347=CARTESIAN_POINT ( 'NONE',  ( 9.844713702461632465, 18.22664983694489749, 83.50141417594349491 ) ) ;
#2348=CARTESIAN_POINT ( 'NONE',  ( 44.85000000109246798, 24.40838939219355197, 84.72553407664153724 ) ) ;
#2350=CARTESIAN_POINT ( 'NONE',  ( 30.99999999999998934, 20.00000000000000355, 83.29316153445364534 ) ) ;
#2351=CARTESIAN_POINT ( 'NONE',  ( 27.07500000054622902, 26.19570976099943493, 86.29171490190961435 ) ) ;
#2353=FACE_OUTER_BOUND ( 'NONE', #11122, .T. ) ;
#2355=CARTESIAN_POINT ( 'NONE',  ( 37.99999999999999289, 20.00000000000000355, 98.29316153445363113 ) ) ;
#2356=ORIENTED_EDGE ( 'NONE', *, *, #8239, .T. ) ;
#2358=CARTESIAN_POINT ( 'NONE',  ( 31.27500000054622831, 26.92701409722686634, 88.54243821818162985 ) ) ;
#2360=CARTESIAN_POINT ( 'NONE',  ( 20.15000000109246514, 12.11403331821300533, 90.79316153445363113 ) ) ;
#2361=CARTESIAN_POINT ( 'NONE',  ( 34.87500000054622262, 20.00000000000000355, 83.50966788445364841 ) ) ;
#2362=CARTESIAN_POINT ( 'NONE',  ( 35.50000000000000000, 27.88596668178699645, 90.79316153445363113 ) ) ;
#2363=CARTESIAN_POINT ( 'NONE',  ( 46.27500000054622120, 12.34168156654572535, 90.79316153445363113 ) ) ;
#2365=CARTESIAN_POINT ( 'NONE',  ( 27.85000000109246443, 15.59161060780645691, 96.86078899226572503 ) ) ;
#2369=( BOUNDED_CURVE ( )  B_SPLINE_CURVE ( 2, ( #9596, #3748, #10594, #903, #1846, #8639, #4773, #2930, #4899, #10536, #2867 ),
 .UNSPECIFIED., .F., .F. ) 
 B_SPLINE_CURVE_WITH_KNOTS ( ( 3, 2, 2, 2, 2, 3 ),
 ( 0.5666666666666666519, 0.5733333333333333615, 0.5799999999999999600, 0.5866666666666666696, 0.5933333333333333792, 0.5999999999999999778 ),
 .UNSPECIFIED. ) 
 CURVE ( )  GEOMETRIC_REPRESENTATION_ITEM ( )  RATIONAL_B_SPLINE_CURVE ( ( 1.000000000000000000, 0.9510565162951535312, 1.000000000000000000, 0.9510565162951535312, 1.000000000000000000, 0.9510565162951535312, 1.000000000000000000, 0.9510565162951535312, 1.000000000000000000, 0.9510565162951535312, 1.000000000000000000 ) ) 
 REPRESENTATION_ITEM ( '' )  );
#2374=DIRECTION ( 'NONE',  ( 0.000000000000000000, 0.000000000000000000, -1.000000000000000000 ) ) ;
#2375=CARTESIAN_POINT ( 'NONE',  ( 33.37500000054622973, 26.92701409722686634, 93.04388485072563242 ) ) ;
#2376=CARTESIAN_POINT ( 'NONE',  ( 27.77500000054622475, 22.36655054427230027, 98.07665518445361386 ) ) ;
#2379=CARTESIAN_POINT ( 'NONE',  ( 43.75000000109246656, 17.56310227825320425, 98.29316153445363113 ) ) ;
#2382=DIRECTION ( 'NONE',  ( 1.000000000000000000, -0.000000000000000000, 0.000000000000000000 ) ) ;
#2392=DIRECTION ( 'NONE',  ( 1.000000000000000000, -0.000000000000000000, -0.000000000000000000 ) ) ;
#2393=EDGE_LOOP ( 'NONE', ( #2964, #2456, #5123, #3875, #4597 ) ) ;
#2394=VECTOR ( 'NONE', #9999, 1000.000000000000000 ) ;
#2400=CARTESIAN_POINT ( 'NONE',  ( 41.67500000054622689, 24.28113015263587116, 96.68563167572563088 ) ) ;
#2401=CARTESIAN_POINT ( 'NONE',  ( 24.37500000054622618, 13.07298590277314432, 88.54243821818161564 ) ) ;
#2403=CARTESIAN_POINT ( 'NONE',  ( 8.869784206589267583, 15.36130915976373501, 96.70605587419206017 ) ) ;
#2411=DIRECTION ( 'NONE',  ( -1.000000000000000000, 0.000000000000000000, 0.000000000000000000 ) ) ;
#2415=CARTESIAN_POINT ( 'NONE',  ( 31.17500000054621978, 26.19570976099943849, 86.29171490190961435 ) ) ;
#2417=CARTESIAN_POINT ( 'NONE',  ( 48.47500000054622404, 13.80429023900056684, 86.29171490190961435 ) ) ;
#2418=CARTESIAN_POINT ( 'NONE',  ( 34.37500000054622973, 12.34168156654572535, 90.79316153445363113 ) ) ;
#2419=CARTESIAN_POINT ( 'NONE',  ( 38.89999999999997726, 17.56310227825321135, 83.29316153445363113 ) ) ;
#2421=CARTESIAN_POINT ( 'NONE',  ( 47.27500000054622831, 27.65831843345427998, 90.79316153445363113 ) ) ;
#2423=CARTESIAN_POINT ( 'NONE',  ( 27.95000000109246585, 13.62011893735971135, 95.42841645007781892 ) ) ;
#2427=ORIENTED_EDGE ( 'NONE', *, *, #4592, .F. ) ;
#2428=EDGE_CURVE ( 'NONE', #6680, #8919, #8109, .T. ) ;
#2430=CARTESIAN_POINT ( 'NONE',  ( 10.00000000000000355, 20.00000000000000355, 109.9999999999999858 ) ) ;
#2431=CARTESIAN_POINT ( 'NONE',  ( -5.000000000000004441, 20.00000000000000000, 137.5000000000000000 ) ) ;
#2433=CYLINDRICAL_SURFACE ( 'NONE', #6562, 7.500000000000000000 ) ;
#2434=CARTESIAN_POINT ( 'NONE',  ( 24.27500000054622475, 12.34168156654572535, 90.79316153445363113 ) ) ;
#2435=CARTESIAN_POINT ( 'NONE',  ( 24.37500000054622262, 12.34168156654572535, 90.79316153445363113 ) ) ;
#2436=DIRECTION ( 'NONE',  ( 0.000000000000000000, 0.000000000000000000, 1.000000000000000000 ) ) ;
#2437=( BOUNDED_CURVE ( )  B_SPLINE_CURVE ( 2, ( #9695, #4808, #6766, #1816, #1943, #2006, #5703, #11464, #8487, #3716, #2836 ),
 .UNSPECIFIED., .F., .F. ) 
 B_SPLINE_CURVE_WITH_KNOTS ( ( 3, 2, 2, 2, 2, 3 ),
 ( 0.9333333333333333481, 0.9399999999999999467, 0.9466666666666666563, 0.9533333333333333659, 0.9599999999999999645, 0.9666666666666666741 ),
 .UNSPECIFIED. ) 
 CURVE ( )  GEOMETRIC_REPRESENTATION_ITEM ( )  RATIONAL_B_SPLINE_CURVE ( ( 1.000000000000000000, 0.9510565162951535312, 1.000000000000000000, 0.9510565162951535312, 1.000000000000000000, 0.9510565162951535312, 1.000000000000000000, 0.9510565162951535312, 1.000000000000000000, 0.9510565162951535312, 1.000000000000000000 ) ) 
 REPRESENTATION_ITEM ( '' )  );
#2439=ORIENTED_EDGE ( 'NONE', *, *, #2151, .F. ) ;
#2440=CARTESIAN_POINT ( 'NONE',  ( 45.35000000109246088, 26.37988106264029398, 95.42841645007781892 ) ) ;
#2442=DIRECTION ( 'NONE',  ( 1.000000000000000000, -0.000000000000000000, -0.000000000000000000 ) ) ;
#2451=DIRECTION ( 'NONE',  ( 1.000000000000000000, -0.000000000000000000, 0.000000000000000000 ) ) ;
#2456=ORIENTED_EDGE ( 'NONE', *, *, #4472, .T. ) ;
#2460=CARTESIAN_POINT ( 'NONE',  ( 44.57500000054622546, 13.80429023900056684, 86.29171490190961435 ) ) ;
#2461=CARTESIAN_POINT ( 'NONE',  ( 29.47500000054622404, 26.19570976099943849, 95.29460816699764791 ) ) ;
#2463=FACE_OUTER_BOUND ( 'NONE', #1916, .T. ) ;
#2467=ORIENTED_EDGE ( 'NONE', *, *, #8533, .F. ) ;
#2469=DIRECTION ( 'NONE',  ( 1.000000000000000000, -0.000000000000000000, -0.000000000000000000 ) ) ;
#2474=EDGE_CURVE ( 'NONE', #5241, #12263, #1951, .T. ) ;
#2475=CARTESIAN_POINT ( 'NONE',  ( 31.97500000054622760, 17.63344945572769973, 98.07665518445361386 ) ) ;
#2477=CARTESIAN_POINT ( 'NONE',  ( 45.87500000054622973, 17.63344945572769973, 98.07665518445361386 ) ) ;
#2478=CARTESIAN_POINT ( 'NONE',  ( 33.37500000054621552, 27.65831843345427998, 90.79316153445363113 ) ) ;
#2479=CARTESIAN_POINT ( 'NONE',  ( 35.89999999999998437, 22.43689772174679575, 98.29316153445363113 ) ) ;
#2481=CARTESIAN_POINT ( 'NONE',  ( 42.47500000054622404, 13.80429023900056684, 86.29171490190961435 ) ) ;
#2483=CARTESIAN_POINT ( 'NONE',  ( 27.75000000109246301, 17.56310227825320425, 98.29316153445363113 ) ) ;
#2489=CARTESIAN_POINT ( 'NONE',  ( 22.99999999999998934, 20.00000000000000355, 83.29316153445364534 ) ) ;
#2490=CARTESIAN_POINT ( 'NONE',  ( 27.49999999999999645, 20.00000000000000355, 170.0000119999999697 ) ) ;
#2494=CARTESIAN_POINT ( 'NONE',  ( 32.65000000109246514, 20.00000000000000355, 83.29316153445364534 ) ) ;
#2495=( BOUNDED_CURVE ( )  B_SPLINE_CURVE ( 3, ( #11374, #9166, #11311, #4521 ),
 .UNSPECIFIED., .F., .F. ) 
 B_SPLINE_CURVE_WITH_KNOTS ( ( 4, 4 ),
 ( 1.570796326794896558, 2.871659857756389655 ),
 .UNSPECIFIED. ) 
 CURVE ( )  GEOMETRIC_REPRESENTATION_ITEM ( )  RATIONAL_B_SPLINE_CURVE ( ( 1.000000000000000000, 0.8638816171694809753, 0.8638816171694809753, 1.000000000000000000 ) ) 
 REPRESENTATION_ITEM ( '' )  );
#2496=CARTESIAN_POINT ( 'NONE',  ( 25.77500000054622831, 20.00000000000000355, 98.07665518445361386 ) ) ;
#2497=CARTESIAN_POINT ( 'NONE',  ( 28.07500000054622546, 15.71886984736413417, 96.68563167572563088 ) ) ;
#2498=AXIS2_PLACEMENT_3D ( 'NONE', #7592, #12472, #2829 ) ;
#2499=DIRECTION ( 'NONE',  ( 1.000000000000000000, -0.000000000000000000, -0.000000000000000000 ) ) ;
#2500=EDGE_CURVE ( 'NONE', #2989, #315, #4579, .T. ) ;
#2502=ORIENTED_EDGE ( 'NONE', *, *, #1701, .F. ) ;
#2503=CARTESIAN_POINT ( 'NONE',  ( 44.25000000109246656, 12.86707612778636012, 88.47553407664152303 ) ) ;
#2506=CARTESIAN_POINT ( 'NONE',  ( 46.99999999999998579, 20.00000000000000355, 83.29316153445364534 ) ) ;
#2508=EDGE_CURVE ( 'NONE', #5989, #8756, #5481, .T. ) ;
#2513=EDGE_CURVE ( 'NONE', #6066, #5525, #10418, .T. ) ;
#2526=CARTESIAN_POINT ( 'NONE',  ( 38.07500000054622546, 15.71886984736413417, 96.68563167572563088 ) ) ;
#2527=CARTESIAN_POINT ( 'NONE',  ( 26.27500000054622475, 12.34168156654572357, 90.79316153445363113 ) ) ;
#2528=CARTESIAN_POINT ( 'NONE',  ( 6.732131639182266092, 12.60512992570006929, 92.06969329359783671 ) ) ;
#2532=DIRECTION ( 'NONE',  ( 1.000000000000000000, -0.000000000000000000, -0.000000000000000000 ) ) ;
#2533=ORIENTED_EDGE ( 'NONE', *, *, #10351, .F. ) ;
#2538=CARTESIAN_POINT ( 'NONE',  ( 30.07500000054622546, 15.71886984736413417, 96.68563167572563088 ) ) ;
#2540=AXIS2_PLACEMENT_3D ( 'NONE', #3055, #271, #6917 ) ;
#2541=CARTESIAN_POINT ( 'NONE',  ( 42.97500000054623115, 24.28113015263587471, 84.90069139318163138 ) ) ;
#2542=CARTESIAN_POINT ( 'NONE',  ( 34.09999999999998721, 17.56310227825320425, 98.29316153445363113 ) ) ;
#2544=CARTESIAN_POINT ( 'NONE',  ( 37.87500000054622262, 17.63344945572769973, 98.07665518445361386 ) ) ;
#2546=CARTESIAN_POINT ( 'NONE',  ( 45.57500000054622546, 24.28113015263587116, 96.68563167572563088 ) ) ;
#2547=CARTESIAN_POINT ( 'NONE',  ( 28.65000000109246514, 20.00000000000000355, 83.29316153445364534 ) ) ;
#2552=CARTESIAN_POINT ( 'NONE',  ( 48.65000000109246514, 20.00000000000000355, 83.29316153445364534 ) ) ;
#2553=CARTESIAN_POINT ( 'NONE',  ( -27.49999999999999645, 12.50000000000001066, 145.0000000000000000 ) ) ;
#2554=CARTESIAN_POINT ( 'NONE',  ( 25.99999999999998934, 20.00000000000000355, 98.29316153445363113 ) ) ;
#2556=CARTESIAN_POINT ( 'NONE',  ( 21.17500000054623044, 26.92701409722686634, 88.54243821818162985 ) ) ;
#2557=CARTESIAN_POINT ( 'NONE',  ( 23.57500000054622546, 26.19570976099943493, 95.29460816699764791 ) ) ;
#2559=CARTESIAN_POINT ( 'NONE',  ( 41.79999999999999005, 24.40838939219354842, 96.86078899226572503 ) ) ;
#2562=CARTESIAN_POINT ( 'NONE',  ( 40.15000000109245804, 12.11403331821300533, 90.79316153445363113 ) ) ;
#2565=CARTESIAN_POINT ( 'NONE',  ( -2.000000000000015543, 20.00000000000000355, 83.29316153445364534 ) ) ;
#2571=CARTESIAN_POINT ( 'NONE',  ( 20.37500000054622618, 13.07298590277314432, 88.54243821818161564 ) ) ;
#2572=EDGE_CURVE ( 'NONE', #2798, #12151, #964, .T. ) ;
#2573=LINE ( 'NONE', #9187, #5982 ) ;
#2578=CARTESIAN_POINT ( 'NONE',  ( 27.87500000054622618, 17.63344945572769973, 98.07665518445361386 ) ) ;
#2579=AXIS2_PLACEMENT_3D ( 'NONE', #10387, #3665, #5521 ) ;
#2584=VECTOR ( 'NONE', #6211, 1000.000000000000000 ) ;
#2585=CARTESIAN_POINT ( 'NONE',  ( -28.50000000000001066, 69.50000000000000000, 146.8533255156881978 ) ) ;
#2586=CARTESIAN_POINT ( 'NONE',  ( 39.37500000054622973, 26.92701409722686634, 93.04388485072563242 ) ) ;
#2587=CARTESIAN_POINT ( 'NONE',  ( 37.07500000054622546, 24.28113015263587471, 84.90069139318163138 ) ) ;
#2588=CARTESIAN_POINT ( 'NONE',  ( 29.87500000054622618, 17.63344945572769973, 98.07665518445361386 ) ) ;
#2589=CARTESIAN_POINT ( 'NONE',  ( 8.035382134961579936, 14.03808006457184199, 95.36761081598396572 ) ) ;
#2592=CYLINDRICAL_SURFACE ( 'NONE', #5060, 7.500000000000007105 ) ;
#2595=FACE_OUTER_BOUND ( 'NONE', #7906, .T. ) ;
#2597=CARTESIAN_POINT ( 'NONE',  ( -50.00000000000001421, 92.00000000000000000, 166.8533255156881694 ) ) ;
#2600=CARTESIAN_POINT ( 'NONE',  ( 29.87500000054622618, 20.00000000000000355, 98.07665518445361386 ) ) ;
#2601=CARTESIAN_POINT ( 'NONE',  ( 29.05000000109246727, 27.13292387221364876, 88.47553407664153724 ) ) ;
#2602=CARTESIAN_POINT ( 'NONE',  ( 44.07500000054623257, 13.80429023900056507, 95.29460816699764791 ) ) ;
#2603=VECTOR ( 'NONE', #4720, 1000.000000000000000 ) ;
#2604=CARTESIAN_POINT ( 'NONE',  ( 33.87500000054622262, 20.00000000000000355, 98.07665518445361386 ) ) ;
#2605=CARTESIAN_POINT ( 'NONE',  ( 31.39999999999998437, 27.13292387221364876, 88.47553407664153724 ) ) ;
#2606=CARTESIAN_POINT ( 'NONE',  ( -19.99999999999999645, 20.00000000000000355, 99.99999999999997158 ) ) ;
#2607=ADVANCED_FACE ( 'NONE', ( #5846 ), #8698, .F. ) ;
#2608=CARTESIAN_POINT ( 'NONE',  ( 41.37500000054622262, 26.92701409722686634, 93.04388485072563242 ) ) ;
#2610=CARTESIAN_POINT ( 'NONE',  ( 49.77500000054622831, 20.00000000000000355, 98.07665518445361386 ) ) ;
#2611=DIRECTION ( 'NONE',  ( -0.000000000000000000, -0.000000000000000000, 1.000000000000000000 ) ) ;
#2617=CARTESIAN_POINT ( 'NONE',  ( 41.85000000109246798, 15.59161060780645691, 96.86078899226572503 ) ) ;
#2618=CARTESIAN_POINT ( 'NONE',  ( 21.45000000109246230, 24.40838939219354842, 96.86078899226572503 ) ) ;
#2620=DIRECTION ( 'NONE',  ( 0.000000000000000000, 0.000000000000000000, -1.000000000000000000 ) ) ;
#2621=DIRECTION ( 'NONE',  ( -1.000000000000000000, 0.000000000000000000, 0.000000000000000000 ) ) ;
#2622=CARTESIAN_POINT ( 'NONE',  ( 21.77500000054622831, 20.00000000000000355, 98.07665518445361386 ) ) ;
#2623=CARTESIAN_POINT ( 'NONE',  ( 22.77500000054622475, 17.63344945572770328, 83.50966788445364841 ) ) ;
#2625=VECTOR ( 'NONE', #6308, 1000.000000000000000 ) ;
#2627=ORIENTED_EDGE ( 'NONE', *, *, #952, .F. ) ;
#2628=CARTESIAN_POINT ( 'NONE',  ( 35.55000000109245661, 22.43689772174679575, 98.29316153445363113 ) ) ;
#2631=CARTESIAN_POINT ( 'NONE',  ( 47.99999999999998579, 20.00000000000000355, 98.29316153445363113 ) ) ;
#2633=ORIENTED_EDGE ( 'NONE', *, *, #5487, .F. ) ;
#2637=DIRECTION ( 'NONE',  ( 1.000000000000000000, -0.000000000000000000, -0.000000000000000000 ) ) ;
#2638=ADVANCED_FACE ( 'NONE', ( #7686 ), #3996, .F. ) ;
#2641=CIRCLE ( 'NONE', #7716, 7.500000000000000000 ) ;
#2642=DIRECTION ( 'NONE',  ( 1.000000000000000000, -0.000000000000000000, -0.000000000000000000 ) ) ;
#2643=CARTESIAN_POINT ( 'NONE',  ( 47.95000000109246230, 13.62011893735970958, 95.42841645007781892 ) ) ;
#2644=CARTESIAN_POINT ( 'NONE',  ( 47.47500000054622404, 26.92701409722686634, 93.04388485072563242 ) ) ;
#2649=DIRECTION ( 'NONE',  ( 1.000000000000000000, 0.000000000000000000, 0.000000000000000000 ) ) ;
#2653=CARTESIAN_POINT ( 'NONE',  ( 35.27500000054622831, 27.65831843345427998, 90.79316153445363113 ) ) ;
#2654=CARTESIAN_POINT ( 'NONE',  ( 35.07500000054622546, 24.28113015263587471, 84.90069139318163138 ) ) ;
#2655=CARTESIAN_POINT ( 'NONE',  ( 20.67500000054622689, 17.63344945572770328, 83.50966788445364841 ) ) ;
#2656=DIRECTION ( 'NONE',  ( 0.000000000000000000, 0.000000000000000000, 1.000000000000000000 ) ) ;
#2659=LINE ( 'NONE', #1758, #5470 ) ;
#2661=VECTOR ( 'NONE', #140, 1000.000000000000000 ) ;
#2662=DIRECTION ( 'NONE',  ( 1.000000000000000000, 0.000000000000000000, 0.000000000000000000 ) ) ;
#2666=CARTESIAN_POINT ( 'NONE',  ( 24.87500000054622262, 20.00000000000000355, 83.50966788445364841 ) ) ;
#2668=CARTESIAN_POINT ( 'NONE',  ( 43.57500000054623257, 24.28113015263587116, 96.68563167572563088 ) ) ;
#2669=CARTESIAN_POINT ( 'NONE',  ( 26.77500000054622475, 17.63344945572770328, 83.50966788445364841 ) ) ;
#2670=CARTESIAN_POINT ( 'NONE',  ( 27.09999999999999076, 22.43689772174679575, 83.29316153445363113 ) ) ;
#2672=CARTESIAN_POINT ( 'NONE',  ( 39.57500000054622546, 24.28113015263587116, 96.68563167572563088 ) ) ;
#2674=CARTESIAN_POINT ( 'NONE',  ( 47.37500000054622973, 26.92701409722686634, 93.04388485072563242 ) ) ;
#2676=ORIENTED_EDGE ( 'NONE', *, *, #5792, .T. ) ;
#2681=CARTESIAN_POINT ( 'NONE',  ( -20.27158385259952667, 18.00000000000000355, 152.2284161474004520 ) ) ;
#2682=CARTESIAN_POINT ( 'NONE',  ( 43.47500000054622404, 26.92701409722686634, 93.04388485072563242 ) ) ;
#2684=CARTESIAN_POINT ( 'NONE',  ( 25.07500000054623257, 26.19570976099943493, 86.29171490190961435 ) ) ;
#2685=CARTESIAN_POINT ( 'NONE',  ( 48.29999999999999005, 13.62011893735971135, 95.42841645007781892 ) ) ;
#2686=DIRECTION ( 'NONE',  ( 1.000000000000000000, -0.000000000000000000, -0.000000000000000000 ) ) ;
#2688=ORIENTED_EDGE ( 'NONE', *, *, #1952, .T. ) ;
#2690=VECTOR ( 'NONE', #6588, 1000.000000000000000 ) ;
#2691=CARTESIAN_POINT ( 'NONE',  ( 38.55000000109247082, 17.56310227825321135, 83.29316153445363113 ) ) ;
#2692=LINE ( 'NONE', #4532, #1817 ) ;
#2694=FACE_BOUND ( 'NONE', #8794, .T. ) ;
#2702=ORIENTED_EDGE ( 'NONE', *, *, #6023, .F. ) ;
#2704=CARTESIAN_POINT ( 'NONE',  ( 47.85000000109246088, 15.59161060780645691, 96.86078899226572503 ) ) ;
#2705=CARTESIAN_POINT ( 'NONE',  ( 49.17500000054622689, 26.19570976099943493, 86.29171490190961435 ) ) ;
#2708=CARTESIAN_POINT ( 'NONE',  ( 36.65000000109245804, 20.00000000000000355, 83.29316153445364534 ) ) ;
#2714=CARTESIAN_POINT ( 'NONE',  ( 36.27500000054622120, 13.07298590277314254, 93.04388485072563242 ) ) ;
#2717=CARTESIAN_POINT ( 'NONE',  ( 21.17500000054623044, 26.92701409722686634, 88.54243821818162985 ) ) ;
#2722=EDGE_CURVE ( 'NONE', #8756, #3198, #70, .T. ) ;
#2725=CARTESIAN_POINT ( 'NONE',  ( -50.00000000000001421, 22.00000000000000000, 188.4007504869563263 ) ) ;
#2729=CARTESIAN_POINT ( 'NONE',  ( 24.57500000054622191, 13.80429023900056684, 86.29171490190961435 ) ) ;
#2730=CARTESIAN_POINT ( 'NONE',  ( 36.29999999999997584, 13.62011893735970958, 95.42841645007781892 ) ) ;
#2731=CARTESIAN_POINT ( 'NONE',  ( 37.87500000054622262, 17.63344945572769973, 98.07665518445361386 ) ) ;
#2732=CARTESIAN_POINT ( 'NONE',  ( 26.07500000054622546, 15.71886984736413417, 96.68563167572563088 ) ) ;
#2733=CARTESIAN_POINT ( 'NONE',  ( 28.59999999999998721, 12.86707612778636012, 88.47553407664152303 ) ) ;
#2734=CARTESIAN_POINT ( 'NONE',  ( 34.99999999999999289, 20.00000000000000355, 83.29316153445364534 ) ) ;
#2735=CARTESIAN_POINT ( 'NONE',  ( 42.67500000054623399, 17.63344945572770328, 83.50966788445364841 ) ) ;
#2738=ADVANCED_FACE ( 'NONE', ( #10094 ), #5211, .F. ) ;
#2739=CARTESIAN_POINT ( 'NONE',  ( 46.87500000054622262, 22.36655054427230382, 83.50966788445364841 ) ) ;
#2740=DIRECTION ( 'NONE',  ( -1.000000000000000000, -0.000000000000000000, -0.000000000000000000 ) ) ;
#2741=VERTEX_POINT ( 'NONE', #11102 ) ;
#2744=DIRECTION ( 'NONE',  ( 0.000000000000000000, 0.000000000000000000, 1.000000000000000000 ) ) ;
#2747=CARTESIAN_POINT ( 'NONE',  ( 42.47500000054623115, 13.07298590277314432, 88.54243821818161564 ) ) ;
#2748=LINE ( 'NONE', #7442, #7583 ) ;
#2749=CARTESIAN_POINT ( 'NONE',  ( 48.79999999999999005, 15.59161060780646046, 84.72553407664153724 ) ) ;
#2754=CARTESIAN_POINT ( 'NONE',  ( 37.65000000109246514, 20.00000000000000355, 98.29316153445363113 ) ) ;
#2756=DIRECTION ( 'NONE',  ( 0.000000000000000000, 0.000000000000000000, -1.000000000000000000 ) ) ;
#2757=ORIENTED_EDGE ( 'NONE', *, *, #9053, .T. ) ;
#2760=LINE ( 'NONE', #11331, #10599 ) ;
#2763=ORIENTED_EDGE ( 'NONE', *, *, #1134, .T. ) ;
#2766=CARTESIAN_POINT ( 'NONE',  ( 22.17500000054622689, 13.07298590277314254, 93.04388485072563242 ) ) ;
#2771=AXIS2_PLACEMENT_3D ( 'NONE', #8363, #12295, #2649 ) ;
#2776=CARTESIAN_POINT ( 'NONE',  ( 22.97500000054622760, 24.28113015263587471, 84.90069139318163138 ) ) ;
#2780=CARTESIAN_POINT ( 'NONE',  ( 26.35000000109246443, 13.62011893735970958, 86.15790661882942914 ) ) ;
#2784=EDGE_CURVE ( 'NONE', #136, #1411, #2845, .T. ) ;
#2787=CARTESIAN_POINT ( 'NONE',  ( 28.47500000054622404, 13.07298590277314432, 88.54243821818161564 ) ) ;
#2788=CARTESIAN_POINT ( 'NONE',  ( 36.09999999999998721, 17.56310227825319004, 98.29316153445361692 ) ) ;
#2789=CARTESIAN_POINT ( 'NONE',  ( 39.37500000054622973, 26.92701409722686634, 93.04388485072563242 ) ) ;
#2790=VECTOR ( 'NONE', #6247, 1000.000000000000000 ) ;
#2791=CARTESIAN_POINT ( 'NONE',  ( 29.57500000054621836, 26.19570976099943493, 95.29460816699764791 ) ) ;
#2792=CARTESIAN_POINT ( 'NONE',  ( 26.69999999999998508, 13.62011893735971135, 86.15790661882942914 ) ) ;
#2793=CARTESIAN_POINT ( 'NONE',  ( 30.99999999999998934, 20.00000000000000355, 83.29316153445364534 ) ) ;
#2794=CARTESIAN_POINT ( 'NONE',  ( 35.07500000054623257, 26.19570976099943493, 86.29171490190961435 ) ) ;
#2796=CARTESIAN_POINT ( 'NONE',  ( 21.35000000109246443, 26.37988106264029398, 95.42841645007781892 ) ) ;
#2798=VERTEX_POINT ( 'NONE', #9081 ) ;
#2802=DIRECTION ( 'NONE',  ( 1.000000000000000000, -0.000000000000000000, -0.000000000000000000 ) ) ;
#2804=CARTESIAN_POINT ( 'NONE',  ( 41.57500000054622546, 26.19570976099943849, 95.29460816699764791 ) ) ;
#2808=CARTESIAN_POINT ( 'NONE',  ( 45.87500000054622973, 20.00000000000000355, 98.07665518445361386 ) ) ;
#2809=CARTESIAN_POINT ( 'NONE',  ( 46.99999999999998579, 20.00000000000000355, 83.29316153445364534 ) ) ;
#2811=CARTESIAN_POINT ( 'NONE',  ( 39.05000000109247082, 27.13292387221364876, 88.47553407664153724 ) ) ;
#2812=AXIS2_PLACEMENT_3D ( 'NONE', #1217, #6030, #3048 ) ;
#2814=CARTESIAN_POINT ( 'NONE',  ( 39.75000000109247367, 17.56310227825320425, 98.29316153445363113 ) ) ;
#2817=DIRECTION ( 'NONE',  ( -1.000000000000000000, 0.000000000000000000, 0.000000000000000000 ) ) ;
#2818=ADVANCED_FACE ( 'NONE', ( #2353 ), #514, .F. ) ;
#2822=AXIS2_PLACEMENT_3D ( 'NONE', #8251, #5463, #5397 ) ;
#2829=DIRECTION ( 'NONE',  ( 0.000000000000000000, -0.000000000000000000, 1.000000000000000000 ) ) ;
#2830=CARTESIAN_POINT ( 'NONE',  ( 23.27500000054622120, 27.65831843345427998, 90.79316153445363113 ) ) ;
#2832=DIRECTION ( 'NONE',  ( -1.000000000000000000, 0.000000000000000000, 0.000000000000000000 ) ) ;
#2836=CARTESIAN_POINT ( 'NONE',  ( 20.99999999999998579, 20.00000000000000355, 83.29316153445364534 ) ) ;
#2837=EDGE_CURVE ( 'NONE', #4281, #11966, #624, .T. ) ;
#2840=CARTESIAN_POINT ( 'NONE',  ( 21.27500000054622475, 27.65831843345427998, 90.79316153445363113 ) ) ;
#2844=EDGE_CURVE ( 'NONE', #7750, #8571, #8843, .T. ) ;
#2845=( BOUNDED_CURVE ( )  B_SPLINE_CURVE ( 2, ( #451, #5087, #8001, #9147, #7104, #8192, #6160, #1278, #7165, #11873, #11043 ),
 .UNSPECIFIED., .F., .F. ) 
 B_SPLINE_CURVE_WITH_KNOTS ( ( 3, 2, 2, 2, 2, 3 ),
 ( 0.5333333333333333259, 0.5400000000000000355, 0.5466666666666666341, 0.5533333333333333437, 0.5600000000000000533, 0.5666666666666666519 ),
 .UNSPECIFIED. ) 
 CURVE ( )  GEOMETRIC_REPRESENTATION_ITEM ( )  RATIONAL_B_SPLINE_CURVE ( ( 1.000000000000000000, 0.9510565162951535312, 1.000000000000000000, 0.9510565162951535312, 1.000000000000000000, 0.9510565162951535312, 1.000000000000000000, 0.9510565162951535312, 1.000000000000000000, 0.9510565162951535312, 1.000000000000000000 ) ) 
 REPRESENTATION_ITEM ( '' )  );
#2848=VERTEX_POINT ( 'NONE', #9970 ) ;
#2850=EDGE_CURVE ( 'NONE', #2251, #5929, #3240, .T. ) ;
#2851=CARTESIAN_POINT ( 'NONE',  ( 25.27500000054622475, 26.92701409722686634, 88.54243821818162985 ) ) ;
#2852=CARTESIAN_POINT ( 'NONE',  ( 48.07500000054622546, 15.71886984736413417, 96.68563167572563088 ) ) ;
#2853=CARTESIAN_POINT ( 'NONE',  ( 41.57500000054623257, 24.28113015263587116, 96.68563167572563088 ) ) ;
#2854=CARTESIAN_POINT ( 'NONE',  ( 27.57500000054622191, 26.19570976099943493, 95.29460816699764791 ) ) ;
#2855=CARTESIAN_POINT ( 'NONE',  ( 32.39999999999998437, 12.86707612778636012, 93.11078899226572503 ) ) ;
#2858=CARTESIAN_POINT ( 'NONE',  ( 49.99999999999998579, 40.00000000000000000, 169.9999999999999716 ) ) ;
#2859=CARTESIAN_POINT ( 'NONE',  ( 31.07500000054622191, 26.19570976099943493, 86.29171490190961435 ) ) ;
#2860=ORIENTED_EDGE ( 'NONE', *, *, #12102, .F. ) ;
#2862=ORIENTED_EDGE ( 'NONE', *, *, #4474, .T. ) ;
#2867=CARTESIAN_POINT ( 'NONE',  ( 31.99999999999998579, 20.00000000000000355, 98.29316153445363113 ) ) ;
#2869=CARTESIAN_POINT ( 'NONE',  ( 45.87500000054622973, 20.00000000000000355, 98.07665518445361386 ) ) ;
#2870=CARTESIAN_POINT ( 'NONE',  ( 20.09999999999998721, 17.56310227825320425, 98.29316153445363113 ) ) ;
#2871=DIRECTION ( 'NONE',  ( -1.000000000000000000, 0.000000000000000000, -0.000000000000000000 ) ) ;
#2872=CARTESIAN_POINT ( 'NONE',  ( 44.87500000054622973, 20.00000000000000355, 83.50966788445364841 ) ) ;
#2873=CARTESIAN_POINT ( 'NONE',  ( 45.99999999999998579, 20.00000000000000355, 98.29316153445363113 ) ) ;
#2874=CARTESIAN_POINT ( 'NONE',  ( 39.89999999999999147, 22.43689772174681707, 98.29316153445361692 ) ) ;
#2875=CARTESIAN_POINT ( 'NONE',  ( 44.79999999999998295, 15.59161060780646046, 84.72553407664153724 ) ) ;
#2877=CARTESIAN_POINT ( 'NONE',  ( 29.15000000109246159, 27.88596668178699645, 90.79316153445363113 ) ) ;
#2878=DIRECTION ( 'NONE',  ( 0.000000000000000000, 0.000000000000000000, 1.000000000000000000 ) ) ;
#2880=LINE ( 'NONE', #790, #2603 ) ;
#2881=EDGE_CURVE ( 'NONE', #11262, #9504, #2252, .T. ) ;
#2885=DIRECTION ( 'NONE',  ( 1.000000000000000000, -0.000000000000000000, -0.000000000000000000 ) ) ;
#2886=ADVANCED_FACE ( 'NONE', ( #2595 ), #7610, .F. ) ;
#2887=CARTESIAN_POINT ( 'NONE',  ( 36.97500000054623115, 24.28113015263587471, 84.90069139318163138 ) ) ;
#2890=CARTESIAN_POINT ( 'NONE',  ( 34.55000000109246372, 17.56310227825320425, 83.29316153445363113 ) ) ;
#2891=ORIENTED_EDGE ( 'NONE', *, *, #4626, .F. ) ;
#2893=PLANE ( 'NONE',  #2498 ) ;
#2894=CARTESIAN_POINT ( 'NONE',  ( 48.87500000054622262, 20.00000000000000355, 83.50966788445364841 ) ) ;
#2895=VERTEX_POINT ( 'NONE', #6585 ) ;
#2898=CARTESIAN_POINT ( 'NONE',  ( 22.99999999999998934, 20.00000000000000355, 83.29316153445364534 ) ) ;
#2900=ORIENTED_EDGE ( 'NONE', *, *, #2322, .F. ) ;
#2903=CARTESIAN_POINT ( 'NONE',  ( -27.49999999999999645, 27.49999999999999645, 145.0000000000000000 ) ) ;
#2904=CARTESIAN_POINT ( 'NONE',  ( 22.47500000054622760, 13.80429023900056684, 86.29171490190961435 ) ) ;
#2909=CARTESIAN_POINT ( 'NONE',  ( 26.15000000109246159, 12.11403331821300533, 90.79316153445363113 ) ) ;
#2912=CARTESIAN_POINT ( 'NONE',  ( 37.45000000109246230, 24.40838939219354842, 96.86078899226572503 ) ) ;
#2913=VECTOR ( 'NONE', #11897, 1000.000000000000000 ) ;
#2915=CARTESIAN_POINT ( 'NONE',  ( 47.57500000054621125, 26.19570976099943493, 95.29460816699764791 ) ) ;
#2916=CARTESIAN_POINT ( 'NONE',  ( 38.27500000054623541, 12.34168156654572357, 90.79316153445363113 ) ) ;
#2917=( BOUNDED_CURVE ( )  B_SPLINE_CURVE ( 2, ( #5366, #12150, #8032, #6187, #1311, #3270, #5180, #3390, #359, #7133, #1436 ),
 .UNSPECIFIED., .F., .F. ) 
 B_SPLINE_CURVE_WITH_KNOTS ( ( 3, 2, 2, 2, 2, 3 ),
 ( 0.9000000000000000222, 0.9066666666666666208, 0.9133333333333333304, 0.9200000000000000400, 0.9266666666666666385, 0.9333333333333333481 ),
 .UNSPECIFIED. ) 
 CURVE ( )  GEOMETRIC_REPRESENTATION_ITEM ( )  RATIONAL_B_SPLINE_CURVE ( ( 1.000000000000000000, 0.9510565162951535312, 1.000000000000000000, 0.9510565162951535312, 1.000000000000000000, 0.9510565162951535312, 1.000000000000000000, 0.9510565162951535312, 1.000000000000000000, 0.9510565162951535312, 1.000000000000000000 ) ) 
 REPRESENTATION_ITEM ( '' )  );
#2918=CARTESIAN_POINT ( 'NONE',  ( 25.07500000054622191, 24.28113015263587471, 84.90069139318163138 ) ) ;
#2919=CARTESIAN_POINT ( 'NONE',  ( 20.29999999999998650, 13.62011893735971135, 95.42841645007781892 ) ) ;
#2920=CARTESIAN_POINT ( 'NONE',  ( 30.29999999999998295, 13.62011893735970958, 95.42841645007781892 ) ) ;
#2921=CARTESIAN_POINT ( 'NONE',  ( 33.47500000054623115, 26.19570976099943493, 95.29460816699764791 ) ) ;
#2929=( LENGTH_UNIT ( ) NAMED_UNIT ( * ) SI_UNIT ( .MILLI., .METRE. ) );
#2930=CARTESIAN_POINT ( 'NONE',  ( 32.29999999999999005, 13.62011893735970958, 95.42841645007781892 ) ) ;
#2932=CARTESIAN_POINT ( 'NONE',  ( 44.37500000054622262, 12.34168156654572357, 90.79316153445363113 ) ) ;
#2934=CARTESIAN_POINT ( 'NONE',  ( 42.79999999999999005, 15.59161060780646046, 84.72553407664153724 ) ) ;
#2936=CARTESIAN_POINT ( 'NONE',  ( 40.79999999999999005, 15.59161060780646046, 84.72553407664153724 ) ) ;
#2940=CARTESIAN_POINT ( 'NONE',  ( 28.55000000109246372, 17.56310227825321135, 83.29316153445363113 ) ) ;
#2942=ORIENTED_EDGE ( 'NONE', *, *, #4970, .F. ) ;
#2945=FACE_OUTER_BOUND ( 'NONE', #11874, .T. ) ;
#2951=CARTESIAN_POINT ( 'NONE',  ( 34.07500000054622546, 13.80429023900056507, 95.29460816699764791 ) ) ;
#2952=CARTESIAN_POINT ( 'NONE',  ( 39.47500000054622404, 26.92701409722686634, 93.04388485072563242 ) ) ;
#2953=VECTOR ( 'NONE', #10374, 1000.000000000000000 ) ;
#2954=CARTESIAN_POINT ( 'NONE',  ( 34.85000000109246798, 24.40838939219355197, 84.72553407664153724 ) ) ;
#2955=CARTESIAN_POINT ( 'NONE',  ( 43.95000000109245519, 13.62011893735970958, 95.42841645007781892 ) ) ;
#2960=ORIENTED_EDGE ( 'NONE', *, *, #7602, .T. ) ;
#2962=EDGE_LOOP ( 'NONE', ( #6347, #7972, #3483, #9733 ) ) ;
#2963=EDGE_CURVE ( 'NONE', #949, #10590, #816, .T. ) ;
#2964=ORIENTED_EDGE ( 'NONE', *, *, #11892, .F. ) ;
#2966=( BOUNDED_CURVE ( )  B_SPLINE_CURVE ( 2, ( #3060, #2102, #5979, #9853, #1168, #8896, #702, #5344, #9340, #1652, #5283, #9399, #12250, #2417, #4570, #8442, #6294, #8199, #3611, #5406, #643, #4506, #12312, #11112, #10275, #6412, #1592, #460, #10165, #5474, #7427, #8382, #7489, #12069, #11230, #11360, #10335, #10103, #3369, #2477, #6352, #9215, #1471, #10220, #581, #3491, #7239, #5534, #521, #11174, #4382, #8259, #4322, #9277, #11297, #4447, #12129, #2602, #8324, #6473, #7299, #3437, #2668, #3553, #1417, #12191, #1533, #7362, #2541, #9154, #5592, #5652, #3734, #10458, #10520, #7741, #889, #11544, #957, #4759, #7616, #3799, #2853, #11479, #5838, #4825, #8625, #4887, #12375, #1833, #6651, #12496, #7679, #5716, #6716, #3865, #3929, #9710, #9463, #3675, #8691, #7553, #1960, #9525, #2789, #761, #5777, #10584, #1, #9583, #6530, #1895, #11676, #9650, #11609, #2916, #11422, #7804, #6780, #2731, #6589, #4632, #64, #10647, #1026, #8748, #1768, #10399, #8502, #1710, #823, #4693, #8566, #12437, #7995, #4052, #11865, #4248, #3043, #3172, #9838, #2982, #4948, #7931, #11795, #8120, #2086, #7035, #4117, #10909, #8060, #2224, #3102, #6847, #2155, #10710, #10976, #2021, #6093, #10841, #383, #5903, #1272, #5206, #9965, #6906, #3234, #5144, #9011, #6027, #7867, #5962, #195, #5013, #9773, #1150, #6972, #10772, #9900, #4185, #1214, #7095, #10028, #1083, #6154, #259, #322, #5080, #2284, #11927, #8948, #1337, #8812, #9075, #131, #3990, #11738, #8877, #565, #2588, #7345, #6460, #12237, #2461, #3418, #3355, #10321, #8184, #7412, #7286, #1638, #11282, #4556, #11216, #6337, #5457, #10205, #11156, #4371, #1516, #4428, #11035, #1579, #5519, #3539, #5393, #9265, #7224, #9386, #12055, #689, #8308, #11990, #3294, #7158, #2527, #12176, #9326, #3479, #6398, #8247, #628, #2345, #6214, #10087, #5266, #10263, #444, #4493, #8367, #1400, #9138, #4306, #11095, #2401, #6278, #10149, #1461, #5329, #9200, #509, #12115, #9448, #5826, #5765, #1697, #5578, #10444, #2776, #1754, #11405, #3663, #7664, #2904, #751, #8613, #4745, #12482, #11349, #8490, #3787, #9511, #11530, #9697, #12362, #2840, #2717, #1884, #6704, #4813, #10385, #2655, #7538, #6580, #4683, #11467, #1819, #4616, #8678, #5638, #811 ),
 .UNSPECIFIED., .F., .F. ) 
 B_SPLINE_CURVE_WITH_KNOTS ( ( 3, 2, 2, 2, 2, 2, 2, 2, 2, 2, 2, 2, 2, 2, 2, 2, 2, 2, 2, 2, 2, 2, 2, 2, 2, 2, 2, 2, 2, 2, 2, 2, 2, 2, 2, 2, 2, 2, 2, 2, 2, 2, 2, 2, 2, 2, 2, 2, 2, 2, 2, 2, 2, 2, 2, 2, 2, 2, 2, 2, 2, 2, 2, 2, 2, 2, 2, 2, 2, 2, 2, 2, 2, 2, 2, 2, 2, 2, 2, 2, 2, 2, 2, 2, 2, 2, 2, 2, 2, 2, 2, 2, 2, 2, 2, 2, 2, 2, 2, 2, 2, 2, 2, 2, 2, 2, 2, 2, 2, 2, 2, 2, 2, 2, 2, 2, 2, 2, 2, 2, 2, 2, 2, 2, 2, 2, 2, 2, 2, 2, 2, 2, 2, 2, 2, 2, 2, 2, 2, 2, 2, 2, 2, 2, 2, 2, 2, 2, 2, 2, 3 ),
 ( 0.000000000000000000, 0.006666666666666667095, 0.01333333333333333419, 0.02000000000000000042, 0.02666666666666666838, 0.03333333333333333287, 0.04000000000000000083, 0.04666666666666666879, 0.05333333333333333676, 0.05999999999999999778, 0.06666666666666666574, 0.07333333333333333370, 0.08000000000000000167, 0.08666666666666666963, 0.09333333333333333759, 0.1000000000000000056, 0.1066666666666666735, 0.1133333333333333276, 0.1199999999999999956, 0.1266666666666666774, 0.1333333333333333315, 0.1400000000000000133, 0.1466666666666666674, 0.1533333333333333215, 0.1600000000000000033, 0.1666666666666666574, 0.1733333333333333393, 0.1799999999999999933, 0.1866666666666666752, 0.1933333333333333293, 0.2000000000000000111, 0.2066666666666666652, 0.2133333333333333470, 0.2200000000000000011, 0.2266666666666666552, 0.2333333333333333370, 0.2399999999999999911, 0.2466666666666666730, 0.2533333333333333548, 0.2600000000000000089, 0.2666666666666666630, 0.2733333333333333171, 0.2800000000000000266, 0.2866666666666666807, 0.2933333333333333348, 0.2999999999999999889, 0.3066666666666666430, 0.3133333333333333526, 0.3200000000000000067, 0.3266666666666666607, 0.3333333333333333148, 0.3400000000000000244, 0.3466666666666666785, 0.3533333333333333326, 0.3599999999999999867, 0.3666666666666666408, 0.3733333333333333504, 0.3800000000000000044, 0.3866666666666666585, 0.3933333333333333126, 0.4000000000000000222, 0.4066666666666666763, 0.4133333333333333304, 0.4199999999999999845, 0.4266666666666666941, 0.4333333333333333481, 0.4400000000000000022, 0.4466666666666666563, 0.4533333333333333104, 0.4600000000000000200, 0.4666666666666666741, 0.4733333333333333282, 0.4799999999999999822, 0.4866666666666666918, 0.4933333333333333459, 0.5000000000000000000, 0.5066666666666667096, 0.5133333333333333082, 0.5200000000000000178, 0.5266666666666666163, 0.5333333333333333259, 0.5400000000000000355, 0.5466666666666666341, 0.5533333333333333437, 0.5600000000000000533, 0.5666666666666666519, 0.5733333333333333615, 0.5799999999999999600, 0.5866666666666666696, 0.5933333333333333792, 0.5999999999999999778, 0.6066666666666666874, 0.6133333333333332860, 0.6199999999999999956, 0.6266666666666667052, 0.6333333333333333037, 0.6400000000000000133, 0.6466666666666666119, 0.6533333333333333215, 0.6600000000000000311, 0.6666666666666666297, 0.6733333333333333393, 0.6800000000000000488, 0.6866666666666666474, 0.6933333333333333570, 0.6999999999999999556, 0.7066666666666666652, 0.7133333333333333748, 0.7199999999999999734, 0.7266666666666666829, 0.7333333333333332815, 0.7399999999999999911, 0.7466666666666667007, 0.7533333333333332993, 0.7600000000000000089, 0.7666666666666667185, 0.7733333333333333171, 0.7800000000000000266, 0.7866666666666666252, 0.7933333333333333348, 0.8000000000000000444, 0.8066666666666666430, 0.8133333333333333526, 0.8199999999999999512, 0.8266666666666666607, 0.8333333333333333703, 0.8399999999999999689, 0.8466666666666666785, 0.8533333333333333881, 0.8599999999999999867, 0.8666666666666666963, 0.8733333333333332948, 0.8800000000000000044, 0.8866666666666667140, 0.8933333333333333126, 0.9000000000000000222, 0.9066666666666666208, 0.9133333333333333304, 0.9200000000000000400, 0.9266666666666666385, 0.9333333333333333481, 0.9399999999999999467, 0.9466666666666666563, 0.9533333333333333659, 0.9599999999999999645, 0.9666666666666666741, 0.9733333333333333837, 0.9799999999999999822, 0.9866666666666666918, 0.9933333333333332904, 1.000000000000000000 ),
 .UNSPECIFIED. ) 
 CURVE ( )  GEOMETRIC_REPRESENTATION_ITEM ( )  RATIONAL_B_SPLINE_CURVE ( ( 1.000000000000000000, 0.9510565162951535312, 1.000000000000000000, 0.9510565162951535312, 1.000000000000000000, 0.9510565162951535312, 1.000000000000000000, 0.9510565162951535312, 1.000000000000000000, 0.9510565162951535312, 1.000000000000000000, 0.9510565162951535312, 1.000000000000000000, 0.9510565162951535312, 1.000000000000000000, 0.9510565162951535312, 1.000000000000000000, 0.9510565162951535312, 1.000000000000000000, 0.9510565162951535312, 1.000000000000000000, 0.9510565162951535312, 1.000000000000000000, 0.9510565162951535312, 1.000000000000000000, 0.9510565162951535312, 1.000000000000000000, 0.9510565162951535312, 1.000000000000000000, 0.9510565162951535312, 1.000000000000000000, 0.9510565162951535312, 1.000000000000000000, 0.9510565162951535312, 1.000000000000000000, 0.9510565162951535312, 1.000000000000000000, 0.9510565162951535312, 1.000000000000000000, 0.9510565162951535312, 1.000000000000000000, 0.9510565162951535312, 1.000000000000000000, 0.9510565162951535312, 1.000000000000000000, 0.9510565162951535312, 1.000000000000000000, 0.9510565162951535312, 1.000000000000000000, 0.9510565162951535312, 1.000000000000000000, 0.9510565162951535312, 1.000000000000000000, 0.9510565162951535312, 1.000000000000000000, 0.9510565162951535312, 1.000000000000000000, 0.9510565162951535312, 1.000000000000000000, 0.9510565162951535312, 1.000000000000000000, 0.9510565162951535312, 1.000000000000000000, 0.9510565162951535312, 1.000000000000000000, 0.9510565162951535312, 1.000000000000000000, 0.9510565162951535312, 1.000000000000000000, 0.9510565162951535312, 1.000000000000000000, 0.9510565162951535312, 1.000000000000000000, 0.9510565162951535312, 1.000000000000000000, 0.9510565162951535312, 1.000000000000000000, 0.9510565162951535312, 1.000000000000000000, 0.9510565162951535312, 1.000000000000000000, 0.9510565162951535312, 1.000000000000000000, 0.9510565162951535312, 1.000000000000000000, 0.9510565162951535312, 1.000000000000000000, 0.9510565162951535312, 1.000000000000000000, 0.9510565162951535312, 1.000000000000000000, 0.9510565162951535312, 1.000000000000000000, 0.9510565162951535312, 1.000000000000000000, 0.9510565162951535312, 1.000000000000000000, 0.9510565162951535312, 1.000000000000000000, 0.9510565162951535312, 1.000000000000000000, 0.9510565162951535312, 1.000000000000000000, 0.9510565162951535312, 1.000000000000000000, 0.9510565162951535312, 1.000000000000000000, 0.9510565162951535312, 1.000000000000000000, 0.9510565162951535312, 1.000000000000000000, 0.9510565162951535312, 1.000000000000000000, 0.9510565162951535312, 1.000000000000000000, 0.9510565162951535312, 1.000000000000000000, 0.9510565162951535312, 1.000000000000000000, 0.9510565162951535312, 1.000000000000000000, 0.9510565162951535312, 1.000000000000000000, 0.9510565162951535312, 1.000000000000000000, 0.9510565162951535312, 1.000000000000000000, 0.9510565162951535312, 1.000000000000000000, 0.9510565162951535312, 1.000000000000000000, 0.9510565162951535312, 1.000000000000000000, 0.9510565162951535312, 1.000000000000000000, 0.9510565162951535312, 1.000000000000000000, 0.9510565162951535312, 1.000000000000000000, 0.9510565162951535312, 1.000000000000000000, 0.9510565162951535312, 1.000000000000000000, 0.9510565162951535312, 1.000000000000000000, 0.9510565162951535312, 1.000000000000000000, 0.9510565162951535312, 1.000000000000000000, 0.9510565162951535312, 1.000000000000000000, 0.9510565162951535312, 1.000000000000000000, 0.9510565162951535312, 1.000000000000000000, 0.9510565162951535312, 1.000000000000000000, 0.9510565162951535312, 1.000000000000000000, 0.9510565162951535312, 1.000000000000000000, 0.9510565162951535312, 1.000000000000000000, 0.9510565162951535312, 1.000000000000000000, 0.9510565162951535312, 1.000000000000000000, 0.9510565162951535312, 1.000000000000000000, 0.9510565162951535312, 1.000000000000000000, 0.9510565162951535312, 1.000000000000000000, 0.9510565162951535312, 1.000000000000000000, 0.9510565162951535312, 1.000000000000000000, 0.9510565162951535312, 1.000000000000000000, 0.9510565162951535312, 1.000000000000000000, 0.9510565162951535312, 1.000000000000000000, 0.9510565162951535312, 1.000000000000000000, 0.9510565162951535312, 1.000000000000000000, 0.9510565162951535312, 1.000000000000000000, 0.9510565162951535312, 1.000000000000000000, 0.9510565162951535312, 1.000000000000000000, 0.9510565162951535312, 1.000000000000000000, 0.9510565162951535312, 1.000000000000000000, 0.9510565162951535312, 1.000000000000000000, 0.9510565162951535312, 1.000000000000000000, 0.9510565162951535312, 1.000000000000000000, 0.9510565162951535312, 1.000000000000000000, 0.9510565162951535312, 1.000000000000000000, 0.9510565162951535312, 1.000000000000000000, 0.9510565162951535312, 1.000000000000000000, 0.9510565162951535312, 1.000000000000000000, 0.9510565162951535312, 1.000000000000000000, 0.9510565162951535312, 1.000000000000000000, 0.9510565162951535312, 1.000000000000000000, 0.9510565162951535312, 1.000000000000000000, 0.9510565162951535312, 1.000000000000000000, 0.9510565162951535312, 1.000000000000000000, 0.9510565162951535312, 1.000000000000000000, 0.9510565162951535312, 1.000000000000000000, 0.9510565162951535312, 1.000000000000000000, 0.9510565162951535312, 1.000000000000000000, 0.9510565162951535312, 1.000000000000000000, 0.9510565162951535312, 1.000000000000000000, 0.9510565162951535312, 1.000000000000000000, 0.9510565162951535312, 1.000000000000000000, 0.9510565162951535312, 1.000000000000000000, 0.9510565162951535312, 1.000000000000000000, 0.9510565162951535312, 1.000000000000000000, 0.9510565162951535312, 1.000000000000000000, 0.9510565162951535312, 1.000000000000000000, 0.9510565162951535312, 1.000000000000000000, 0.9510565162951535312, 1.000000000000000000, 0.9510565162951535312, 1.000000000000000000, 0.9510565162951535312, 1.000000000000000000, 0.9510565162951535312, 1.000000000000000000, 0.9510565162951535312, 1.000000000000000000, 0.9510565162951535312, 1.000000000000000000, 0.9510565162951535312, 1.000000000000000000, 0.9510565162951535312, 1.000000000000000000, 0.9510565162951535312, 1.000000000000000000, 0.9510565162951535312, 1.000000000000000000, 0.9510565162951535312, 1.000000000000000000, 0.9510565162951535312, 1.000000000000000000, 0.9510565162951535312, 1.000000000000000000, 0.9510565162951535312, 1.000000000000000000, 0.9510565162951535312, 1.000000000000000000, 0.9510565162951535312, 1.000000000000000000, 0.9510565162951535312, 1.000000000000000000, 0.9510565162951535312, 1.000000000000000000, 0.9510565162951535312, 1.000000000000000000, 0.9510565162951535312, 1.000000000000000000, 0.9510565162951535312, 1.000000000000000000, 0.9510565162951535312, 1.000000000000000000, 0.9510565162951535312, 1.000000000000000000, 0.9510565162951535312, 1.000000000000000000 ) ) 
 REPRESENTATION_ITEM ( '' )  );
#2969=CARTESIAN_POINT ( 'NONE',  ( 7.324799518705101598, 26.80913330496100855, 87.63976656848456059 ) ) ;
#2974=CARTESIAN_POINT ( 'NONE',  ( 26.45000000109246585, 15.59161060780646046, 84.72553407664153724 ) ) ;
#2978=CARTESIAN_POINT ( 'NONE',  ( 37.05000000109246372, 27.13292387221364876, 88.47553407664153724 ) ) ;
#2980=AXIS2_PLACEMENT_3D ( 'NONE', #2135, #5946, #8930 ) ;
#2981=CARTESIAN_POINT ( 'NONE',  ( 20.37500000054621907, 12.34168156654572357, 90.79316153445363113 ) ) ;
#2982=CARTESIAN_POINT ( 'NONE',  ( 35.67500000054622689, 22.36655054427230027, 98.07665518445361386 ) ) ;
#2983=CARTESIAN_POINT ( 'NONE',  ( 23.57500000054622546, 26.19570976099943493, 95.29460816699764791 ) ) ;
#2984=CARTESIAN_POINT ( 'NONE',  ( 20.49999999999998224, 12.11403331821300533, 90.79316153445363113 ) ) ;
#2986=CARTESIAN_POINT ( 'NONE',  ( 32.57500000054623257, 15.71886984736413773, 84.90069139318163138 ) ) ;
#2988=DIRECTION ( 'NONE',  ( -1.000000000000000000, 0.000000000000000000, 0.000000000000000000 ) ) ;
#2989=VERTEX_POINT ( 'NONE', #5399 ) ;
#2992=LINE ( 'NONE', #9975, #10646 ) ;
#2994=CARTESIAN_POINT ( 'NONE',  ( 38.57500000054621836, 13.80429023900056684, 86.29171490190961435 ) ) ;
#2995=FACE_BOUND ( 'NONE', #450, .T. ) ;
#2996=EDGE_CURVE ( 'NONE', #5544, #2895, #8559, .T. ) ;
#2997=CARTESIAN_POINT ( 'NONE',  ( 46.57500000054623257, 13.80429023900056684, 86.29171490190961435 ) ) ;
#2998=CARTESIAN_POINT ( 'NONE',  ( 41.49999999999997158, 27.88596668178699645, 90.79316153445363113 ) ) ;
#2999=LINE ( 'NONE', #9792, #886 ) ;
#3000=CARTESIAN_POINT ( 'NONE',  ( 27.50000000000000355, 27.49999999999999645, 145.0000000000000000 ) ) ;
#3002=CARTESIAN_POINT ( 'NONE',  ( 28.85000000109246443, 24.40838939219355197, 84.72553407664153724 ) ) ;
#3008=LINE ( 'NONE', #9931, #4736 ) ;
#3009=CIRCLE ( 'NONE', #4423, 7.500000000000000000 ) ;
#3010=CARTESIAN_POINT ( 'NONE',  ( 38.27500000054623541, 12.34168156654572535, 90.79316153445363113 ) ) ;
#3011=CARTESIAN_POINT ( 'NONE',  ( 30.97500000054622760, 22.36655054427230382, 83.50966788445364841 ) ) ;
#3013=CARTESIAN_POINT ( 'NONE',  ( 43.65000000109246514, 20.00000000000000355, 98.29316153445363113 ) ) ;
#3021=AXIS2_PLACEMENT_3D ( 'NONE', #3237, #1154, #9776 ) ;
#3033=CARTESIAN_POINT ( 'NONE',  ( 41.47500000054623115, 26.19570976099943493, 95.29460816699764791 ) ) ;
#3039=( BOUNDED_CURVE ( )  B_SPLINE_CURVE ( 2, ( #4433, #10389, #512, #3602, #3482, #9141, #12181, #12058, #7350, #3359, #11221 ),
 .UNSPECIFIED., .F., .F. ) 
 B_SPLINE_CURVE_WITH_KNOTS ( ( 3, 2, 2, 2, 2, 3 ),
 ( 0.4666666666666666186, 0.4733333333333332726, 0.4799999999999999267, 0.4866666666666666918, 0.4933333333333333459, 0.5000000000000000000 ),
 .UNSPECIFIED. ) 
 CURVE ( )  GEOMETRIC_REPRESENTATION_ITEM ( )  RATIONAL_B_SPLINE_CURVE ( ( 1.000000000000000444, 0.9510565162951531981, 1.000000000000000000, 0.9510565162951535312, 1.000000000000000000, 0.9510565162951535312, 1.000000000000000000, 0.9510565162951535312, 1.000000000000000000, 0.9510565162951535312, 1.000000000000000000 ) ) 
 REPRESENTATION_ITEM ( '' )  );
#3040=CARTESIAN_POINT ( 'NONE',  ( 20.27500000054622475, 13.07298590277314254, 93.04388485072563242 ) ) ;
#3041=CARTESIAN_POINT ( 'NONE',  ( 24.65000000109246514, 20.00000000000000355, 83.29316153445364534 ) ) ;
#3043=CARTESIAN_POINT ( 'NONE',  ( 35.97500000054623115, 15.71886984736413417, 96.68563167572563088 ) ) ;
#3046=CARTESIAN_POINT ( 'NONE',  ( 23.87500000054622262, 20.00000000000000355, 98.07665518445361386 ) ) ;
#3047=CARTESIAN_POINT ( 'NONE',  ( 24.29999999999999005, 13.62011893735971135, 95.42841645007781892 ) ) ;
#3048=DIRECTION ( 'NONE',  ( 0.000000000000000000, 0.000000000000000000, -1.000000000000000000 ) ) ;
#3049=CARTESIAN_POINT ( 'NONE',  ( 34.67500000054621268, 17.63344945572770328, 83.50966788445364841 ) ) ;
#3052=VERTEX_POINT ( 'NONE', #6899 ) ;
#3054=ORIENTED_EDGE ( 'NONE', *, *, #11635, .F. ) ;
#3055=CARTESIAN_POINT ( 'NONE',  ( -50.00000000000001421, 22.00000000000000000, 188.4007504869563263 ) ) ;
#3056=CYLINDRICAL_SURFACE ( 'NONE', #8069, 7.499999999999992895 ) ;
#3057=VECTOR ( 'NONE', #11045, 1000.000000000000000 ) ;
#3058=CARTESIAN_POINT ( 'NONE',  ( 35.67500000054622689, 24.28113015263587116, 96.68563167572563088 ) ) ;
#3060=CARTESIAN_POINT ( 'NONE',  ( 49.77500000054622831, 20.00000000000000355, 98.07665518445361386 ) ) ;
#3061=CARTESIAN_POINT ( 'NONE',  ( 41.67500000054622689, 24.28113015263587116, 96.68563167572563088 ) ) ;
#3062=CARTESIAN_POINT ( 'NONE',  ( 40.79999999999999005, 15.59161060780646046, 84.72553407664153724 ) ) ;
#3063=CARTESIAN_POINT ( 'NONE',  ( 39.79999999999999005, 24.40838939219354842, 96.86078899226572503 ) ) ;
#3065=ORIENTED_EDGE ( 'NONE', *, *, #6049, .F. ) ;
#3066=CARTESIAN_POINT ( 'NONE',  ( 33.15000000109246514, 27.88596668178699645, 90.79316153445363113 ) ) ;
#3073=CARTESIAN_POINT ( 'NONE',  ( 31.77500000054622831, 20.00000000000000355, 98.07665518445361386 ) ) ;
#3074=CARTESIAN_POINT ( 'NONE',  ( 29.37500000054622618, 27.65831843345427998, 90.79316153445363113 ) ) ;
#3075=CARTESIAN_POINT ( 'NONE',  ( 44.35000000109246798, 13.62011893735970958, 86.15790661882942914 ) ) ;
#3077=ORIENTED_EDGE ( 'NONE', *, *, #8511, .F. ) ;
#3078=CARTESIAN_POINT ( 'NONE',  ( 49.27500000054622120, 26.92701409722686634, 88.54243821818162985 ) ) ;
#3079=CARTESIAN_POINT ( 'NONE',  ( 47.25000000109246656, 27.13292387221364876, 93.11078899226573924 ) ) ;
#3081=CARTESIAN_POINT ( 'NONE',  ( 19.65000000109246514, 20.00000000000000355, 98.29316153445363113 ) ) ;
#3084=CARTESIAN_POINT ( 'NONE',  ( -6.999999999999999112, 40.00000000000000000, 132.8533255156884820 ) ) ;
#3088=CARTESIAN_POINT ( 'NONE',  ( 7.147088427834759727, 26.99542114996404507, 93.50820798009134194 ) ) ;
#3093=CARTESIAN_POINT ( 'NONE',  ( 43.47500000054623115, 26.19570976099943493, 95.29460816699764791 ) ) ;
#3095=CARTESIAN_POINT ( 'NONE',  ( -20.00000000000000355, 24.39339828220178674, 137.5000000000000000 ) ) ;
#3098=EDGE_CURVE ( 'NONE', #10212, #3211, #4046, .T. ) ;
#3099=EDGE_CURVE ( 'NONE', #5557, #9486, #2641, .T. ) ;
#3101=VECTOR ( 'NONE', #1629, 1000.000000000000000 ) ;
#3102=CARTESIAN_POINT ( 'NONE',  ( 34.57500000054623257, 15.71886984736413773, 84.90069139318163138 ) ) ;
#3103=CARTESIAN_POINT ( 'NONE',  ( 21.37500000054622262, 27.65831843345427998, 90.79316153445363113 ) ) ;
#3104=CARTESIAN_POINT ( 'NONE',  ( 24.19999999999998863, 15.59161060780645691, 96.86078899226572503 ) ) ;
#3106=CARTESIAN_POINT ( 'NONE',  ( -50.00000000000001421, 92.00000000000000000, 166.8533255156881694 ) ) ;
#3107=CARTESIAN_POINT ( 'NONE',  ( 25.07500000054623257, 26.19570976099943493, 86.29171490190961435 ) ) ;
#3108=ORIENTED_EDGE ( 'NONE', *, *, #6601, .T. ) ;
#3110=FACE_OUTER_BOUND ( 'NONE', #5693, .T. ) ;
#3113=ORIENTED_EDGE ( 'NONE', *, *, #6355, .T. ) ;
#3114=CIRCLE ( 'NONE', #4537, 7.499999999999992895 ) ;
#3119=CARTESIAN_POINT ( 'NONE',  ( 40.25000000109246656, 12.86707612778636012, 88.47553407664152303 ) ) ;
#3120=CARTESIAN_POINT ( 'NONE',  ( 26.89999999999998792, 17.56310227825324333, 83.29316153445360271 ) ) ;
#3121=CARTESIAN_POINT ( 'NONE',  ( 40.47500000054622404, 13.07298590277314432, 88.54243821818161564 ) ) ;
#3122=CARTESIAN_POINT ( 'NONE',  ( 40.29999999999997584, 13.62011893735971135, 95.42841645007781892 ) ) ;
#3124=CARTESIAN_POINT ( 'NONE',  ( 0.000000000000000000, 20.00000000000000355, 69.99999999999998579 ) ) ;
#3127=VECTOR ( 'NONE', #3327, 1000.000000000000000 ) ;
#3128=CARTESIAN_POINT ( 'NONE',  ( 31.25000000109246656, 27.13292387221364876, 93.11078899226573924 ) ) ;
#3130=ORIENTED_EDGE ( 'NONE', *, *, #6068, .T. ) ;
#3131=FACE_OUTER_BOUND ( 'NONE', #7454, .T. ) ;
#3134=FACE_OUTER_BOUND ( 'NONE', #9033, .T. ) ;
#3136=DIRECTION ( 'NONE',  ( 0.000000000000000000, 0.000000000000000000, -1.000000000000000000 ) ) ;
#3137=CARTESIAN_POINT ( 'NONE',  ( 31.07500000054622191, 26.19570976099943493, 86.29171490190961435 ) ) ;
#3138=CARTESIAN_POINT ( 'NONE',  ( 29.77500000054622120, 22.36655054427230027, 98.07665518445361386 ) ) ;
#3141=CARTESIAN_POINT ( 'NONE',  ( 33.95000000109246940, 13.62011893735970958, 95.42841645007781892 ) ) ;
#3145=CARTESIAN_POINT ( 'NONE',  ( -34.99999999999997868, 20.00000000000000000, 137.5000000000000000 ) ) ;
#3156=CARTESIAN_POINT ( 'NONE',  ( 6.689122664262947993, 27.43351973878651862, 91.82200081781293477 ) ) ;
#3161=CARTESIAN_POINT ( 'NONE',  ( -6.999999999999999112, 84.49999999999998579, 101.8533255156881978 ) ) ;
#3162=CARTESIAN_POINT ( 'NONE',  ( 44.37500000054622973, 13.07298590277314432, 88.54243821818161564 ) ) ;
#3163=CARTESIAN_POINT ( 'NONE',  ( -23.10660171779820971, 27.49999999999999645, 140.6066017177982133 ) ) ;
#3165=ADVANCED_FACE ( 'NONE', ( #7923 ), #5771, .F. ) ;
#3169=CARTESIAN_POINT ( 'NONE',  ( 21.47500000054622404, 26.92701409722686634, 93.04388485072563242 ) ) ;
#3170=CARTESIAN_POINT ( 'NONE',  ( 42.67500000054622689, 15.71886984736413773, 84.90069139318163138 ) ) ;
#3171=VECTOR ( 'NONE', #1255, 1000.000000000000000 ) ;
#3172=CARTESIAN_POINT ( 'NONE',  ( 35.87500000054622262, 17.63344945572769973, 98.07665518445361386 ) ) ;
#3173=CARTESIAN_POINT ( 'NONE',  ( 21.17500000054622689, 26.19570976099943493, 86.29171490190961435 ) ) ;
#3174=CARTESIAN_POINT ( 'NONE',  ( 21.89999999999999147, 22.43689772174679575, 98.29316153445363113 ) ) ;
#3175=FACE_OUTER_BOUND ( 'NONE', #12522, .T. ) ;
#3176=CARTESIAN_POINT ( 'NONE',  ( 28.17500000054622689, 13.07298590277314254, 93.04388485072563242 ) ) ;
#3177=ORIENTED_EDGE ( 'NONE', *, *, #2508, .T. ) ;
#3179=EDGE_CURVE ( 'NONE', #1799, #3939, #9343, .T. ) ;
#3180=CARTESIAN_POINT ( 'NONE',  ( 23.15000000109246514, 27.88596668178699645, 90.79316153445363113 ) ) ;
#3187=CARTESIAN_POINT ( 'NONE',  ( 40.55000000109246372, 17.56310227825320425, 83.29316153445363113 ) ) ;
#3189=CARTESIAN_POINT ( 'NONE',  ( 39.97500000054623115, 17.63344945572769973, 98.07665518445361386 ) ) ;
#3190=CARTESIAN_POINT ( 'NONE',  ( 45.19999999999998863, 24.40838939219355197, 84.72553407664153724 ) ) ;
#3192=CARTESIAN_POINT ( 'NONE',  ( 48.67500000054623399, 17.63344945572770328, 83.50966788445364841 ) ) ;
#3194=CARTESIAN_POINT ( 'NONE',  ( 24.65000000109246514, 20.00000000000000355, 83.29316153445364534 ) ) ;
#3195=CARTESIAN_POINT ( 'NONE',  ( -50.00000000000001421, 40.00000000000000000, 69.99999999999998579 ) ) ;
#3197=CARTESIAN_POINT ( 'NONE',  ( 23.19999999999998863, 24.40838939219355197, 84.72553407664153724 ) ) ;
#3198=VERTEX_POINT ( 'NONE', #12488 ) ;
#3200=EDGE_CURVE ( 'NONE', #10184, #4281, #3793, .T. ) ;
#3204=CARTESIAN_POINT ( 'NONE',  ( 27.77500000054622831, 20.00000000000000355, 98.07665518445361386 ) ) ;
#3205=CARTESIAN_POINT ( 'NONE',  ( 34.17500000054622689, 13.80429023900056507, 95.29460816699764791 ) ) ;
#3206=CARTESIAN_POINT ( 'NONE',  ( -50.00000000000001421, 92.00000000000000000, 69.99999999999998579 ) ) ;
#3211=VERTEX_POINT ( 'NONE', #4300 ) ;
#3213=DIRECTION ( 'NONE',  ( 0.000000000000000000, 0.000000000000000000, -1.000000000000000000 ) ) ;
#3215=CARTESIAN_POINT ( 'NONE',  ( -6.500000000000214051, 0.000000000000000000, 26.49999999999998934 ) ) ;
#3219=CARTESIAN_POINT ( 'NONE',  ( -5.000000000000000888, 22.00000000000000000, 169.9999999999999716 ) ) ;
#3221=CARTESIAN_POINT ( 'NONE',  ( 6.899297396606579369, 27.24035709017728379, 88.77211908039561195 ) ) ;
#3223=CARTESIAN_POINT ( 'NONE',  ( 34.99999999999999289, 20.00000000000000355, 99.99999999999997158 ) ) ;
#3227=CARTESIAN_POINT ( 'NONE',  ( 42.47500000054622404, 13.80429023900056684, 86.29171490190961435 ) ) ;
#3229=ORIENTED_EDGE ( 'NONE', *, *, #6546, .T. ) ;
#3232=CARTESIAN_POINT ( 'NONE',  ( 23.97500000054622049, 17.63344945572769973, 98.07665518445361386 ) ) ;
#3233=CARTESIAN_POINT ( 'NONE',  ( 46.37500000054621552, 12.34168156654572535, 90.79316153445363113 ) ) ;
#3234=CARTESIAN_POINT ( 'NONE',  ( 33.17500000054622689, 26.92701409722686634, 88.54243821818162985 ) ) ;
#3237=CARTESIAN_POINT ( 'NONE',  ( -2.000000000000015543, 20.00000000000000355, 90.79316153445363113 ) ) ;
#3238=CARTESIAN_POINT ( 'NONE',  ( 28.07500000054622902, 13.80429023900056507, 95.29460816699764791 ) ) ;
#3240=LINE ( 'NONE', #2289, #1237 ) ;
#3242=ORIENTED_EDGE ( 'NONE', *, *, #11448, .T. ) ;
#3243=CARTESIAN_POINT ( 'NONE',  ( -21.00000000000001066, 77.00000000000000000, 166.8533255156881694 ) ) ;
#3246=CARTESIAN_POINT ( 'NONE',  ( 38.67500000054622689, 15.71886984736413773, 84.90069139318163138 ) ) ;
#3249=CARTESIAN_POINT ( 'NONE',  ( 19.65000000109246514, 20.00000000000000355, 98.29316153445363113 ) ) ;
#3250=CARTESIAN_POINT ( 'NONE',  ( 38.07500000054622546, 15.71886984736413417, 96.68563167572563088 ) ) ;
#3251=CARTESIAN_POINT ( 'NONE',  ( 37.29999999999998295, 26.37988106264029398, 86.15790661882942914 ) ) ;
#3252=CARTESIAN_POINT ( 'NONE',  ( 49.07500000054622546, 26.19570976099943493, 86.29171490190961435 ) ) ;
#3254=CARTESIAN_POINT ( 'NONE',  ( 22.35000000109246443, 13.62011893735971135, 86.15790661882942914 ) ) ;
#3257=( BOUNDED_CURVE ( )  B_SPLINE_CURVE ( 2, ( #1823, #4937, #2974, #2780, #6840, #2909, #6642, #6708, #5709, #4751, #4816 ),
 .UNSPECIFIED., .F., .F. ) 
 B_SPLINE_CURVE_WITH_KNOTS ( ( 3, 2, 2, 2, 2, 3 ),
 ( 0.7666666666666666075, 0.7733333333333332060, 0.7799999999999999156, 0.7866666666666666252, 0.7933333333333333348, 0.8000000000000000444 ),
 .UNSPECIFIED. ) 
 CURVE ( )  GEOMETRIC_REPRESENTATION_ITEM ( )  RATIONAL_B_SPLINE_CURVE ( ( 1.000000000000000888, 0.9510565162951527540, 1.000000000000000000, 0.9510565162951535312, 1.000000000000000000, 0.9510565162951535312, 1.000000000000000000, 0.9510565162951535312, 1.000000000000000000, 0.9510565162951535312, 1.000000000000000000 ) ) 
 REPRESENTATION_ITEM ( '' )  );
#3260=VECTOR ( 'NONE', #2532, 1000.000000000000000 ) ;
#3261=DIRECTION ( 'NONE',  ( -1.000000000000000000, 0.000000000000000000, -0.000000000000000000 ) ) ;
#3267=CARTESIAN_POINT ( 'NONE',  ( 30.27500000054623186, 12.34168156654572535, 90.79316153445363113 ) ) ;
#3268=CARTESIAN_POINT ( 'NONE',  ( 33.47500000054622404, 26.92701409722686634, 93.04388485072563242 ) ) ;
#3270=CARTESIAN_POINT ( 'NONE',  ( 22.15000000109246514, 12.11403331821300533, 90.79316153445363113 ) ) ;
#3271=ORIENTED_EDGE ( 'NONE', *, *, #11604, .F. ) ;
#3274=CARTESIAN_POINT ( 'NONE',  ( 42.55000000109245661, 17.56310227825321135, 83.29316153445363113 ) ) ;
#3276=VERTEX_POINT ( 'NONE', #1206 ) ;
#3292=CARTESIAN_POINT ( 'NONE',  ( 28.89999999999998437, 17.56310227825320425, 83.29316153445363113 ) ) ;
#3293=CARTESIAN_POINT ( 'NONE',  ( 43.47500000054622404, 26.92701409722686634, 93.04388485072563242 ) ) ;
#3294=CARTESIAN_POINT ( 'NONE',  ( 26.47500000054622760, 13.80429023900056684, 86.29171490190961435 ) ) ;
#3295=CARTESIAN_POINT ( 'NONE',  ( 9.410854331999907174, 16.58509554716785317, 97.48886294417630438 ) ) ;
#3298=CARTESIAN_POINT ( 'NONE',  ( 26.87500000054622618, 22.36655054427230382, 83.50966788445364841 ) ) ;
#3300=CARTESIAN_POINT ( 'NONE',  ( 23.05000000109246372, 27.13292387221364876, 88.47553407664153724 ) ) ;
#3301=VERTEX_POINT ( 'NONE', #437 ) ;
#3302=LINE ( 'NONE', #1281, #9961 ) ;
#3303=ORIENTED_EDGE ( 'NONE', *, *, #5968, .F. ) ;
#3304=CIRCLE ( 'NONE', #6938, 10.00000000000000355 ) ;
#3305=CARTESIAN_POINT ( 'NONE',  ( 35.27500000054622120, 26.92701409722686634, 88.54243821818162985 ) ) ;
#3306=DIRECTION ( 'NONE',  ( 0.000000000000000000, 0.000000000000000000, -1.000000000000000000 ) ) ;
#3307=CARTESIAN_POINT ( 'NONE',  ( 20.45000000109246585, 15.59161060780646046, 84.72553407664153724 ) ) ;
#3308=CARTESIAN_POINT ( 'NONE',  ( 31.27500000054622831, 26.92701409722686634, 88.54243821818162985 ) ) ;
#3309=CARTESIAN_POINT ( 'NONE',  ( 34.19999999999998863, 15.59161060780645691, 96.86078899226572503 ) ) ;
#3310=EDGE_CURVE ( 'NONE', #2251, #11822, #12002, .T. ) ;
#3311=CARTESIAN_POINT ( 'NONE',  ( 42.97500000054623115, 24.28113015263587471, 84.90069139318163138 ) ) ;
#3312=VERTEX_POINT ( 'NONE', #10142 ) ;
#3314=CARTESIAN_POINT ( 'NONE',  ( 22.05000000109246372, 12.86707612778636012, 93.11078899226572503 ) ) ;
#3318=CARTESIAN_POINT ( 'NONE',  ( 36.85000000109246798, 24.40838939219355197, 84.72553407664153724 ) ) ;
#3319=ORIENTED_EDGE ( 'NONE', *, *, #7383, .T. ) ;
#3320=CARTESIAN_POINT ( 'NONE',  ( -2.000000000000015543, 20.00000000000000355, 90.79316153445363113 ) ) ;
#3321=CARTESIAN_POINT ( 'NONE',  ( 36.45000000109246940, 15.59161060780646046, 84.72553407664153724 ) ) ;
#3322=DIRECTION ( 'NONE',  ( -1.000000000000000000, 0.000000000000000000, 0.000000000000000000 ) ) ;
#3324=CARTESIAN_POINT ( 'NONE',  ( 28.07500000054622902, 13.80429023900056507, 95.29460816699764791 ) ) ;
#3325=CARTESIAN_POINT ( 'NONE',  ( 22.17500000054622333, 13.80429023900056507, 95.29460816699764791 ) ) ;
#3327=DIRECTION ( 'NONE',  ( -1.000000000000000000, -0.000000000000000000, -0.000000000000000000 ) ) ;
#3328=( BOUNDED_CURVE ( )  B_SPLINE_CURVE ( 3, ( #12303, #11039, #3360, #7229 ),
 .UNSPECIFIED., .F., .F. ) 
 B_SPLINE_CURVE_WITH_KNOTS ( ( 4, 4 ),
 ( 3.141592653589793116, 4.712388980384689674 ),
 .UNSPECIFIED. ) 
 CURVE ( )  GEOMETRIC_REPRESENTATION_ITEM ( )  RATIONAL_B_SPLINE_CURVE ( ( 1.000000000000000000, 0.8047378541243649375, 0.8047378541243649375, 1.000000000000000000 ) ) 
 REPRESENTATION_ITEM ( '' )  );
#3329=PLANE ( 'NONE',  #571 ) ;
#3331=CARTESIAN_POINT ( 'NONE',  ( 44.55000000109245661, 17.56310227825321135, 83.29316153445363113 ) ) ;
#3333=ORIENTED_EDGE ( 'NONE', *, *, #7811, .F. ) ;
#3334=CARTESIAN_POINT ( 'NONE',  ( 47.49999999999997868, 27.88596668178699645, 90.79316153445363113 ) ) ;
#3336=ORIENTED_EDGE ( 'NONE', *, *, #6601, .F. ) ;
#3344=CARTESIAN_POINT ( 'NONE',  ( -10.00000000000000355, 20.00000000000000355, 109.9999999999999858 ) ) ;
#3348=ORIENTED_EDGE ( 'NONE', *, *, #490, .F. ) ;
#3353=LINE ( 'NONE', #1459, #7836 ) ;
#3354=CARTESIAN_POINT ( 'NONE',  ( 42.57500000054622546, 13.80429023900056684, 86.29171490190961435 ) ) ;
#3355=CARTESIAN_POINT ( 'NONE',  ( 29.27500000054622831, 27.65831843345427998, 90.79316153445363113 ) ) ;
#3356=CARTESIAN_POINT ( 'NONE',  ( 9.621280771571464996, 17.26369774818443759, 83.80577239012578161 ) ) ;
#3357=FACE_OUTER_BOUND ( 'NONE', #1466, .T. ) ;
#3359=CARTESIAN_POINT ( 'NONE',  ( 35.09999999999998721, 22.43689772174679575, 83.29316153445363113 ) ) ;
#3360=CARTESIAN_POINT ( 'NONE',  ( -32.89339828220179385, 69.50000000000000000, 151.2467237978899846 ) ) ;
#3361=EDGE_CURVE ( 'NONE', #9944, #11196, #11592, .T. ) ;
#3363=CARTESIAN_POINT ( 'NONE',  ( -111.8465843842649292, 77.00000000000000000, 101.8533255156881978 ) ) ;
#3364=ORIENTED_EDGE ( 'NONE', *, *, #5202, .F. ) ;
#3367=CARTESIAN_POINT ( 'NONE',  ( 34.07500000054622546, 15.71886984736413417, 96.68563167572563088 ) ) ;
#3369=CARTESIAN_POINT ( 'NONE',  ( 45.97500000054623115, 15.71886984736413417, 96.68563167572563088 ) ) ;
#3371=CARTESIAN_POINT ( 'NONE',  ( 36.47500000054622404, 13.07298590277314432, 88.54243821818161564 ) ) ;
#3372=CARTESIAN_POINT ( 'NONE',  ( 34.79999999999999005, 15.59161060780646046, 84.72553407664153724 ) ) ;
#3373=CARTESIAN_POINT ( 'NONE',  ( 46.67500000054623399, 17.63344945572770328, 83.50966788445364841 ) ) ;
#3374=VERTEX_POINT ( 'NONE', #2708 ) ;
#3375=CARTESIAN_POINT ( 'NONE',  ( 23.35000000109246798, 26.37988106264029398, 95.42841645007781892 ) ) ;
#3378=ORIENTED_EDGE ( 'NONE', *, *, #5111, .F. ) ;
#3382=CARTESIAN_POINT ( 'NONE',  ( 36.99999999999999289, 20.00000000000000355, 83.29316153445364534 ) ) ;
#3387=CARTESIAN_POINT ( 'NONE',  ( 22.37500000054622973, 13.07298590277314432, 88.54243821818161564 ) ) ;
#3388=CARTESIAN_POINT ( 'NONE',  ( 24.17500000054622689, 13.80429023900056507, 95.29460816699764791 ) ) ;
#3390=CARTESIAN_POINT ( 'NONE',  ( 21.95000000109245875, 13.62011893735970958, 95.42841645007781892 ) ) ;
#3391=EDGE_LOOP ( 'NONE', ( #530, #5759, #12470, #11713, #8982 ) ) ;
#3392=CARTESIAN_POINT ( 'NONE',  ( 45.05000000109246372, 27.13292387221364876, 88.47553407664153724 ) ) ;
#3396=VERTEX_POINT ( 'NONE', #9503 ) ;
#3409=CARTESIAN_POINT ( 'NONE',  ( 47.35000000109245377, 26.37988106264029398, 95.42841645007781892 ) ) ;
#3414=CYLINDRICAL_SURFACE ( 'NONE', #9057, 7.499999999999992895 ) ;
#3416=CARTESIAN_POINT ( 'NONE',  ( 44.37500000054622262, 12.34168156654572535, 90.79316153445363113 ) ) ;
#3417=EDGE_CURVE ( 'NONE', #2160, #12416, #5449, .T. ) ;
#3418=CARTESIAN_POINT ( 'NONE',  ( 29.37500000054622973, 26.92701409722686634, 93.04388485072563242 ) ) ;
#3419=VECTOR ( 'NONE', #4237, 1000.000000000000000 ) ;
#3423=CARTESIAN_POINT ( 'NONE',  ( -111.8465843842649292, 77.00000000000000000, 146.8533255156881978 ) ) ;
#3426=DIRECTION ( 'NONE',  ( 0.000000000000000000, 0.000000000000000000, 1.000000000000000000 ) ) ;
#3427=ORIENTED_EDGE ( 'NONE', *, *, #8133, .T. ) ;
#3428=DIRECTION ( 'NONE',  ( -0.000000000000000000, -0.000000000000000000, 1.000000000000000000 ) ) ;
#3431=AXIS2_PLACEMENT_3D ( 'NONE', #11099, #8372, #6282 ) ;
#3432=ADVANCED_FACE ( 'NONE', ( #5105 ), #283, .F. ) ;
#3435=CARTESIAN_POINT ( 'NONE',  ( 32.97500000054621694, 22.36655054427230382, 83.50966788445364841 ) ) ;
#3437=CARTESIAN_POINT ( 'NONE',  ( 43.67500000054621978, 22.36655054427230027, 98.07665518445361386 ) ) ;
#3438=CARTESIAN_POINT ( 'NONE',  ( 32.27500000054622831, 13.07298590277314254, 93.04388485072563242 ) ) ;
#3439=CARTESIAN_POINT ( 'NONE',  ( 37.09999999999998010, 22.43689772174679575, 83.29316153445363113 ) ) ;
#3441=CARTESIAN_POINT ( 'NONE',  ( 47.47500000054623115, 26.19570976099943493, 95.29460816699764791 ) ) ;
#3443=CARTESIAN_POINT ( 'NONE',  ( 28.05000000109246372, 12.86707612778636012, 93.11078899226572503 ) ) ;
#3447=ORIENTED_EDGE ( 'NONE', *, *, #4084, .F. ) ;
#3449=FACE_OUTER_BOUND ( 'NONE', #6539, .T. ) ;
#3451=( BOUNDED_CURVE ( )  B_SPLINE_CURVE ( 2, ( #6735, #5034, #8832, #11631, #3884, #9731, #6992, #4908, #10600, #1913, #87 ),
 .UNSPECIFIED., .F., .F. ) 
 B_SPLINE_CURVE_WITH_KNOTS ( ( 3, 2, 2, 2, 2, 3 ),
 ( 0.1333333333333334425, 0.1400000000000000966, 0.1466666666666666952, 0.1533333333333333215, 0.1599999999999999756, 0.1666666666666665741 ),
 .UNSPECIFIED. ) 
 CURVE ( )  GEOMETRIC_REPRESENTATION_ITEM ( )  RATIONAL_B_SPLINE_CURVE ( ( 0.9999999999999992228, 0.9510565162951543083, 1.000000000000000000, 0.9510565162951535312, 1.000000000000000000, 0.9510565162951535312, 1.000000000000000000, 0.9510565162951535312, 1.000000000000000000, 0.9510565162951541973, 0.9999999999999993339 ) ) 
 REPRESENTATION_ITEM ( '' )  );
#3454=CARTESIAN_POINT ( 'NONE',  ( 21.97500000054622760, 15.71886984736413417, 96.68563167572563088 ) ) ;
#3455=CARTESIAN_POINT ( 'NONE',  ( 24.77500000054622475, 17.63344945572770328, 83.50966788445364841 ) ) ;
#3457=DIRECTION ( 'NONE',  ( -0.000000000000000000, 0.000000000000000000, -1.000000000000000000 ) ) ;
#3459=CARTESIAN_POINT ( 'NONE',  ( 41.65000000109246514, 20.00000000000000355, 98.29316153445363113 ) ) ;
#3460=VERTEX_POINT ( 'NONE', #4737 ) ;
#3462=AXIS2_PLACEMENT_3D ( 'NONE', #4377, #3426, #4191 ) ;
#3463=VERTEX_POINT ( 'NONE', #11893 ) ;
#3466=CARTESIAN_POINT ( 'NONE',  ( 29.19999999999998508, 24.40838939219355197, 84.72553407664153724 ) ) ;
#3472=ADVANCED_FACE ( 'NONE', ( #7596 ), #3778, .F. ) ;
#3474=CARTESIAN_POINT ( 'NONE',  ( 23.59999999999999076, 27.13292387221364876, 93.11078899226573924 ) ) ;
#3478=CARTESIAN_POINT ( 'NONE',  ( 36.47500000054622404, 13.07298590277314432, 88.54243821818161564 ) ) ;
#3479=CARTESIAN_POINT ( 'NONE',  ( 25.97500000054622760, 15.71886984736413417, 96.68563167572563088 ) ) ;
#3480=CARTESIAN_POINT ( 'NONE',  ( 7.416892943932571924, 13.28747952548623878, 87.41303169954825592 ) ) ;
#3482=CARTESIAN_POINT ( 'NONE',  ( 35.59999999999998721, 27.13292387221364876, 93.11078899226573924 ) ) ;
#3483=ORIENTED_EDGE ( 'NONE', *, *, #6675, .F. ) ;
#3489=CARTESIAN_POINT ( 'NONE',  ( 30.57500000054622191, 13.80429023900056684, 86.29171490190961435 ) ) ;
#3491=CARTESIAN_POINT ( 'NONE',  ( 45.27500000054622831, 27.65831843345427998, 90.79316153445363113 ) ) ;
#3492=CARTESIAN_POINT ( 'NONE',  ( 35.77500000054622831, 22.36655054427230027, 98.07665518445361386 ) ) ;
#3493=CARTESIAN_POINT ( 'NONE',  ( 33.09999999999998010, 22.43689772174679575, 83.29316153445363113 ) ) ;
#3495=CARTESIAN_POINT ( 'NONE',  ( 38.87500000054623683, 22.36655054427230382, 83.50966788445364841 ) ) ;
#3497=CARTESIAN_POINT ( 'NONE',  ( 46.37500000054622973, 13.07298590277314432, 88.54243821818161564 ) ) ;
#3506=CARTESIAN_POINT ( 'NONE',  ( 31.65000000109246514, 20.00000000000000355, 98.29316153445363113 ) ) ;
#3508=CARTESIAN_POINT ( 'NONE',  ( 21.07500000054622546, 26.19570976099943493, 86.29171490190961435 ) ) ;
#3509=CARTESIAN_POINT ( 'NONE',  ( 23.77500000054622475, 22.36655054427230027, 98.07665518445361386 ) ) ;
#3511=CARTESIAN_POINT ( 'NONE',  ( -50.00000000000001421, 77.00000000000000000, 101.8533255156881978 ) ) ;
#3514=CARTESIAN_POINT ( 'NONE',  ( 44.35000000109246798, 13.62011893735971135, 86.15790661882942914 ) ) ;
#3517=CARTESIAN_POINT ( 'NONE',  ( 47.09999999999998010, 22.43689772174677088, 83.29316153445361692 ) ) ;
#3518=ORIENTED_EDGE ( 'NONE', *, *, #6802, .T. ) ;
#3521=AXIS2_PLACEMENT_3D ( 'NONE', #11352, #5396, #11098 ) ;
#3522=ORIENTED_EDGE ( 'NONE', *, *, #2113, .F. ) ;
#3524=CARTESIAN_POINT ( 'NONE',  ( 38.45000000109246230, 15.59161060780646046, 84.72553407664153724 ) ) ;
#3525=CARTESIAN_POINT ( 'NONE',  ( 22.19999999999998863, 15.59161060780645691, 96.86078899226572503 ) ) ;
#3528=CARTESIAN_POINT ( 'NONE',  ( 29.57500000054622546, 24.28113015263587116, 96.68563167572563088 ) ) ;
#3529=DIRECTION ( 'NONE',  ( 0.000000000000000000, 0.000000000000000000, -1.000000000000000000 ) ) ;
#3533=ADVANCED_FACE ( 'NONE', ( #5700 ), #7658, .F. ) ;
#3537=CARTESIAN_POINT ( 'NONE',  ( 38.77500000054622831, 20.00000000000000355, 83.50966788445364841 ) ) ;
#3538=CARTESIAN_POINT ( 'NONE',  ( 39.87500000054622262, 20.00000000000000355, 98.07665518445361386 ) ) ;
#3539=CARTESIAN_POINT ( 'NONE',  ( 27.37500000054622973, 26.92701409722686634, 93.04388485072563242 ) ) ;
#3540=AXIS2_PLACEMENT_3D ( 'NONE', #6558, #10887, #3213 ) ;
#3541=CARTESIAN_POINT ( 'NONE',  ( 8.868804215452586348, 15.35919039895786220, 84.88169823822040883 ) ) ;
#3544=CARTESIAN_POINT ( 'NONE',  ( 31.69999999999999218, 26.37988106264029398, 95.42841645007781892 ) ) ;
#3551=CARTESIAN_POINT ( 'NONE',  ( 32.37500000054621552, 12.34168156654572357, 90.79316153445363113 ) ) ;
#3552=LINE ( 'NONE', #7488, #2690 ) ;
#3553=CARTESIAN_POINT ( 'NONE',  ( 43.47500000054623115, 26.19570976099943849, 95.29460816699764791 ) ) ;
#3554=CARTESIAN_POINT ( 'NONE',  ( 35.07500000054622546, 24.28113015263587471, 84.90069139318163138 ) ) ;
#3555=CARTESIAN_POINT ( 'NONE',  ( 27.99999999999998579, 20.00000000000000355, 98.29316153445363113 ) ) ;
#3556=ADVANCED_FACE ( 'NONE', ( #3131 ), #5758, .F. ) ;
#3558=CARTESIAN_POINT ( 'NONE',  ( 39.47500000054623115, 26.19570976099943493, 95.29460816699764791 ) ) ;
#3559=VERTEX_POINT ( 'NONE', #6999 ) ;
#3560=CARTESIAN_POINT ( 'NONE',  ( 21.45000000109246230, 24.40838939219354842, 96.86078899226572503 ) ) ;
#3569=CARTESIAN_POINT ( 'NONE',  ( 23.77500000054622831, 20.00000000000000355, 98.07665518445361386 ) ) ;
#3570=CARTESIAN_POINT ( 'NONE',  ( 27.57500000054622191, 26.19570976099943493, 95.29460816699764791 ) ) ;
#3574=EDGE_LOOP ( 'NONE', ( #11222, #4512, #10657, #9534 ) ) ;
#3575=CARTESIAN_POINT ( 'NONE',  ( 35.75000000109246656, 17.56310227825320425, 98.29316153445363113 ) ) ;
#3578=CARTESIAN_POINT ( 'NONE',  ( 0.000000000000000000, 22.00000000000000000, 169.9999999999999716 ) ) ;
#3579=ADVANCED_FACE ( 'NONE', ( #12139 ), #9102, .F. ) ;
#3580=EDGE_LOOP ( 'NONE', ( #12442, #5339, #6980, #7075 ) ) ;
#3582=CARTESIAN_POINT ( 'NONE',  ( 31.65000000109246514, 20.00000000000000355, 98.29316153445363113 ) ) ;
#3584=CARTESIAN_POINT ( 'NONE',  ( 20.47500000054622760, 13.80429023900056684, 86.29171490190961435 ) ) ;
#3587=CARTESIAN_POINT ( 'NONE',  ( 26.99999999999998934, 20.00000000000000355, 83.29316153445364534 ) ) ;
#3590=CARTESIAN_POINT ( 'NONE',  ( 21.47500000054622760, 26.19570976099943493, 95.29460816699764791 ) ) ;
#3592=CARTESIAN_POINT ( 'NONE',  ( -2.000000000000015543, 20.00000000000000355, 90.79316153445363113 ) ) ;
#3597=CARTESIAN_POINT ( 'NONE',  ( 35.57500000054622546, 24.28113015263587116, 96.68563167572563088 ) ) ;
#3598=CARTESIAN_POINT ( 'NONE',  ( 35.57500000054623257, 26.19570976099943493, 95.29460816699764791 ) ) ;
#3600=CARTESIAN_POINT ( 'NONE',  ( 4.999999999999997335, 22.00000000000000000, 152.2284161474004520 ) ) ;
#3602=CARTESIAN_POINT ( 'NONE',  ( 35.69999999999998153, 26.37988106264029398, 95.42841645007781892 ) ) ;
#3606=EDGE_LOOP ( 'NONE', ( #11875, #10588, #7671, #10674, #11008 ) ) ;
#3611=CARTESIAN_POINT ( 'NONE',  ( 47.97500000054622404, 15.71886984736413417, 96.68563167572563088 ) ) ;
#3612=CARTESIAN_POINT ( 'NONE',  ( 27.97500000054622404, 17.63344945572769973, 98.07665518445361386 ) ) ;
#3613=CARTESIAN_POINT ( 'NONE',  ( 27.29999999999998295, 26.37988106264029398, 86.15790661882942914 ) ) ;
#3614=CARTESIAN_POINT ( 'NONE',  ( -50.00000000000001421, 40.00000000000000000, 69.99999999999998579 ) ) ;
#3615=CARTESIAN_POINT ( 'NONE',  ( 36.37500000054622973, 13.07298590277314432, 88.54243821818161564 ) ) ;
#3617=CARTESIAN_POINT ( 'NONE',  ( 20.65000000109246514, 20.00000000000000355, 83.29316153445364534 ) ) ;
#3619=ORIENTED_EDGE ( 'NONE', *, *, #9086, .F. ) ;
#3621=VECTOR ( 'NONE', #8505, 1000.000000000000114 ) ;
#3623=ORIENTED_EDGE ( 'NONE', *, *, #3361, .F. ) ;
#3624=VECTOR ( 'NONE', #96, 1000.000000000000000 ) ;
#3626=CARTESIAN_POINT ( 'NONE',  ( 21.65000000109246514, 20.00000000000000355, 98.29316153445363113 ) ) ;
#3628=DIRECTION ( 'NONE',  ( 1.000000000000000000, 0.000000000000000000, 0.000000000000000000 ) ) ;
#3630=CARTESIAN_POINT ( 'NONE',  ( 27.17500000054622689, 26.92701409722686634, 88.54243821818162985 ) ) ;
#3631=CARTESIAN_POINT ( 'NONE',  ( 49.79999999999999005, 24.40838939219354842, 96.86078899226572503 ) ) ;
#3635=CARTESIAN_POINT ( 'NONE',  ( 39.25000000109246656, 27.13292387221364876, 93.11078899226573924 ) ) ;
#3636=CARTESIAN_POINT ( 'NONE',  ( 24.09999999999998366, 17.56310227825320425, 98.29316153445363113 ) ) ;
#3647=ORIENTED_EDGE ( 'NONE', *, *, #6068, .F. ) ;
#3651=CARTESIAN_POINT ( 'NONE',  ( 20.67500000054622333, 17.63344945572770328, 83.50966788445364841 ) ) ;
#3655=( BOUNDED_CURVE ( )  B_SPLINE_CURVE ( 3, ( #294, #7430, #7304, #7365 ),
 .UNSPECIFIED., .F., .F. ) 
 B_SPLINE_CURVE_WITH_KNOTS ( ( 4, 4 ),
 ( 3.141592653589793560, 4.712388980384689674 ),
 .UNSPECIFIED. ) 
 CURVE ( )  GEOMETRIC_REPRESENTATION_ITEM ( )  RATIONAL_B_SPLINE_CURVE ( ( 1.000000000000000000, 0.8047378541243650485, 0.8047378541243650485, 1.000000000000000000 ) ) 
 REPRESENTATION_ITEM ( '' )  );
#3661=CARTESIAN_POINT ( 'NONE',  ( 38.77500000054622831, 17.63344945572770328, 83.50966788445364841 ) ) ;
#3663=CARTESIAN_POINT ( 'NONE',  ( 22.67500000054622333, 17.63344945572770328, 83.50966788445364841 ) ) ;
#3665=DIRECTION ( 'NONE',  ( 0.000000000000000000, -1.000000000000000000, -0.000000000000000000 ) ) ;
#3671=CARTESIAN_POINT ( 'NONE',  ( 31.00470515163597085, 12.50000000000001243, 148.5047051516359602 ) ) ;
#3673=CARTESIAN_POINT ( 'NONE',  ( 25.87500000054622618, 20.00000000000000355, 98.07665518445361386 ) ) ;
#3674=CARTESIAN_POINT ( 'NONE',  ( 29.55000000109246727, 22.43689772174679575, 98.29316153445363113 ) ) ;
#3675=CARTESIAN_POINT ( 'NONE',  ( 39.87500000054622262, 17.63344945572769973, 98.07665518445361386 ) ) ;
#3676=CARTESIAN_POINT ( 'NONE',  ( 26.97500000054622049, 22.36655054427230382, 83.50966788445364841 ) ) ;
#3677=CARTESIAN_POINT ( 'NONE',  ( 28.79999999999999005, 15.59161060780646046, 84.72553407664153724 ) ) ;
#3679=CARTESIAN_POINT ( 'NONE',  ( 36.97500000054623115, 24.28113015263587471, 84.90069139318163138 ) ) ;
#3681=CARTESIAN_POINT ( 'NONE',  ( 48.57500000054623257, 15.71886984736413773, 84.90069139318163138 ) ) ;
#3687=CARTESIAN_POINT ( 'NONE',  ( 4.999999999999999112, -3.000000000000002665, 218.7511230907454944 ) ) ;
#3688=CARTESIAN_POINT ( 'NONE',  ( 43.37500000054622973, 27.65831843345427998, 90.79316153445363113 ) ) ;
#3689=FACE_OUTER_BOUND ( 'NONE', #9207, .T. ) ;
#3690=EDGE_CURVE ( 'NONE', #11695, #3276, #7626, .T. ) ;
#3691=CARTESIAN_POINT ( 'NONE',  ( 43.37500000054622973, 27.65831843345427998, 90.79316153445363113 ) ) ;
#3692=CARTESIAN_POINT ( 'NONE',  ( 49.49999999999998579, 27.88596668178699645, 90.79316153445363113 ) ) ;
#3694=CARTESIAN_POINT ( 'NONE',  ( 38.85000000109246798, 24.40838939219355197, 84.72553407664153724 ) ) ;
#3697=CARTESIAN_POINT ( 'NONE',  ( 40.45000000109246940, 15.59161060780646046, 84.72553407664153724 ) ) ;
#3698=CARTESIAN_POINT ( 'NONE',  ( 24.49999999999998579, 12.11403331821300533, 90.79316153445363113 ) ) ;
#3703=CARTESIAN_POINT ( 'NONE',  ( 31.35000000109246088, 26.37988106264029398, 95.42841645007781892 ) ) ;
#3706=ORIENTED_EDGE ( 'NONE', *, *, #7422, .F. ) ;
#3710=CARTESIAN_POINT ( 'NONE',  ( 22.77500000054622831, 20.00000000000000355, 83.50966788445364841 ) ) ;
#3711=CARTESIAN_POINT ( 'NONE',  ( 45.85000000109246798, 15.59161060780645691, 96.86078899226572503 ) ) ;
#3716=CARTESIAN_POINT ( 'NONE',  ( 21.09999999999998366, 22.43689772174679575, 83.29316153445363113 ) ) ;
#3724=DIRECTION ( 'NONE',  ( 1.000000000000000000, -0.000000000000000000, -0.000000000000000000 ) ) ;
#3725=( BOUNDED_CURVE ( )  B_SPLINE_CURVE ( 2, ( #8990, #107, #7904, #8983, #2059, #2125, #3078, #6943, #7968, #8916, #1124, #297, #4989, #41, #8849, #11773, #4092, #11836, #2196, #6067, #5118, #9939, #1247, #1972, #972, #10539, #5731, #10596, #5606, #1848, #12512, #5856, #9725, #9598, #906, #12451, #8518, #1042, #4902, #11436, #2869, #6669, #8762, #6796, #3943, #1908, #4776, #4840, #8641, #3817, #3751, #6729, #10474, #5671, #5793, #2932, #7568, #80, #9664, #10661, #1786, #11376, #16, #3879, #2682, #3688, #7753, #6547, #6605, #11624, #10414, #1728, #9479, #779, #2747, #4647, #12391, #9541, #840, #4708, #8580, #7633, #11496, #2804, #10724, #7047, #8959, #10787, #7880, #5030, #273, #8894, #4135, #9089, #11750, #8008, #2099, #1286, #7113, #4068, #4200, #397, #6920, #11880, #10925, #2239, #337, #6107, #210, #7819, #6987, #11688, #3246, #2994, #9976, #10858, #5219, #146, #6861, #5159, #10042, #10988, #9026, #2168, #6040, #8075, #2037, #11942, #5917, #9851, #11812, #9786, #2296, #6168, #1098, #9915, #4964, #1165, #1353, #8826, #4003, #5976, #3058, #7946, #1225, #5093, #3305, #10333, #6350, #5472, #12248, #8136, #10218, #4504, #7173, #6228, #1530, #5532, #3367, #8322, #5404, #9275, #1414, #8379, #9152, #5342, #5281, #7237, #11050, #3435, #9338, #7297, #11110, #641, #11171, #3551, #1469, #7425, #6411, #2475, #579, #9213, #10273, #9396, #519, #6291, #2358, #2415, #4445, #12127, #12003, #11295, #12189, #3489, #11228, #7360, #4380, #10163, #2538, #1590, #2600, #6471, #1650, #4259, #10101, #8257, #458, #4320, #8197, #12067, #1831, #3863, #7739, #12434, #2787, #1766, #1709, #11605, #6778, #4630, #4757, #6649, #5836, #8689, #700, #12493, #10518, #6714, #5714, #9580, #5650, #887, #12373, #7550, #8623, #1298, #9461, #4567, #11542, #8440, #3673, #12309, #9647, #7676, #7487, #5590, #2851, #11358, #8500, #955, #2666, #6527, #11419, #2729, #10456, #9523, #821, #2019, #7802, #3232, #5011, #4946, #8945, #4182, #10708, #9898, #6025, #1212, #61, #9770, #5078, #7033, #4114, #7093, #11674, #10839, #8058, #9963, #7993, #11925, #257, #11862, #8875, #4050, #3169, #3927, #10907, #4884, #11736, #1148, #9708, #2222, #2152, #1024, #193, #2981, #3040, #1270, #10974, #6845, #320 ),
 .UNSPECIFIED., .F., .F. ) 
 B_SPLINE_CURVE_WITH_KNOTS ( ( 3, 2, 2, 2, 2, 2, 2, 2, 2, 2, 2, 2, 2, 2, 2, 2, 2, 2, 2, 2, 2, 2, 2, 2, 2, 2, 2, 2, 2, 2, 2, 2, 2, 2, 2, 2, 2, 2, 2, 2, 2, 2, 2, 2, 2, 2, 2, 2, 2, 2, 2, 2, 2, 2, 2, 2, 2, 2, 2, 2, 2, 2, 2, 2, 2, 2, 2, 2, 2, 2, 2, 2, 2, 2, 2, 2, 2, 2, 2, 2, 2, 2, 2, 2, 2, 2, 2, 2, 2, 2, 2, 2, 2, 2, 2, 2, 2, 2, 2, 2, 2, 2, 2, 2, 2, 2, 2, 2, 2, 2, 2, 2, 2, 2, 2, 2, 2, 2, 2, 2, 2, 2, 2, 2, 2, 2, 2, 2, 2, 2, 2, 2, 2, 2, 2, 2, 2, 2, 2, 2, 2, 2, 2, 2, 2, 2, 2, 2, 2, 2, 3 ),
 ( 0.000000000000000000, 0.006666666666666667095, 0.01333333333333333419, 0.02000000000000000042, 0.02666666666666666838, 0.03333333333333333287, 0.04000000000000000083, 0.04666666666666666879, 0.05333333333333333676, 0.05999999999999999778, 0.06666666666666666574, 0.07333333333333333370, 0.08000000000000000167, 0.08666666666666666963, 0.09333333333333333759, 0.1000000000000000056, 0.1066666666666666735, 0.1133333333333333276, 0.1199999999999999956, 0.1266666666666666774, 0.1333333333333333315, 0.1400000000000000133, 0.1466666666666666674, 0.1533333333333333215, 0.1600000000000000033, 0.1666666666666666574, 0.1733333333333333393, 0.1799999999999999933, 0.1866666666666666752, 0.1933333333333333293, 0.2000000000000000111, 0.2066666666666666652, 0.2133333333333333470, 0.2200000000000000011, 0.2266666666666666552, 0.2333333333333333370, 0.2399999999999999911, 0.2466666666666666730, 0.2533333333333333548, 0.2600000000000000089, 0.2666666666666666630, 0.2733333333333333171, 0.2800000000000000266, 0.2866666666666666807, 0.2933333333333333348, 0.2999999999999999889, 0.3066666666666666430, 0.3133333333333333526, 0.3200000000000000067, 0.3266666666666666607, 0.3333333333333333148, 0.3400000000000000244, 0.3466666666666666785, 0.3533333333333333326, 0.3599999999999999867, 0.3666666666666666408, 0.3733333333333333504, 0.3800000000000000044, 0.3866666666666666585, 0.3933333333333333126, 0.4000000000000000222, 0.4066666666666666763, 0.4133333333333333304, 0.4199999999999999845, 0.4266666666666666941, 0.4333333333333333481, 0.4400000000000000022, 0.4466666666666666563, 0.4533333333333333104, 0.4600000000000000200, 0.4666666666666666741, 0.4733333333333333282, 0.4799999999999999822, 0.4866666666666666918, 0.4933333333333333459, 0.5000000000000000000, 0.5066666666666667096, 0.5133333333333333082, 0.5200000000000000178, 0.5266666666666666163, 0.5333333333333333259, 0.5400000000000000355, 0.5466666666666666341, 0.5533333333333333437, 0.5600000000000000533, 0.5666666666666666519, 0.5733333333333333615, 0.5799999999999999600, 0.5866666666666666696, 0.5933333333333333792, 0.5999999999999999778, 0.6066666666666666874, 0.6133333333333332860, 0.6199999999999999956, 0.6266666666666667052, 0.6333333333333333037, 0.6400000000000000133, 0.6466666666666666119, 0.6533333333333333215, 0.6600000000000000311, 0.6666666666666666297, 0.6733333333333333393, 0.6800000000000000488, 0.6866666666666666474, 0.6933333333333333570, 0.6999999999999999556, 0.7066666666666666652, 0.7133333333333333748, 0.7199999999999999734, 0.7266666666666666829, 0.7333333333333332815, 0.7399999999999999911, 0.7466666666666667007, 0.7533333333333332993, 0.7600000000000000089, 0.7666666666666667185, 0.7733333333333333171, 0.7800000000000000266, 0.7866666666666666252, 0.7933333333333333348, 0.8000000000000000444, 0.8066666666666666430, 0.8133333333333333526, 0.8199999999999999512, 0.8266666666666666607, 0.8333333333333333703, 0.8399999999999999689, 0.8466666666666666785, 0.8533333333333333881, 0.8599999999999999867, 0.8666666666666666963, 0.8733333333333332948, 0.8800000000000000044, 0.8866666666666667140, 0.8933333333333333126, 0.9000000000000000222, 0.9066666666666666208, 0.9133333333333333304, 0.9200000000000000400, 0.9266666666666666385, 0.9333333333333333481, 0.9399999999999999467, 0.9466666666666666563, 0.9533333333333333659, 0.9599999999999999645, 0.9666666666666666741, 0.9733333333333333837, 0.9799999999999999822, 0.9866666666666666918, 0.9933333333333332904, 1.000000000000000000 ),
 .UNSPECIFIED. ) 
 CURVE ( )  GEOMETRIC_REPRESENTATION_ITEM ( )  RATIONAL_B_SPLINE_CURVE ( ( 1.000000000000000000, 0.9510565162951535312, 1.000000000000000000, 0.9510565162951535312, 1.000000000000000000, 0.9510565162951535312, 1.000000000000000000, 0.9510565162951535312, 1.000000000000000000, 0.9510565162951535312, 1.000000000000000000, 0.9510565162951535312, 1.000000000000000000, 0.9510565162951535312, 1.000000000000000000, 0.9510565162951535312, 1.000000000000000000, 0.9510565162951535312, 1.000000000000000000, 0.9510565162951535312, 1.000000000000000000, 0.9510565162951535312, 1.000000000000000000, 0.9510565162951535312, 1.000000000000000000, 0.9510565162951535312, 1.000000000000000000, 0.9510565162951535312, 1.000000000000000000, 0.9510565162951535312, 1.000000000000000000, 0.9510565162951535312, 1.000000000000000000, 0.9510565162951535312, 1.000000000000000000, 0.9510565162951535312, 1.000000000000000000, 0.9510565162951535312, 1.000000000000000000, 0.9510565162951535312, 1.000000000000000000, 0.9510565162951535312, 1.000000000000000000, 0.9510565162951535312, 1.000000000000000000, 0.9510565162951535312, 1.000000000000000000, 0.9510565162951535312, 1.000000000000000000, 0.9510565162951535312, 1.000000000000000000, 0.9510565162951535312, 1.000000000000000000, 0.9510565162951535312, 1.000000000000000000, 0.9510565162951535312, 1.000000000000000000, 0.9510565162951535312, 1.000000000000000000, 0.9510565162951535312, 1.000000000000000000, 0.9510565162951535312, 1.000000000000000000, 0.9510565162951535312, 1.000000000000000000, 0.9510565162951535312, 1.000000000000000000, 0.9510565162951535312, 1.000000000000000000, 0.9510565162951535312, 1.000000000000000000, 0.9510565162951535312, 1.000000000000000000, 0.9510565162951535312, 1.000000000000000000, 0.9510565162951535312, 1.000000000000000000, 0.9510565162951535312, 1.000000000000000000, 0.9510565162951535312, 1.000000000000000000, 0.9510565162951535312, 1.000000000000000000, 0.9510565162951535312, 1.000000000000000000, 0.9510565162951535312, 1.000000000000000000, 0.9510565162951535312, 1.000000000000000000, 0.9510565162951535312, 1.000000000000000000, 0.9510565162951535312, 1.000000000000000000, 0.9510565162951535312, 1.000000000000000000, 0.9510565162951535312, 1.000000000000000000, 0.9510565162951535312, 1.000000000000000000, 0.9510565162951535312, 1.000000000000000000, 0.9510565162951535312, 1.000000000000000000, 0.9510565162951535312, 1.000000000000000000, 0.9510565162951535312, 1.000000000000000000, 0.9510565162951535312, 1.000000000000000000, 0.9510565162951535312, 1.000000000000000000, 0.9510565162951535312, 1.000000000000000000, 0.9510565162951535312, 1.000000000000000000, 0.9510565162951535312, 1.000000000000000000, 0.9510565162951535312, 1.000000000000000000, 0.9510565162951535312, 1.000000000000000000, 0.9510565162951535312, 1.000000000000000000, 0.9510565162951535312, 1.000000000000000000, 0.9510565162951535312, 1.000000000000000000, 0.9510565162951535312, 1.000000000000000000, 0.9510565162951535312, 1.000000000000000000, 0.9510565162951535312, 1.000000000000000000, 0.9510565162951535312, 1.000000000000000000, 0.9510565162951535312, 1.000000000000000000, 0.9510565162951535312, 1.000000000000000000, 0.9510565162951535312, 1.000000000000000000, 0.9510565162951535312, 1.000000000000000000, 0.9510565162951535312, 1.000000000000000000, 0.9510565162951535312, 1.000000000000000000, 0.9510565162951535312, 1.000000000000000000, 0.9510565162951535312, 1.000000000000000000, 0.9510565162951535312, 1.000000000000000000, 0.9510565162951535312, 1.000000000000000000, 0.9510565162951535312, 1.000000000000000000, 0.9510565162951535312, 1.000000000000000000, 0.9510565162951535312, 1.000000000000000000, 0.9510565162951535312, 1.000000000000000000, 0.9510565162951535312, 1.000000000000000000, 0.9510565162951535312, 1.000000000000000000, 0.9510565162951535312, 1.000000000000000000, 0.9510565162951535312, 1.000000000000000000, 0.9510565162951535312, 1.000000000000000000, 0.9510565162951535312, 1.000000000000000000, 0.9510565162951535312, 1.000000000000000000, 0.9510565162951535312, 1.000000000000000000, 0.9510565162951535312, 1.000000000000000000, 0.9510565162951535312, 1.000000000000000000, 0.9510565162951535312, 1.000000000000000000, 0.9510565162951535312, 1.000000000000000000, 0.9510565162951535312, 1.000000000000000000, 0.9510565162951535312, 1.000000000000000000, 0.9510565162951535312, 1.000000000000000000, 0.9510565162951535312, 1.000000000000000000, 0.9510565162951535312, 1.000000000000000000, 0.9510565162951535312, 1.000000000000000000, 0.9510565162951535312, 1.000000000000000000, 0.9510565162951535312, 1.000000000000000000, 0.9510565162951535312, 1.000000000000000000, 0.9510565162951535312, 1.000000000000000000, 0.9510565162951535312, 1.000000000000000000, 0.9510565162951535312, 1.000000000000000000, 0.9510565162951535312, 1.000000000000000000, 0.9510565162951535312, 1.000000000000000000, 0.9510565162951535312, 1.000000000000000000, 0.9510565162951535312, 1.000000000000000000, 0.9510565162951535312, 1.000000000000000000, 0.9510565162951535312, 1.000000000000000000, 0.9510565162951535312, 1.000000000000000000, 0.9510565162951535312, 1.000000000000000000, 0.9510565162951535312, 1.000000000000000000, 0.9510565162951535312, 1.000000000000000000, 0.9510565162951535312, 1.000000000000000000, 0.9510565162951535312, 1.000000000000000000, 0.9510565162951535312, 1.000000000000000000, 0.9510565162951535312, 1.000000000000000000, 0.9510565162951535312, 1.000000000000000000, 0.9510565162951535312, 1.000000000000000000, 0.9510565162951535312, 1.000000000000000000, 0.9510565162951535312, 1.000000000000000000, 0.9510565162951535312, 1.000000000000000000, 0.9510565162951535312, 1.000000000000000000, 0.9510565162951535312, 1.000000000000000000, 0.9510565162951535312, 1.000000000000000000, 0.9510565162951535312, 1.000000000000000000, 0.9510565162951535312, 1.000000000000000000, 0.9510565162951535312, 1.000000000000000000, 0.9510565162951535312, 1.000000000000000000, 0.9510565162951535312, 1.000000000000000000, 0.9510565162951535312, 1.000000000000000000, 0.9510565162951535312, 1.000000000000000000, 0.9510565162951535312, 1.000000000000000000, 0.9510565162951535312, 1.000000000000000000, 0.9510565162951535312, 1.000000000000000000, 0.9510565162951535312, 1.000000000000000000, 0.9510565162951535312, 1.000000000000000000, 0.9510565162951535312, 1.000000000000000000, 0.9510565162951535312, 1.000000000000000000, 0.9510565162951535312, 1.000000000000000000, 0.9510565162951535312, 1.000000000000000000, 0.9510565162951535312, 1.000000000000000000, 0.9510565162951535312, 1.000000000000000000, 0.9510565162951535312, 1.000000000000000000, 0.9510565162951535312, 1.000000000000000000, 0.9510565162951535312, 1.000000000000000000, 0.9510565162951535312, 1.000000000000000000, 0.9510565162951535312, 1.000000000000000000 ) ) 
 REPRESENTATION_ITEM ( '' )  );
#3726=LINE ( 'NONE', #11536, #1340 ) ;
#3729=CARTESIAN_POINT ( 'NONE',  ( 49.99999999999998579, 22.00000000000000000, 152.2284161474004520 ) ) ;
#3733=CARTESIAN_POINT ( 'NONE',  ( 28.65000000109246514, 20.00000000000000355, 83.29316153445364534 ) ) ;
#3734=CARTESIAN_POINT ( 'NONE',  ( 42.57500000054623257, 15.71886984736413773, 84.90069139318163138 ) ) ;
#3736=CARTESIAN_POINT ( 'NONE',  ( 30.17500000054621978, 13.80429023900056507, 95.29460816699764791 ) ) ;
#3737=CARTESIAN_POINT ( 'NONE',  ( 27.89999999999998792, 22.43689772174679575, 98.29316153445363113 ) ) ;
#3738=( NAMED_UNIT ( * ) PLANE_ANGLE_UNIT ( ) SI_UNIT ( $, .RADIAN. ) );
#3739=CARTESIAN_POINT ( 'NONE',  ( 39.27500000054622120, 27.65831843345427998, 90.79316153445363113 ) ) ;
#3740=VERTEX_POINT ( 'NONE', #12386 ) ;
#3742=CARTESIAN_POINT ( 'NONE',  ( 20.35000000109246088, 13.62011893735971135, 86.15790661882942914 ) ) ;
#3748=CARTESIAN_POINT ( 'NONE',  ( 32.89999999999998437, 17.56310227825320425, 83.29316153445363113 ) ) ;
#3751=CARTESIAN_POINT ( 'NONE',  ( 44.87500000054622973, 20.00000000000000355, 83.50966788445364841 ) ) ;
#3754=DIRECTION ( 'NONE',  ( 1.000000000000000000, -0.000000000000000000, -0.000000000000000000 ) ) ;
#3755=CARTESIAN_POINT ( 'NONE',  ( 42.87500000054622262, 20.00000000000000355, 83.50966788445364841 ) ) ;
#3756=CARTESIAN_POINT ( 'NONE',  ( 45.79999999999999005, 24.40838939219354842, 96.86078899226572503 ) ) ;
#3758=CARTESIAN_POINT ( 'NONE',  ( 38.75000000109247367, 22.43689772174678509, 83.29316153445363113 ) ) ;
#3759=ORIENTED_EDGE ( 'NONE', *, *, #6426, .T. ) ;
#3760=CARTESIAN_POINT ( 'NONE',  ( 40.85000000109246088, 24.40838939219355197, 84.72553407664153724 ) ) ;
#3762=FACE_OUTER_BOUND ( 'NONE', #3606, .T. ) ;
#3764=AXIS2_PLACEMENT_3D ( 'NONE', #11012, #9878, #5122 ) ;
#3767=CARTESIAN_POINT ( 'NONE',  ( 31.45000000109246585, 24.40838939219354842, 96.86078899226572503 ) ) ;
#3772=VERTEX_POINT ( 'NONE', #8888 ) ;
#3775=CARTESIAN_POINT ( 'NONE',  ( 21.77500000054622831, 20.00000000000000355, 98.07665518445361386 ) ) ;
#3777=FACE_OUTER_BOUND ( 'NONE', #93, .T. ) ;
#3778=PLANE ( 'NONE',  #7112 ) ;
#3781=ORIENTED_EDGE ( 'NONE', *, *, #7695, .T. ) ;
#3785=( BOUNDED_CURVE ( )  B_SPLINE_CURVE ( 2, ( #3626, #8273, #2618, #6241, #10118, #6368, #1606, #6425, #1428, #5295, #5357 ),
 .UNSPECIFIED., .F., .F. ) 
 B_SPLINE_CURVE_WITH_KNOTS ( ( 3, 2, 2, 2, 2, 3 ),
 ( 0.9333333333333333481, 0.9399999999999999467, 0.9466666666666666563, 0.9533333333333333659, 0.9599999999999999645, 0.9666666666666666741 ),
 .UNSPECIFIED. ) 
 CURVE ( )  GEOMETRIC_REPRESENTATION_ITEM ( )  RATIONAL_B_SPLINE_CURVE ( ( 1.000000000000000000, 0.9510565162951535312, 1.000000000000000000, 0.9510565162951535312, 1.000000000000000000, 0.9510565162951535312, 1.000000000000000000, 0.9510565162951535312, 1.000000000000000000, 0.9510565162951535312, 1.000000000000000000 ) ) 
 REPRESENTATION_ITEM ( '' )  );
#3786=VECTOR ( 'NONE', #1135, 1000.000000000000000 ) ;
#3787=CARTESIAN_POINT ( 'NONE',  ( 21.77500000054622831, 20.00000000000000355, 98.07665518445361386 ) ) ;
#3793=LINE ( 'NONE', #7670, #1041 ) ;
#3794=ORIENTED_EDGE ( 'NONE', *, *, #5487, .T. ) ;
#3796=AXIS2_PLACEMENT_3D ( 'NONE', #3687, #3628, #7567 ) ;
#3799=CARTESIAN_POINT ( 'NONE',  ( 41.67500000054622689, 22.36655054427230027, 98.07665518445361386 ) ) ;
#3800=( BOUNDED_CURVE ( )  B_SPLINE_CURVE ( 3, ( #4565, #4502, #3671, #5529 ),
 .UNSPECIFIED., .F., .F. ) 
 B_SPLINE_CURVE_WITH_KNOTS ( ( 4, 4 ),
 ( 0.2699327958334041266, 1.570796326794896558 ),
 .UNSPECIFIED. ) 
 CURVE ( )  GEOMETRIC_REPRESENTATION_ITEM ( )  RATIONAL_B_SPLINE_CURVE ( ( 1.000000000000000000, 0.8638816171694810864, 0.8638816171694810864, 1.000000000000000000 ) ) 
 REPRESENTATION_ITEM ( '' )  );
#3802=CARTESIAN_POINT ( 'NONE',  ( 29.27500000054622475, 26.92701409722686634, 88.54243821818162985 ) ) ;
#3803=CARTESIAN_POINT ( 'NONE',  ( 29.99999999999998934, 20.00000000000000355, 98.29316153445363113 ) ) ;
#3804=EDGE_CURVE ( 'NONE', #1585, #4846, #4835, .T. ) ;
#3805=CARTESIAN_POINT ( 'NONE',  ( 31.87500000054622973, 17.63344945572769973, 98.07665518445361386 ) ) ;
#3807=CARTESIAN_POINT ( 'NONE',  ( -50.00000000000001421, 22.00000000000000000, 188.4007504869563263 ) ) ;
#3812=CARTESIAN_POINT ( 'NONE',  ( 42.25000000109246656, 12.86707612778636012, 88.47553407664152303 ) ) ;
#3815=CARTESIAN_POINT ( 'NONE',  ( -2.000000000000015543, 20.00000000000000355, 90.79316153445363113 ) ) ;
#3817=CARTESIAN_POINT ( 'NONE',  ( 44.97500000054621694, 22.36655054427230382, 83.50966788445364841 ) ) ;
#3820=CARTESIAN_POINT ( 'NONE',  ( 44.17500000054622689, 13.80429023900056507, 95.29460816699764791 ) ) ;
#3821=CARTESIAN_POINT ( 'NONE',  ( 21.07500000054622191, 24.28113015263587471, 84.90069139318163138 ) ) ;
#3822=CARTESIAN_POINT ( 'NONE',  ( 39.69999999999998863, 26.37988106264029398, 95.42841645007781892 ) ) ;
#3825=ORIENTED_EDGE ( 'NONE', *, *, #5822, .F. ) ;
#3826=CARTESIAN_POINT ( 'NONE',  ( 36.15000000109245804, 12.11403331821300533, 90.79316153445363113 ) ) ;
#3829=VECTOR ( 'NONE', #668, 1000.000000000000000 ) ;
#3830=ORIENTED_EDGE ( 'NONE', *, *, #598, .F. ) ;
#3831=EDGE_CURVE ( 'NONE', #9392, #11695, #11684, .T. ) ;
#3833=CARTESIAN_POINT ( 'NONE',  ( 31.25000000109246656, 27.13292387221364876, 93.11078899226573924 ) ) ;
#3834=CIRCLE ( 'NONE', #9319, 7.500000000000007105 ) ;
#3835=CARTESIAN_POINT ( 'NONE',  ( 26.65000000109246514, 20.00000000000000355, 83.29316153445364534 ) ) ;
#3836=VECTOR ( 'NONE', #12325, 1000.000000000000000 ) ;
#3837=CARTESIAN_POINT ( 'NONE',  ( 35.07500000054623257, 26.19570976099943493, 86.29171490190961435 ) ) ;
#3839=CARTESIAN_POINT ( 'NONE',  ( -50.00000000000001421, 0.000000000000000000, 69.99999999999998579 ) ) ;
#3842=CARTESIAN_POINT ( 'NONE',  ( 48.35000000109246088, 13.62011893735970958, 86.15790661882942914 ) ) ;
#3843=CARTESIAN_POINT ( 'NONE',  ( 48.27500000054622831, 13.07298590277314254, 93.04388485072563242 ) ) ;
#3846=CARTESIAN_POINT ( 'NONE',  ( 23.39999999999998792, 27.13292387221364876, 88.47553407664153724 ) ) ;
#3847=VERTEX_POINT ( 'NONE', #11876 ) ;
#3860=AXIS2_PLACEMENT_3D ( 'NONE', #4939, #187, #881 ) ;
#3863=CARTESIAN_POINT ( 'NONE',  ( 28.77500000054622831, 17.63344945572770328, 83.50966788445364841 ) ) ;
#3865=CARTESIAN_POINT ( 'NONE',  ( 40.27500000054622831, 12.34168156654572357, 90.79316153445363113 ) ) ;
#3866=CARTESIAN_POINT ( 'NONE',  ( 24.57500000054622191, 13.80429023900056684, 86.29171490190961435 ) ) ;
#3867=CARTESIAN_POINT ( 'NONE',  ( 25.19999999999998508, 24.40838939219355197, 84.72553407664153724 ) ) ;
#3869=CARTESIAN_POINT ( 'NONE',  ( 34.17500000054622689, 13.07298590277314254, 93.04388485072563242 ) ) ;
#3873=EDGE_LOOP ( 'NONE', ( #1093, #95, #6888, #10917, #12199, #1219, #3957, #4192, #176, #9922, #27, #7249, #1890, #3065, #8872, #4330, #11997, #8265, #6433, #11806, #2633, #8670, #7385, #2230, #8226, #2860, #12409, #2942, #3054, #12415, #172, #3706, #327 ) ) ;
#3875=ORIENTED_EDGE ( 'NONE', *, *, #3200, .T. ) ;
#3877=DIRECTION ( 'NONE',  ( 1.000000000000000000, -0.000000000000000000, -0.000000000000000000 ) ) ;
#3879=CARTESIAN_POINT ( 'NONE',  ( 43.57500000054623257, 26.19570976099943849, 95.29460816699764791 ) ) ;
#3881=CARTESIAN_POINT ( 'NONE',  ( -50.00000000000001421, 0.000000000000000000, 69.99999999999998579 ) ) ;
#3882=CARTESIAN_POINT ( 'NONE',  ( 46.97500000054621694, 22.36655054427230382, 83.50966788445364841 ) ) ;
#3883=CARTESIAN_POINT ( 'NONE',  ( 48.19999999999998863, 15.59161060780645691, 96.86078899226572503 ) ) ;
#3884=CARTESIAN_POINT ( 'NONE',  ( 45.59999999999998721, 27.13292387221364876, 93.11078899226573924 ) ) ;
#3887=EDGE_CURVE ( 'NONE', #574, #7418, #11746, .T. ) ;
#3888=CARTESIAN_POINT ( 'NONE',  ( 30.95000000109246585, 26.37988106264029398, 86.15790661882942914 ) ) ;
#3890=EDGE_LOOP ( 'NONE', ( #12214, #4515, #12121, #8375, #4256 ) ) ;
#3891=EDGE_CURVE ( 'NONE', #8158, #589, #7549, .T. ) ;
#3894=EDGE_CURVE ( 'NONE', #3772, #513, #10150, .T. ) ;
#3896=CARTESIAN_POINT ( 'NONE',  ( 38.97500000054622404, 24.28113015263587471, 84.90069139318163138 ) ) ;
#3897=CARTESIAN_POINT ( 'NONE',  ( 38.37500000054622973, 12.34168156654572535, 90.79316153445363113 ) ) ;
#3898=CARTESIAN_POINT ( 'NONE',  ( 35.05000000109246372, 27.13292387221364876, 88.47553407664153724 ) ) ;
#3902=CARTESIAN_POINT ( 'NONE',  ( 49.55000000109246372, 22.43689772174679575, 98.29316153445363113 ) ) ;
#3908=EDGE_LOOP ( 'NONE', ( #4928, #5155, #6598, #5137, #3177, #8373 ) ) ;
#3910=ORIENTED_EDGE ( 'NONE', *, *, #3894, .T. ) ;
#3911=CARTESIAN_POINT ( 'NONE',  ( 42.95000000109246940, 26.37988106264029398, 86.15790661882942914 ) ) ;
#3913=CARTESIAN_POINT ( 'NONE',  ( -31.89339828220176898, 12.50000000000000711, 140.6066017177981848 ) ) ;
#3914=LINE ( 'NONE', #8737, #8013 ) ;
#3921=ORIENTED_EDGE ( 'NONE', *, *, #7766, .F. ) ;
#3922=CARTESIAN_POINT ( 'NONE',  ( 36.95000000109246230, 26.37988106264029398, 86.15790661882942914 ) ) ;
#3925=VECTOR ( 'NONE', #3960, 1000.000000000000000 ) ;
#3927=CARTESIAN_POINT ( 'NONE',  ( 21.37500000054622262, 27.65831843345427998, 90.79316153445363113 ) ) ;
#3928=CARTESIAN_POINT ( 'NONE',  ( 49.57500000054621836, 26.19570976099943493, 95.29460816699764791 ) ) ;
#3929=CARTESIAN_POINT ( 'NONE',  ( 40.17500000054623399, 13.07298590277314254, 93.04388485072563242 ) ) ;
#3930=CARTESIAN_POINT ( 'NONE',  ( 19.87500000054622262, 20.00000000000000355, 98.07665518445361386 ) ) ;
#3931=CARTESIAN_POINT ( 'NONE',  ( 25.09999999999998366, 22.43689772174679575, 83.29316153445363113 ) ) ;
#3933=CARTESIAN_POINT ( 'NONE',  ( 36.17500000054622689, 13.07298590277314254, 93.04388485072563242 ) ) ;
#3936=ORIENTED_EDGE ( 'NONE', *, *, #939, .F. ) ;
#3939=VERTEX_POINT ( 'NONE', #3243 ) ;
#3943=CARTESIAN_POINT ( 'NONE',  ( 45.47500000054622404, 26.92701409722686634, 93.04388485072563242 ) ) ;
#3944=CARTESIAN_POINT ( 'NONE',  ( 40.15000000109245804, 12.11403331821300533, 90.79316153445363113 ) ) ;
#3947=CARTESIAN_POINT ( 'NONE',  ( 44.89999999999998437, 17.56310227825321135, 83.29316153445363113 ) ) ;
#3949=CARTESIAN_POINT ( 'NONE',  ( 40.89999999999998437, 17.56310227825320425, 83.29316153445363113 ) ) ;
#3953=ADVANCED_FACE ( 'NONE', ( #1525 ), #10213, .F. ) ;
#3954=CARTESIAN_POINT ( 'NONE',  ( 32.75000000109245946, 22.43689772174679575, 83.29316153445363113 ) ) ;
#3956=ORIENTED_EDGE ( 'NONE', *, *, #1801, .T. ) ;
#3957=ORIENTED_EDGE ( 'NONE', *, *, #3417, .F. ) ;
#3960=DIRECTION ( 'NONE',  ( 1.000000000000000000, 0.000000000000000000, 0.000000000000000000 ) ) ;
#3961=CARTESIAN_POINT ( 'NONE',  ( 39.97500000054622404, 15.71886984736413417, 96.68563167572563088 ) ) ;
#3962=CARTESIAN_POINT ( 'NONE',  ( 34.47500000054622404, 13.07298590277314432, 88.54243821818161564 ) ) ;
#3965=CARTESIAN_POINT ( 'NONE',  ( 34.65000000109246514, 20.00000000000000355, 83.29316153445364534 ) ) ;
#3966=VERTEX_POINT ( 'NONE', #6223 ) ;
#3970=CARTESIAN_POINT ( 'NONE',  ( 34.99999999999998579, 20.00000000000000000, 137.5000000000000000 ) ) ;
#3971=EDGE_LOOP ( 'NONE', ( #11474, #4080, #5367, #4409 ) ) ;
#3973=EDGE_CURVE ( 'NONE', #652, #11262, #3302, .T. ) ;
#3975=LINE ( 'NONE', #1011, #9668 ) ;
#3976=CARTESIAN_POINT ( 'NONE',  ( 9.685019593098569857, 22.50223202666526134, 97.86792408789433750 ) ) ;
#3978=FACE_OUTER_BOUND ( 'NONE', #6820, .T. ) ;
#3979=FACE_OUTER_BOUND ( 'NONE', #6761, .T. ) ;
#3980=AXIS2_PLACEMENT_3D ( 'NONE', #6274, #1692, #11277 ) ;
#3981=CARTESIAN_POINT ( 'NONE',  ( -24.10660171779822747, 69.50000000000000000, 151.2467237978899846 ) ) ;
#3982=CARTESIAN_POINT ( 'NONE',  ( 41.87500000054622262, 17.63344945572769973, 98.07665518445361386 ) ) ;
#3983=DIRECTION ( 'NONE',  ( 1.000000000000000000, -0.000000000000000000, -0.000000000000000000 ) ) ;
#3984=ORIENTED_EDGE ( 'NONE', *, *, #1388, .F. ) ;
#3985=CARTESIAN_POINT ( 'NONE',  ( 36.75000000109246656, 22.43689772174676023, 83.29316153445360271 ) ) ;
#3986=PRODUCT_CONTEXT ( 'NONE', #8218, 'mechanical' ) ;
#3988=CARTESIAN_POINT ( 'NONE',  ( 46.09999999999998010, 17.56310227825323977, 98.29316153445364534 ) ) ;
#3989=DIRECTION ( 'NONE',  ( 1.000000000000000000, 0.000000000000000000, 0.000000000000000000 ) ) ;
#3990=CARTESIAN_POINT ( 'NONE',  ( 30.27500000054622831, 12.34168156654572357, 90.79316153445363113 ) ) ;
#3992=CARTESIAN_POINT ( 'NONE',  ( 20.79999999999999005, 15.59161060780646046, 84.72553407664153724 ) ) ;
#3993=DIRECTION ( 'NONE',  ( 1.000000000000000000, -0.000000000000000000, -0.000000000000000000 ) ) ;
#3994=CARTESIAN_POINT ( 'NONE',  ( 30.67500000054622689, 17.63344945572770328, 83.50966788445364841 ) ) ;
#3996=PLANE ( 'NONE',  #9125 ) ;
#4002=CYLINDRICAL_SURFACE ( 'NONE', #11913, 7.499999999999992895 ) ;
#4003=CARTESIAN_POINT ( 'NONE',  ( 35.87500000054622973, 20.00000000000000355, 98.07665518445361386 ) ) ;
#4005=FACE_OUTER_BOUND ( 'NONE', #485, .T. ) ;
#4006=CARTESIAN_POINT ( 'NONE',  ( 41.87500000054622262, 20.00000000000000355, 98.07665518445361386 ) ) ;
#4007=CARTESIAN_POINT ( 'NONE',  ( 44.99999999999999289, 20.00000000000000355, 83.29316153445364534 ) ) ;
#4009=EDGE_CURVE ( 'NONE', #3211, #7244, #7167, .T. ) ;
#4012=CARTESIAN_POINT ( 'NONE',  ( 33.45000000109246940, 24.40838939219354842, 96.86078899226572503 ) ) ;
#4013=FACE_OUTER_BOUND ( 'NONE', #5018, .T. ) ;
#4019=DIRECTION ( 'NONE',  ( 0.000000000000000000, 0.000000000000000000, -1.000000000000000000 ) ) ;
#4022=CARTESIAN_POINT ( 'NONE',  ( 30.17500000054623044, 13.07298590277314254, 93.04388485072563242 ) ) ;
#4023=CARTESIAN_POINT ( 'NONE',  ( 34.57500000054621125, 13.80429023900056684, 86.29171490190961435 ) ) ;
#4027=DIRECTION ( 'NONE',  ( 0.000000000000000000, 0.000000000000000000, -1.000000000000000000 ) ) ;
#4029=CARTESIAN_POINT ( 'NONE',  ( 47.45000000109246230, 24.40838939219354842, 96.86078899226572503 ) ) ;
#4034=ORIENTED_EDGE ( 'NONE', *, *, #8993, .T. ) ;
#4035=AXIS2_PLACEMENT_3D ( 'NONE', #1743, #5624, #800 ) ;
#4036=DIRECTION ( 'NONE',  ( -1.000000000000000000, 0.000000000000000000, -0.000000000000000000 ) ) ;
#4037=CARTESIAN_POINT ( 'NONE',  ( 36.99999999999995026, 0.000000000000000000, 69.99999999999998579 ) ) ;
#4039=CARTESIAN_POINT ( 'NONE',  ( 9.796548249817144338, 22.02198220144915553, 98.01984945353935075 ) ) ;
#4040=CARTESIAN_POINT ( 'NONE',  ( -2.000000000000015543, 20.00000000000000355, 83.29316153445364534 ) ) ;
#4045=CARTESIAN_POINT ( 'NONE',  ( 40.57500000054623257, 15.71886984736413773, 84.90069139318163138 ) ) ;
#4046=LINE ( 'NONE', #9765, #10538 ) ;
#4047=ORIENTED_EDGE ( 'NONE', *, *, #3361, .T. ) ;
#4049=EDGE_CURVE ( 'NONE', #4582, #5275, #4890, .T. ) ;
#4050=CARTESIAN_POINT ( 'NONE',  ( 21.57500000054622191, 26.19570976099943849, 95.29460816699764791 ) ) ;
#4052=CARTESIAN_POINT ( 'NONE',  ( 36.27500000054622831, 12.34168156654572357, 90.79316153445363113 ) ) ;
#4053=CARTESIAN_POINT ( 'NONE',  ( 21.67500000054622333, 24.28113015263587116, 96.68563167572563088 ) ) ;
#4054=CARTESIAN_POINT ( 'NONE',  ( 23.89999999999998792, 22.43689772174679575, 98.29316153445363113 ) ) ;
#4055=DIRECTION ( 'NONE',  ( 0.000000000000000000, 0.000000000000000000, -1.000000000000000000 ) ) ;
#4056=CARTESIAN_POINT ( 'NONE',  ( 32.17500000054622689, 13.07298590277314254, 93.04388485072563242 ) ) ;
#4057=VERTEX_POINT ( 'NONE', #7044 ) ;
#4058=AXIS2_PLACEMENT_3D ( 'NONE', #11412, #2662, #1522 ) ;
#4059=PRODUCT_DEFINITION_SHAPE ( 'NONE', 'NONE',  #7910 ) ;
#4064=VERTEX_POINT ( 'NONE', #10159 ) ;
#4068=CARTESIAN_POINT ( 'NONE',  ( 39.97500000054622404, 17.63344945572769973, 98.07665518445361386 ) ) ;
#4069=CARTESIAN_POINT ( 'NONE',  ( -50.00000000000001421, 20.00000000000000000, 145.0000000000000000 ) ) ;
#4071=CARTESIAN_POINT ( 'NONE',  ( 39.77500000054621410, 22.36655054427230027, 98.07665518445361386 ) ) ;
#4072=CARTESIAN_POINT ( 'NONE',  ( 40.39999999999999147, 12.86707612778636012, 93.11078899226572503 ) ) ;
#4074=CARTESIAN_POINT ( 'NONE',  ( -20.00000000000001776, 20.00000000000000000, 137.5000000000000000 ) ) ;
#4076=CARTESIAN_POINT ( 'NONE',  ( 32.65000000109246514, 20.00000000000000355, 83.29316153445364534 ) ) ;
#4080=ORIENTED_EDGE ( 'NONE', *, *, #5795, .T. ) ;
#4082=CARTESIAN_POINT ( 'NONE',  ( 25.45000000109246230, 24.40838939219354842, 96.86078899226572503 ) ) ;
#4084=EDGE_CURVE ( 'NONE', #1716, #3396, #3800, .T. ) ;
#4085=DIRECTION ( 'NONE',  ( 0.000000000000000000, -1.000000000000000000, -0.000000000000000000 ) ) ;
#4086=CARTESIAN_POINT ( 'NONE',  ( 29.27500000054622831, 27.65831843345427998, 90.79316153445363113 ) ) ;
#4087=CARTESIAN_POINT ( 'NONE',  ( 32.47500000054621694, 13.07298590277314432, 88.54243821818161564 ) ) ;
#4090=CARTESIAN_POINT ( 'NONE',  ( 34.25000000109245946, 12.86707612778636012, 88.47553407664152303 ) ) ;
#4092=CARTESIAN_POINT ( 'NONE',  ( 48.27500000054622831, 13.07298590277314254, 93.04388485072563242 ) ) ;
#4093=CARTESIAN_POINT ( 'NONE',  ( 48.45000000109246940, 15.59161060780646046, 84.72553407664153724 ) ) ;
#4095=CARTESIAN_POINT ( 'NONE',  ( 30.65000000109246514, 20.00000000000000355, 83.29316153445364534 ) ) ;
#4102=CARTESIAN_POINT ( 'NONE',  ( 7.415375966899784288, 26.71411643570026229, 94.16958235496709051 ) ) ;
#4105=DIRECTION ( 'NONE',  ( 1.000000000000000000, -0.000000000000000000, -0.000000000000000000 ) ) ;
#4107=CARTESIAN_POINT ( 'NONE',  ( 44.57500000054622546, 15.71886984736413773, 84.90069139318163138 ) ) ;
#4108=ADVANCED_FACE ( 'NONE', ( #6525 ), #4690, .F. ) ;
#4114=CARTESIAN_POINT ( 'NONE',  ( 22.67500000054622333, 15.71886984736413773, 84.90069139318163138 ) ) ;
#4115=CARTESIAN_POINT ( 'NONE',  ( 49.07500000054622546, 24.28113015263587471, 84.90069139318163138 ) ) ;
#4116=AXIS2_PLACEMENT_3D ( 'NONE', #7652, #11585, #12411 ) ;
#4117=CARTESIAN_POINT ( 'NONE',  ( 34.97500000054623115, 24.28113015263587471, 84.90069139318163138 ) ) ;
#4118=CARTESIAN_POINT ( 'NONE',  ( 21.97500000054622049, 17.63344945572769973, 98.07665518445361386 ) ) ;
#4119=CARTESIAN_POINT ( 'NONE',  ( 21.39999999999998792, 27.13292387221364876, 88.47553407664153724 ) ) ;
#4121=CARTESIAN_POINT ( 'NONE',  ( 24.17500000054622689, 13.07298590277314254, 93.04388485072563242 ) ) ;
#4122=ORIENTED_EDGE ( 'NONE', *, *, #1627, .T. ) ;
#4123=EDGE_CURVE ( 'NONE', #6453, #1585, #1706, .T. ) ;
#4126=VERTEX_POINT ( 'NONE', #3729 ) ;
#4127=DIRECTION ( 'NONE',  ( 0.000000000000000000, 0.000000000000000000, -1.000000000000000000 ) ) ;
#4131=CIRCLE ( 'NONE', #11219, 10.00000000000000355 ) ;
#4134=EDGE_CURVE ( 'NONE', #8484, #1332, #10394, .T. ) ;
#4135=CARTESIAN_POINT ( 'NONE',  ( 40.67500000054622689, 15.71886984736413773, 84.90069139318163138 ) ) ;
#4136=PLANE ( 'NONE',  #9184 ) ;
#4138=CARTESIAN_POINT ( 'NONE',  ( 41.47500000054623115, 26.92701409722686634, 93.04388485072563242 ) ) ;
#4139=CARTESIAN_POINT ( 'NONE',  ( 43.99999999999999289, 20.00000000000000355, 98.29316153445363113 ) ) ;
#4140=CARTESIAN_POINT ( 'NONE',  ( 45.47500000054623825, 26.19570976099943493, 95.29460816699764791 ) ) ;
#4141=ORIENTED_EDGE ( 'NONE', *, *, #3831, .F. ) ;
#4143=CARTESIAN_POINT ( 'NONE',  ( 25.85000000109246443, 15.59161060780645691, 96.86078899226572503 ) ) ;
#4146=( BOUNDED_CURVE ( )  B_SPLINE_CURVE ( 2, ( #2734, #6719, #10714, #893, #9654, #961, #11612, #8751, #1963, #4891, #6593 ),
 .UNSPECIFIED., .F., .F. ) 
 B_SPLINE_CURVE_WITH_KNOTS ( ( 3, 2, 2, 2, 2, 3 ),
 ( 0.5000000000000000000, 0.5066666666666667096, 0.5133333333333333082, 0.5200000000000000178, 0.5266666666666666163, 0.5333333333333333259 ),
 .UNSPECIFIED. ) 
 CURVE ( )  GEOMETRIC_REPRESENTATION_ITEM ( )  RATIONAL_B_SPLINE_CURVE ( ( 1.000000000000000000, 0.9510565162951535312, 1.000000000000000000, 0.9510565162951535312, 1.000000000000000000, 0.9510565162951535312, 1.000000000000000000, 0.9510565162951535312, 1.000000000000000000, 0.9510565162951535312, 1.000000000000000000 ) ) 
 REPRESENTATION_ITEM ( '' )  );
#4151=CARTESIAN_POINT ( 'NONE',  ( -50.00000000000001421, 20.00000000000000000, 137.5000000000000000 ) ) ;
#4153=CARTESIAN_POINT ( 'NONE',  ( 28.47500000054622404, 13.80429023900056684, 86.29171490190961435 ) ) ;
#4154=CARTESIAN_POINT ( 'NONE',  ( 28.67500000054622689, 15.71886984736413773, 84.90069139318163138 ) ) ;
#4157=CARTESIAN_POINT ( 'NONE',  ( -27.49999999999999645, 20.00000000000000355, 99.99999999999997158 ) ) ;
#4159=CARTESIAN_POINT ( 'NONE',  ( 47.55000000109247082, 22.43689772174679575, 98.29316153445363113 ) ) ;
#4160=EDGE_LOOP ( 'NONE', ( #12079, #11105, #6997, #9283, #11649, #1574, #8132, #4437, #11447 ) ) ;
#4169=CYLINDRICAL_SURFACE ( 'NONE', #2980, 7.500000000000000000 ) ;
#4171=CARTESIAN_POINT ( 'NONE',  ( 6.614416936062160524, 27.49996590649457673, 90.53406983787975548 ) ) ;
#4172=CARTESIAN_POINT ( 'NONE',  ( -6.999999999999999112, 55.00000000000000000, 147.8533255156883399 ) ) ;
#4173=LINE ( 'NONE', #11725, #4957 ) ;
#4174=CARTESIAN_POINT ( 'NONE',  ( -50.00000000000001421, 22.00000000000000000, 152.2284161474004520 ) ) ;
#4177=CARTESIAN_POINT ( 'NONE',  ( 45.47500000054623825, 26.19570976099943493, 95.29460816699764791 ) ) ;
#4179=ORIENTED_EDGE ( 'NONE', *, *, #7811, .T. ) ;
#4182=CARTESIAN_POINT ( 'NONE',  ( 23.57500000054622191, 26.19570976099943849, 95.29460816699764791 ) ) ;
#4183=CARTESIAN_POINT ( 'NONE',  ( 42.37500000054621552, 12.34168156654572535, 90.79316153445363113 ) ) ;
#4184=VECTOR ( 'NONE', #4491, 1000.000000000000000 ) ;
#4185=CARTESIAN_POINT ( 'NONE',  ( 31.87500000054622973, 17.63344945572769973, 98.07665518445361386 ) ) ;
#4186=CARTESIAN_POINT ( 'NONE',  ( 19.97500000054622404, 17.63344945572769973, 98.07665518445361386 ) ) ;
#4187=LINE ( 'NONE', #6339, #11532 ) ;
#4189=CARTESIAN_POINT ( 'NONE',  ( 24.57500000054622902, 15.71886984736413773, 84.90069139318163138 ) ) ;
#4190=ORIENTED_EDGE ( 'NONE', *, *, #5188, .F. ) ;
#4191=DIRECTION ( 'NONE',  ( 1.000000000000000000, 0.000000000000000000, 0.000000000000000000 ) ) ;
#4192=ORIENTED_EDGE ( 'NONE', *, *, #2114, .F. ) ;
#4194=CARTESIAN_POINT ( 'NONE',  ( 38.59999999999998721, 12.86707612778636012, 88.47553407664152303 ) ) ;
#4196=EDGE_CURVE ( 'NONE', #6070, #5277, #8620, .T. ) ;
#4199=CARTESIAN_POINT ( 'NONE',  ( 0.000000000000000000, 0.000000000000000000, 69.99999999999998579 ) ) ;
#4200=CARTESIAN_POINT ( 'NONE',  ( 39.87500000054622262, 20.00000000000000355, 98.07665518445361386 ) ) ;
#4203=CARTESIAN_POINT ( 'NONE',  ( 26.39999999999998792, 12.86707612778636012, 93.11078899226572503 ) ) ;
#4204=CARTESIAN_POINT ( 'NONE',  ( 37.97500000054621694, 17.63344945572769973, 98.07665518445361386 ) ) ;
#4205=CARTESIAN_POINT ( 'NONE',  ( 40.59999999999998721, 12.86707612778636012, 88.47553407664152303 ) ) ;
#4207=CARTESIAN_POINT ( 'NONE',  ( 47.87500000054622973, 17.63344945572769973, 98.07665518445361386 ) ) ;
#4208=ORIENTED_EDGE ( 'NONE', *, *, #12157, .F. ) ;
#4209=CARTESIAN_POINT ( 'NONE',  ( 26.15000000109246159, 12.11403331821300533, 90.79316153445363113 ) ) ;
#4211=ORIENTED_EDGE ( 'NONE', *, *, #2572, .F. ) ;
#4215=ORIENTED_EDGE ( 'NONE', *, *, #5834, .T. ) ;
#4218=CARTESIAN_POINT ( 'NONE',  ( 41.15000000109246514, 27.88596668178699645, 90.79316153445363113 ) ) ;
#4219=CARTESIAN_POINT ( 'NONE',  ( 25.49999999999998934, 27.88596668178699645, 90.79316153445363113 ) ) ;
#4220=CARTESIAN_POINT ( 'NONE',  ( 32.97500000054622404, 24.28113015263587471, 84.90069139318163138 ) ) ;
#4221=CARTESIAN_POINT ( 'NONE',  ( 30.17500000054621978, 13.80429023900056507, 95.29460816699764791 ) ) ;
#4223=( BOUNDED_CURVE ( )  B_SPLINE_CURVE ( 3, ( #5185, #2266, #1251, #6133 ),
 .UNSPECIFIED., .F., .F. ) 
 B_SPLINE_CURVE_WITH_KNOTS ( ( 4, 4 ),
 ( 1.570796326794896558, 3.141592653589793116 ),
 .UNSPECIFIED. ) 
 CURVE ( )  GEOMETRIC_REPRESENTATION_ITEM ( )  RATIONAL_B_SPLINE_CURVE ( ( 1.000000000000000000, 0.8047378541243649375, 0.8047378541243649375, 1.000000000000000000 ) ) 
 REPRESENTATION_ITEM ( '' )  );
#4224=LINE ( 'NONE', #12025, #8476 ) ;
#4227=CARTESIAN_POINT ( 'NONE',  ( 41.15000000109247225, 27.88596668178699645, 90.79316153445363113 ) ) ;
#4230=ORIENTED_EDGE ( 'NONE', *, *, #9017, .F. ) ;
#4237=DIRECTION ( 'NONE',  ( 0.000000000000000000, 1.000000000000000000, 0.000000000000000000 ) ) ;
#4239=DIRECTION ( 'NONE',  ( 0.000000000000000000, 0.000000000000000000, -1.000000000000000000 ) ) ;
#4243=VECTOR ( 'NONE', #853, 1000.000000000000000 ) ;
#4245=ADVANCED_FACE ( 'NONE', ( #638, #8376 ), #12247, .F. ) ;
#4247=CARTESIAN_POINT ( 'NONE',  ( 46.27500000054622831, 13.07298590277314254, 93.04388485072563242 ) ) ;
#4248=CARTESIAN_POINT ( 'NONE',  ( 36.07500000054622546, 13.80429023900056507, 95.29460816699764791 ) ) ;
#4249=CARTESIAN_POINT ( 'NONE',  ( 6.629289121864024636, 12.51307322058950611, 91.30463553460788262 ) ) ;
#4250=CARTESIAN_POINT ( 'NONE',  ( 45.65000000109247225, 20.00000000000000355, 98.29316153445363113 ) ) ;
#4252=CARTESIAN_POINT ( 'NONE',  ( 27.27500000054622475, 27.65831843345427998, 90.79316153445363113 ) ) ;
#4254=DIRECTION ( 'NONE',  ( 0.000000000000000000, 0.000000000000000000, -1.000000000000000000 ) ) ;
#4256=ORIENTED_EDGE ( 'NONE', *, *, #5253, .F. ) ;
#4257=CARTESIAN_POINT ( 'NONE',  ( 38.89999999999999147, 17.56310227825319359, 83.29316153445364534 ) ) ;
#4259=CARTESIAN_POINT ( 'NONE',  ( 29.57500000054621836, 26.19570976099943849, 95.29460816699764791 ) ) ;
#4260=DIRECTION ( 'NONE',  ( 0.000000000000000000, 0.000000000000000000, -1.000000000000000000 ) ) ;
#4263=CARTESIAN_POINT ( 'NONE',  ( 38.27500000054622831, 13.07298590277314254, 93.04388485072563242 ) ) ;
#4264=CARTESIAN_POINT ( 'NONE',  ( 36.29999999999997584, 13.62011893735971135, 95.42841645007781892 ) ) ;
#4266=CARTESIAN_POINT ( 'NONE',  ( 43.47500000054623115, 26.19570976099943493, 95.29460816699764791 ) ) ;
#4267=ORIENTED_EDGE ( 'NONE', *, *, #11999, .T. ) ;
#4268=CARTESIAN_POINT ( 'NONE',  ( 27.45000000109246585, 24.40838939219354842, 96.86078899226572503 ) ) ;
#4272=EDGE_LOOP ( 'NONE', ( #5387, #7660, #330, #7515 ) ) ;
#4273=DIRECTION ( 'NONE',  ( 1.000000000000000000, -0.000000000000000000, -0.000000000000000000 ) ) ;
#4275=CARTESIAN_POINT ( 'NONE',  ( 40.65000000109246514, 20.00000000000000355, 83.29316153445364534 ) ) ;
#4276=CARTESIAN_POINT ( 'NONE',  ( 32.07500000054623257, 13.80429023900056507, 95.29460816699764791 ) ) ;
#4277=CARTESIAN_POINT ( 'NONE',  ( 22.87500000054622618, 20.00000000000000355, 83.50966788445364841 ) ) ;
#4281=VERTEX_POINT ( 'NONE', #12490 ) ;
#4282=AXIS2_PLACEMENT_3D ( 'NONE', #4804, #8669, #12539 ) ;
#4283=CARTESIAN_POINT ( 'NONE',  ( 43.55000000109246372, 22.43689772174679575, 98.29316153445363113 ) ) ;
#4291=DIRECTION ( 'NONE',  ( 1.000000000000000000, -0.000000000000000000, -0.000000000000000000 ) ) ;
#4296=CARTESIAN_POINT ( 'NONE',  ( 20.27158385259951956, 18.00000000000000355, 169.9999999999999716 ) ) ;
#4300=CARTESIAN_POINT ( 'NONE',  ( -6.999999999999999112, 69.50000000000000000, 146.8533255156881978 ) ) ;
#4305=CARTESIAN_POINT ( 'NONE',  ( 45.87500000054622973, 20.00000000000000355, 98.07665518445361386 ) ) ;
#4306=CARTESIAN_POINT ( 'NONE',  ( 24.57500000054622902, 15.71886984736413773, 84.90069139318163138 ) ) ;
#4307=CARTESIAN_POINT ( 'NONE',  ( 9.959687983327881966, 18.97177336558172911, 83.34667569529023012 ) ) ;
#4308=AXIS2_PLACEMENT_3D ( 'NONE', #5012, #3989, #11606 ) ;
#4309=CARTESIAN_POINT ( 'NONE',  ( 33.19999999999998863, 24.40838939219355197, 84.72553407664153724 ) ) ;
#4310=DIRECTION ( 'NONE',  ( 1.000000000000000000, -0.000000000000000000, -0.000000000000000000 ) ) ;
#4311=CARTESIAN_POINT ( 'NONE',  ( 24.87500000054622618, 22.36655054427230382, 83.50966788445364841 ) ) ;
#4312=ORIENTED_EDGE ( 'NONE', *, *, #2844, .T. ) ;
#4314=EDGE_CURVE ( 'NONE', #4704, #3374, #6258, .T. ) ;
#4317=ORIENTED_EDGE ( 'NONE', *, *, #7463, .F. ) ;
#4319=VECTOR ( 'NONE', #6959, 1000.000000000000000 ) ;
#4320=CARTESIAN_POINT ( 'NONE',  ( 29.17500000054622333, 26.19570976099943849, 86.29171490190961435 ) ) ;
#4322=CARTESIAN_POINT ( 'NONE',  ( 44.57500000054622546, 15.71886984736413773, 84.90069139318163138 ) ) ;
#4323=CARTESIAN_POINT ( 'NONE',  ( 32.47500000054621694, 13.07298590277314432, 88.54243821818161564 ) ) ;
#4324=CARTESIAN_POINT ( 'NONE',  ( 37.39999999999999147, 27.13292387221364876, 88.47553407664153724 ) ) ;
#4325=CARTESIAN_POINT ( 'NONE',  ( 44.07500000054623968, 13.80429023900056507, 95.29460816699764791 ) ) ;
#4326=ORIENTED_EDGE ( 'NONE', *, *, #5218, .F. ) ;
#4327=VECTOR ( 'NONE', #12405, 1000.000000000000000 ) ;
#4328=CARTESIAN_POINT ( 'NONE',  ( 22.55000000109246017, 17.56310227825321135, 83.29316153445363113 ) ) ;
#4330=ORIENTED_EDGE ( 'NONE', *, *, #647, .F. ) ;
#4340=DIRECTION ( 'NONE',  ( 1.000000000000000000, -0.000000000000000000, -0.000000000000000000 ) ) ;
#4342=CARTESIAN_POINT ( 'NONE',  ( 26.97500000054622760, 24.28113015263587471, 84.90069139318163138 ) ) ;
#4343=CARTESIAN_POINT ( 'NONE',  ( 27.17500000054621978, 26.19570976099943493, 86.29171490190961435 ) ) ;
#4349=CARTESIAN_POINT ( 'NONE',  ( 41.75000000109247367, 17.56310227825320425, 98.29316153445363113 ) ) ;
#4351=ORIENTED_EDGE ( 'NONE', *, *, #261, .F. ) ;
#4354=AXIS2_PLACEMENT_3D ( 'NONE', #8479, #8663, #6507 ) ;
#4362=DIRECTION ( 'NONE',  ( 1.000000000000000000, 0.000000000000000000, 0.000000000000000000 ) ) ;
#4365=CARTESIAN_POINT ( 'NONE',  ( -20.00000000000001776, 20.00000000000000000, 137.5000000000000000 ) ) ;
#4370=CARTESIAN_POINT ( 'NONE',  ( 41.97500000054623115, 17.63344945572769973, 98.07665518445361386 ) ) ;
#4371=CARTESIAN_POINT ( 'NONE',  ( 27.97500000054623115, 15.71886984736413417, 96.68563167572563088 ) ) ;
#4372=CARTESIAN_POINT ( 'NONE',  ( 36.99999999999995026, 0.000000000000000000, 69.99999999999998579 ) ) ;
#4373=DIRECTION ( 'NONE',  ( 0.000000000000000000, -0.000000000000000000, -1.000000000000000000 ) ) ;
#4375=FACE_OUTER_BOUND ( 'NONE', #609, .T. ) ;
#4377=CARTESIAN_POINT ( 'NONE',  ( 27.49999999999999645, 20.00000000000000355, 99.99999999999997158 ) ) ;
#4378=CARTESIAN_POINT ( 'NONE',  ( 38.79999999999999005, 15.59161060780646046, 84.72553407664153724 ) ) ;
#4380=CARTESIAN_POINT ( 'NONE',  ( 30.27500000054622475, 13.07298590277314254, 93.04388485072563242 ) ) ;
#4382=CARTESIAN_POINT ( 'NONE',  ( 44.77500000054623541, 20.00000000000000355, 83.50966788445364841 ) ) ;
#4383=CARTESIAN_POINT ( 'NONE',  ( 36.07500000054622546, 15.71886984736413417, 96.68563167572563088 ) ) ;
#4384=CARTESIAN_POINT ( 'NONE',  ( 36.59999999999998721, 12.86707612778636012, 88.47553407664152303 ) ) ;
#4386=CARTESIAN_POINT ( 'NONE',  ( 48.57500000054623257, 15.71886984736413773, 84.90069139318163138 ) ) ;
#4388=CARTESIAN_POINT ( 'NONE',  ( 24.55000000109246017, 17.56310227825321135, 83.29316153445363113 ) ) ;
#4396=CARTESIAN_POINT ( 'NONE',  ( 36.65000000109245804, 20.00000000000000355, 83.29316153445364534 ) ) ;
#4400=CARTESIAN_POINT ( 'NONE',  ( 26.57500000054622902, 15.71886984736413773, 84.90069139318163138 ) ) ;
#4401=CARTESIAN_POINT ( 'NONE',  ( 23.27500000054622475, 26.92701409722686634, 88.54243821818162985 ) ) ;
#4402=CARTESIAN_POINT ( 'NONE',  ( 19.93750000027310421, 20.00000000000000355, 98.18490835945361539 ) ) ;
#4404=ORIENTED_EDGE ( 'NONE', *, *, #7849, .F. ) ;
#4405=CARTESIAN_POINT ( 'NONE',  ( 45.55000000109247082, 22.43689772174679575, 98.29316153445363113 ) ) ;
#4408=CARTESIAN_POINT ( 'NONE',  ( 30.35000000109246088, 13.62011893735970958, 86.15790661882942914 ) ) ;
#4409=ORIENTED_EDGE ( 'NONE', *, *, #8138, .F. ) ;
#4411=LINE ( 'NONE', #10364, #10125 ) ;
#4413=DIRECTION ( 'NONE',  ( 0.000000000000000000, 0.000000000000000000, -1.000000000000000000 ) ) ;
#4414=VECTOR ( 'NONE', #10357, 1000.000000000000000 ) ;
#4416=DIRECTION ( 'NONE',  ( -1.000000000000000000, 0.000000000000000000, 0.000000000000000000 ) ) ;
#4423=AXIS2_PLACEMENT_3D ( 'NONE', #1639, #10445, #10510 ) ;
#4427=CARTESIAN_POINT ( 'NONE',  ( 38.67500000054622689, 15.71886984736413773, 84.90069139318163138 ) ) ;
#4428=CARTESIAN_POINT ( 'NONE',  ( 27.77500000054622831, 20.00000000000000355, 98.07665518445361386 ) ) ;
#4429=EDGE_CURVE ( 'NONE', #8586, #10212, #10905, .T. ) ;
#4430=VECTOR ( 'NONE', #12347, 1000.000000000000000 ) ;
#4431=CARTESIAN_POINT ( 'NONE',  ( 9.796987274755800001, 17.98000013482726089, 83.56587684317791798 ) ) ;
#4432=CARTESIAN_POINT ( 'NONE',  ( 45.15000000109246514, 27.88596668178699645, 90.79316153445363113 ) ) ;
#4433=CARTESIAN_POINT ( 'NONE',  ( 35.99999999999999289, 20.00000000000000355, 98.29316153445363113 ) ) ;
#4434=FACE_OUTER_BOUND ( 'NONE', #73, .T. ) ;
#4437=ORIENTED_EDGE ( 'NONE', *, *, #5792, .F. ) ;
#4441=ADVANCED_FACE ( 'NONE', ( #9874 ), #1186, .F. ) ;
#4445=CARTESIAN_POINT ( 'NONE',  ( 31.07500000054622546, 24.28113015263587471, 84.90069139318163138 ) ) ;
#4447=CARTESIAN_POINT ( 'NONE',  ( 44.27500000054622120, 12.34168156654572357, 90.79316153445363113 ) ) ;
#4448=CARTESIAN_POINT ( 'NONE',  ( 30.97500000054622760, 22.36655054427230382, 83.50966788445364841 ) ) ;
#4449=CARTESIAN_POINT ( 'NONE',  ( 37.79999999999998295, 24.40838939219354842, 96.86078899226572503 ) ) ;
#4451=CARTESIAN_POINT ( 'NONE',  ( 40.37500000054622973, 13.07298590277314432, 88.54243821818161564 ) ) ;
#4452=ORIENTED_EDGE ( 'NONE', *, *, #1262, .T. ) ;
#4453=CARTESIAN_POINT ( 'NONE',  ( 45.97500000054623115, 15.71886984736413417, 96.68563167572563088 ) ) ;
#4455=ORIENTED_EDGE ( 'NONE', *, *, #9568, .F. ) ;
#4456=DIRECTION ( 'NONE',  ( 0.000000000000000000, 0.000000000000000000, -1.000000000000000000 ) ) ;
#4457=ORIENTED_EDGE ( 'NONE', *, *, #9017, .T. ) ;
#4461=CARTESIAN_POINT ( 'NONE',  ( 31.95000000109245875, 13.62011893735970958, 95.42841645007781892 ) ) ;
#4462=CARTESIAN_POINT ( 'NONE',  ( 26.37500000054622973, 13.07298590277314432, 88.54243821818161564 ) ) ;
#4463=CARTESIAN_POINT ( 'NONE',  ( 22.27500000054622120, 13.07298590277314254, 93.04388485072563242 ) ) ;
#4466=ORIENTED_EDGE ( 'NONE', *, *, #6134, .F. ) ;
#4467=CARTESIAN_POINT ( 'NONE',  ( 45.15000000109245804, 27.88596668178699645, 90.79316153445363113 ) ) ;
#4472=EDGE_CURVE ( 'NONE', #2741, #5074, #11928, .T. ) ;
#4474=EDGE_CURVE ( 'NONE', #2895, #136, #8115, .T. ) ;
#4478=CYLINDRICAL_SURFACE ( 'NONE', #11827, 7.499999999999992895 ) ;
#4484=CARTESIAN_POINT ( 'NONE',  ( 27.49999999999999645, 20.00000000000000355, 170.0000119999999697 ) ) ;
#4489=EDGE_CURVE ( 'NONE', #5074, #10297, #5524, .T. ) ;
#4491=DIRECTION ( 'NONE',  ( 1.000000000000000000, -0.000000000000000000, -0.000000000000000000 ) ) ;
#4492=CARTESIAN_POINT ( 'NONE',  ( 36.97500000054623115, 22.36655054427230382, 83.50966788445364841 ) ) ;
#4493=CARTESIAN_POINT ( 'NONE',  ( 24.97500000054622760, 24.28113015263587471, 84.90069139318163138 ) ) ;
#4494=CARTESIAN_POINT ( 'NONE',  ( 7.619081503294689028, 13.51451987764450990, 94.58903075352336032 ) ) ;
#4496=ADVANCED_FACE ( 'NONE', ( #9684 ), #11709, .F. ) ;
#4502=CARTESIAN_POINT ( 'NONE',  ( 33.79382810696422013, 14.62220435867159551, 151.2938281069642130 ) ) ;
#4504=CARTESIAN_POINT ( 'NONE',  ( 34.57500000054622546, 13.80429023900056684, 86.29171490190961435 ) ) ;
#4505=CARTESIAN_POINT ( 'NONE',  ( 27.25000000109246656, 27.13292387221364876, 93.11078899226573924 ) ) ;
#4506=CARTESIAN_POINT ( 'NONE',  ( 47.67500000054622689, 22.36655054427230027, 98.07665518445361386 ) ) ;
#4507=CARTESIAN_POINT ( 'NONE',  ( 34.47500000054622404, 13.07298590277314432, 88.54243821818161564 ) ) ;
#4508=CARTESIAN_POINT ( 'NONE',  ( 34.59999999999999432, 12.86707612778636012, 88.47553407664152303 ) ) ;
#4511=CARTESIAN_POINT ( 'NONE',  ( 38.47500000054621694, 13.80429023900056684, 86.29171490190961435 ) ) ;
#4512=ORIENTED_EDGE ( 'NONE', *, *, #7204, .T. ) ;
#4513=CARTESIAN_POINT ( 'NONE',  ( 20.45000000109246585, 15.59161060780646046, 84.72553407664153724 ) ) ;
#4515=ORIENTED_EDGE ( 'NONE', *, *, #3310, .T. ) ;
#4517=ORIENTED_EDGE ( 'NONE', *, *, #1269, .T. ) ;
#4521=CARTESIAN_POINT ( 'NONE',  ( 20.27158385259951956, 18.00000000000000355, 152.2284161474004520 ) ) ;
#4522=CARTESIAN_POINT ( 'NONE',  ( -21.20617189303578343, 14.62220435867159551, 151.2938281069642130 ) ) ;
#4523=CARTESIAN_POINT ( 'NONE',  ( 19.99999999999998579, 20.00000000000000355, 98.29316153445363113 ) ) ;
#4524=CARTESIAN_POINT ( 'NONE',  ( 22.97500000054622760, 24.28113015263587471, 84.90069139318163138 ) ) ;
#4525=CARTESIAN_POINT ( 'NONE',  ( 27.87500000054622262, 20.00000000000000355, 98.07665518445361386 ) ) ;
#4527=CARTESIAN_POINT ( 'NONE',  ( -2.000000000000015543, 20.00000000000000355, 90.79316153445363113 ) ) ;
#4528=CARTESIAN_POINT ( 'NONE',  ( 39.55000000109245661, 22.43689772174681707, 98.29316153445361692 ) ) ;
#4531=CARTESIAN_POINT ( 'NONE',  ( 38.65000000109246514, 20.00000000000000355, 83.29316153445364534 ) ) ;
#4532=CARTESIAN_POINT ( 'NONE',  ( 0.000000000000000000, 22.00000000000000000, 169.9999999999999716 ) ) ;
#4537=AXIS2_PLACEMENT_3D ( 'NONE', #9247, #551, #4413 ) ;
#4539=CARTESIAN_POINT ( 'NONE',  ( 29.89999999999998437, 22.43689772174679575, 98.29316153445363113 ) ) ;
#4542=CARTESIAN_POINT ( 'NONE',  ( 27.89999999999998792, 22.43689772174679575, 98.29316153445363113 ) ) ;
#4543=CARTESIAN_POINT ( 'NONE',  ( 42.69999999999998153, 13.62011893735970958, 86.15790661882942914 ) ) ;
#4545=CARTESIAN_POINT ( 'NONE',  ( 49.37500000054622973, 27.65831843345427998, 90.79316153445363113 ) ) ;
#4546=FACE_OUTER_BOUND ( 'NONE', #8542, .T. ) ;
#4547=AXIS2_PLACEMENT_3D ( 'NONE', #11123, #11186, #4036 ) ;
#4550=( BOUNDED_CURVE ( )  B_SPLINE_CURVE ( 2, ( #2631, #12281, #10362, #12093, #8349, #3334, #7199, #12215, #9242, #3517, #2506 ),
 .UNSPECIFIED., .F., .F. ) 
 B_SPLINE_CURVE_WITH_KNOTS ( ( 3, 2, 2, 2, 2, 3 ),
 ( 0.06666666666666672125, 0.07333333333333338921, 0.08000000000000007105, 0.08666666666666673902, 0.09333333333333342086, 0.1000000000000000888 ),
 .UNSPECIFIED. ) 
 CURVE ( )  GEOMETRIC_REPRESENTATION_ITEM ( )  RATIONAL_B_SPLINE_CURVE ( ( 0.9999999999999995559, 0.9510565162951539753, 1.000000000000000000, 0.9510565162951535312, 1.000000000000000000, 0.9510565162951535312, 1.000000000000000000, 0.9510565162951535312, 1.000000000000000000, 0.9510565162951529761, 1.000000000000000666 ) ) 
 REPRESENTATION_ITEM ( '' )  );
#4552=CARTESIAN_POINT ( 'NONE',  ( 20.00000000000003908, 20.00000000000000000, 137.5000000000000000 ) ) ;
#4553=CARTESIAN_POINT ( 'NONE',  ( 34.77500000054622831, 20.00000000000000355, 83.50966788445364841 ) ) ;
#4554=CARTESIAN_POINT ( 'NONE',  ( 36.67500000054622689, 15.71886984736413773, 84.90069139318163138 ) ) ;
#4555=AXIS2_PLACEMENT_3D ( 'NONE', #12039, #5252, #10136 ) ;
#4556=CARTESIAN_POINT ( 'NONE',  ( 28.57500000054622902, 15.71886984736413773, 84.90069139318163138 ) ) ;
#4561=CARTESIAN_POINT ( 'NONE',  ( 31.89999999999998437, 22.43689772174679575, 98.29316153445363113 ) ) ;
#4562=EDGE_CURVE ( 'NONE', #527, #5212, #8272, .T. ) ;
#4565=CARTESIAN_POINT ( 'NONE',  ( 34.72841614740047333, 18.00000000000000355, 152.2284161474004520 ) ) ;
#4567=CARTESIAN_POINT ( 'NONE',  ( 26.17500000054622689, 13.80429023900056507, 95.29460816699764791 ) ) ;
#4568=CARTESIAN_POINT ( 'NONE',  ( 26.65000000109246514, 20.00000000000000355, 83.29316153445364534 ) ) ;
#4569=VECTOR ( 'NONE', #7668, 1000.000000000000000 ) ;
#4570=CARTESIAN_POINT ( 'NONE',  ( 48.37500000054622973, 13.07298590277314432, 88.54243821818161564 ) ) ;
#4571=CARTESIAN_POINT ( 'NONE',  ( 32.67500000054622689, 15.71886984736413773, 84.90069139318163138 ) ) ;
#4572=CARTESIAN_POINT ( 'NONE',  ( 28.89999999999998437, 17.56310227825321135, 83.29316153445363113 ) ) ;
#4575=CARTESIAN_POINT ( 'NONE',  ( 36.67500000054623399, 17.63344945572770328, 83.50966788445364841 ) ) ;
#4578=CARTESIAN_POINT ( 'NONE',  ( 20.55000000109246372, 17.56310227825321135, 83.29316153445363113 ) ) ;
#4579=LINE ( 'NONE', #10283, #2244 ) ;
#4582=VERTEX_POINT ( 'NONE', #9811 ) ;
#4584=CARTESIAN_POINT ( 'NONE',  ( -50.00000000000001421, 22.00000000000000000, 152.2284161474004520 ) ) ;
#4588=CARTESIAN_POINT ( 'NONE',  ( 26.07500000054622902, 13.80429023900056507, 95.29460816699764791 ) ) ;
#4589=CARTESIAN_POINT ( 'NONE',  ( 21.67500000054622333, 24.28113015263587116, 96.68563167572563088 ) ) ;
#4592=EDGE_CURVE ( 'NONE', #5728, #10127, #8847, .T. ) ;
#4595=CARTESIAN_POINT ( 'NONE',  ( 39.85000000109246798, 15.59161060780645691, 96.86078899226572503 ) ) ;
#4596=CARTESIAN_POINT ( 'NONE',  ( 23.99999999999998579, 20.00000000000000355, 98.29316153445363113 ) ) ;
#4597=ORIENTED_EDGE ( 'NONE', *, *, #9414, .F. ) ;
#4603=CARTESIAN_POINT ( 'NONE',  ( -2.000000000000015543, 20.00000000000000355, 98.29316153445363113 ) ) ;
#4606=CARTESIAN_POINT ( 'NONE',  ( -6.999999999999999112, 92.00000000000000000, 69.99999999999998579 ) ) ;
#4607=CARTESIAN_POINT ( 'NONE',  ( 48.57500000054622546, 13.80429023900056684, 86.29171490190961435 ) ) ;
#4612=EDGE_LOOP ( 'NONE', ( #2688, #6512 ) ) ;
#4613=CARTESIAN_POINT ( 'NONE',  ( 43.45000000109246230, 24.40838939219354842, 96.86078899226572503 ) ) ;
#4615=CARTESIAN_POINT ( 'NONE',  ( 37.47500000054622404, 26.92701409722686634, 93.04388485072563242 ) ) ;
#4616=CARTESIAN_POINT ( 'NONE',  ( 20.07500000054622546, 13.80429023900056507, 95.29460816699764791 ) ) ;
#4617=CARTESIAN_POINT ( 'NONE',  ( 49.99999999999998579, 40.00000000000000000, 69.99999999999998579 ) ) ;
#4618=CARTESIAN_POINT ( 'NONE',  ( -50.00000000000001421, 69.50000000000000000, 146.8533255156881978 ) ) ;
#4621=( BOUNDED_CURVE ( )  B_SPLINE_CURVE ( 2, ( #6121, #9990, #412, #1302, #5173, #4218, #8090, #11956, #2311, #6180, #4275 ),
 .UNSPECIFIED., .F., .F. ) 
 B_SPLINE_CURVE_WITH_KNOTS ( ( 3, 2, 2, 2, 2, 3 ),
 ( 0.2666666666666666630, 0.2733333333333333171, 0.2800000000000000266, 0.2866666666666666807, 0.2933333333333333348, 0.2999999999999999889 ),
 .UNSPECIFIED. ) 
 CURVE ( )  GEOMETRIC_REPRESENTATION_ITEM ( )  RATIONAL_B_SPLINE_CURVE ( ( 1.000000000000000000, 0.9510565162951535312, 1.000000000000000000, 0.9510565162951535312, 1.000000000000000000, 0.9510565162951535312, 1.000000000000000000, 0.9510565162951535312, 1.000000000000000000, 0.9510565162951535312, 1.000000000000000000 ) ) 
 REPRESENTATION_ITEM ( '' )  );
#4625=DIRECTION ( 'NONE',  ( 0.000000000000000000, 0.000000000000000000, -1.000000000000000000 ) ) ;
#4626=EDGE_CURVE ( 'NONE', #8571, #8548, #2917, .T. ) ;
#4630=CARTESIAN_POINT ( 'NONE',  ( 27.97500000054622404, 17.63344945572769973, 98.07665518445361386 ) ) ;
#4632=CARTESIAN_POINT ( 'NONE',  ( 37.67500000054622689, 22.36655054427230027, 98.07665518445361386 ) ) ;
#4633=CARTESIAN_POINT ( 'NONE',  ( 28.57500000054622191, 13.80429023900056684, 86.29171490190961435 ) ) ;
#4634=CARTESIAN_POINT ( 'NONE',  ( 28.29999999999998650, 13.62011893735971135, 95.42841645007781892 ) ) ;
#4635=CARTESIAN_POINT ( 'NONE',  ( 40.47500000054622404, 13.80429023900056684, 86.29171490190961435 ) ) ;
#4637=CARTESIAN_POINT ( 'NONE',  ( 20.25000000109246301, 12.86707612778636012, 88.47553407664152303 ) ) ;
#4639=ORIENTED_EDGE ( 'NONE', *, *, #6839, .T. ) ;
#4644=DIRECTION ( 'NONE',  ( 1.000000000000000000, -0.000000000000000000, -0.000000000000000000 ) ) ;
#4645=CYLINDRICAL_SURFACE ( 'NONE', #1805, 7.499999999999992895 ) ;
#4647=CARTESIAN_POINT ( 'NONE',  ( 42.37500000054621552, 12.34168156654572357, 90.79316153445363113 ) ) ;
#4649=ADVANCED_FACE ( 'NONE', ( #6129 ), #3329, .F. ) ;
#4650=CARTESIAN_POINT ( 'NONE',  ( 43.57500000054623257, 26.19570976099943493, 95.29460816699764791 ) ) ;
#4651=CARTESIAN_POINT ( 'NONE',  ( 47.29999999999998295, 26.37988106264029398, 86.15790661882942914 ) ) ;
#4656=CARTESIAN_POINT ( 'NONE',  ( 36.55000000109247082, 17.56310227825321135, 83.29316153445363113 ) ) ;
#4657=CARTESIAN_POINT ( 'NONE',  ( 24.19999999999998863, 15.59161060780645691, 96.86078899226572503 ) ) ;
#4663=CARTESIAN_POINT ( 'NONE',  ( 30.65000000109246514, 20.00000000000000355, 83.29316153445364534 ) ) ;
#4668=LINE ( 'NONE', #3839, #11127 ) ;
#4671=CARTESIAN_POINT ( 'NONE',  ( -50.00000000000001421, 40.00000000000000000, 69.99999999999998579 ) ) ;
#4672=EDGE_CURVE ( 'NONE', #1996, #58, #4224, .T. ) ;
#4674=CARTESIAN_POINT ( 'NONE',  ( 47.37500000054622973, 27.65831843345427998, 90.79316153445363113 ) ) ;
#4675=CARTESIAN_POINT ( 'NONE',  ( -2.000000000000015543, 20.00000000000000355, 98.29316153445363113 ) ) ;
#4677=ORIENTED_EDGE ( 'NONE', *, *, #6421, .F. ) ;
#4682=LINE ( 'NONE', #5575, #5620 ) ;
#4683=CARTESIAN_POINT ( 'NONE',  ( 20.37500000054622618, 13.07298590277314432, 88.54243821818161564 ) ) ;
#4684=CARTESIAN_POINT ( 'NONE',  ( 4.999999999999999112, 40.00000000000000000, 169.9999999999999716 ) ) ;
#4686=FACE_OUTER_BOUND ( 'NONE', #7090, .T. ) ;
#4687=LINE ( 'NONE', #8558, #4569 ) ;
#4690=CYLINDRICAL_SURFACE ( 'NONE', #8536, 7.500000000000000000 ) ;
#4692=CARTESIAN_POINT ( 'NONE',  ( 36.19999999999998863, 15.59161060780645691, 96.86078899226572503 ) ) ;
#4693=CARTESIAN_POINT ( 'NONE',  ( 36.67500000054622689, 17.63344945572770328, 83.50966788445364841 ) ) ;
#4694=CARTESIAN_POINT ( 'NONE',  ( 30.87500000054622618, 20.00000000000000355, 83.50966788445364841 ) ) ;
#4695=CARTESIAN_POINT ( 'NONE',  ( 30.49999999999998934, 12.11403331821300533, 90.79316153445363113 ) ) ;
#4696=CARTESIAN_POINT ( 'NONE',  ( 30.89999999999998437, 17.56310227825320425, 83.29316153445363113 ) ) ;
#4697=EDGE_CURVE ( 'NONE', #3463, #5153, #11962, .T. ) ;
#4698=CARTESIAN_POINT ( 'NONE',  ( 39.77500000054622831, 20.00000000000000355, 98.07665518445361386 ) ) ;
#4700=CARTESIAN_POINT ( 'NONE',  ( 20.15000000109246514, 12.11403331821300533, 90.79316153445363113 ) ) ;
#4702=ORIENTED_EDGE ( 'NONE', *, *, #2513, .T. ) ;
#4704=VERTEX_POINT ( 'NONE', #2261 ) ;
#4708=CARTESIAN_POINT ( 'NONE',  ( 41.97500000054623115, 17.63344945572769973, 98.07665518445361386 ) ) ;
#4709=CARTESIAN_POINT ( 'NONE',  ( 20.69999999999998508, 13.62011893735970958, 86.15790661882942914 ) ) ;
#4710=DIRECTION ( 'NONE',  ( 0.000000000000000000, -1.000000000000000000, -0.000000000000000000 ) ) ;
#4711=CARTESIAN_POINT ( 'NONE',  ( 42.97500000054622404, 22.36655054427230382, 83.50966788445364841 ) ) ;
#4712=CARTESIAN_POINT ( 'NONE',  ( 20.57500000054622546, 13.80429023900056684, 86.29171490190961435 ) ) ;
#4717=CARTESIAN_POINT ( 'NONE',  ( 34.55000000109247082, 17.56310227825321135, 83.29316153445363113 ) ) ;
#4719=ORIENTED_EDGE ( 'NONE', *, *, #1424, .T. ) ;
#4720=DIRECTION ( 'NONE',  ( 0.000000000000000000, 0.000000000000000000, 1.000000000000000000 ) ) ;
#4724=CARTESIAN_POINT ( 'NONE',  ( 20.27158385259951956, 22.00000000000000000, 169.9999999999999716 ) ) ;
#4726=EDGE_CURVE ( 'NONE', #8716, #9224, #5304, .T. ) ;
#4733=CARTESIAN_POINT ( 'NONE',  ( 48.77500000054623541, 17.63344945572770328, 83.50966788445364841 ) ) ;
#4734=ORIENTED_EDGE ( 'NONE', *, *, #3098, .F. ) ;
#4735=CARTESIAN_POINT ( 'NONE',  ( 45.75000000109247367, 17.56310227825317227, 98.29316153445361692 ) ) ;
#4736=VECTOR ( 'NONE', #10741, 1000.000000000000000 ) ;
#4737=CARTESIAN_POINT ( 'NONE',  ( -5.000000000000002665, 18.00000000000000355, 152.2284161474004520 ) ) ;
#4745=CARTESIAN_POINT ( 'NONE',  ( 22.17500000054622689, 13.07298590277314254, 93.04388485072563242 ) ) ;
#4747=AXIS2_PLACEMENT_3D ( 'NONE', #12024, #7193, #5736 ) ;
#4751=CARTESIAN_POINT ( 'NONE',  ( 25.75000000109246301, 17.56310227825320425, 98.29316153445363113 ) ) ;
#4753=ORIENTED_EDGE ( 'NONE', *, *, #12049, .T. ) ;
#4757=CARTESIAN_POINT ( 'NONE',  ( 27.87500000054622262, 20.00000000000000355, 98.07665518445361386 ) ) ;
#4759=CARTESIAN_POINT ( 'NONE',  ( 41.87500000054621552, 17.63344945572769973, 98.07665518445361386 ) ) ;
#4760=CARTESIAN_POINT ( 'NONE',  ( 26.87500000054622618, 20.00000000000000355, 83.50966788445364841 ) ) ;
#4761=CARTESIAN_POINT ( 'NONE',  ( 31.09999999999999076, 22.43689772174679575, 83.29316153445363113 ) ) ;
#4764=CARTESIAN_POINT ( 'NONE',  ( 33.57500000054623257, 24.28113015263587116, 96.68563167572563088 ) ) ;
#4765=ORIENTED_EDGE ( 'NONE', *, *, #10552, .F. ) ;
#4767=CARTESIAN_POINT ( 'NONE',  ( 41.97500000054623115, 15.71886984736413417, 96.68563167572563088 ) ) ;
#4771=ORIENTED_EDGE ( 'NONE', *, *, #11626, .F. ) ;
#4773=CARTESIAN_POINT ( 'NONE',  ( 32.39999999999998437, 12.86707612778636012, 93.11078899226572503 ) ) ;
#4776=CARTESIAN_POINT ( 'NONE',  ( 45.27500000054622831, 26.92701409722686634, 88.54243821818162985 ) ) ;
#4779=CARTESIAN_POINT ( 'NONE',  ( 45.37500000054622973, 27.65831843345427998, 90.79316153445363113 ) ) ;
#4780=CARTESIAN_POINT ( 'NONE',  ( 20.67500000054622689, 15.71886984736413773, 84.90069139318163138 ) ) ;
#4782=CARTESIAN_POINT ( 'NONE',  ( 49.57500000054623257, 24.28113015263587116, 96.68563167572563088 ) ) ;
#4784=CARTESIAN_POINT ( 'NONE',  ( 37.35000000109246088, 26.37988106264029398, 95.42841645007781892 ) ) ;
#4785=CARTESIAN_POINT ( 'NONE',  ( 23.99999999999998579, 20.00000000000000355, 98.29316153445363113 ) ) ;
#4786=ORIENTED_EDGE ( 'NONE', *, *, #764, .F. ) ;
#4787=FACE_OUTER_BOUND ( 'NONE', #8725, .T. ) ;
#4788=ORIENTED_EDGE ( 'NONE', *, *, #11212, .T. ) ;
#4790=CARTESIAN_POINT ( 'NONE',  ( 31.55000000109246727, 22.43689772174679575, 98.29316153445363113 ) ) ;
#4791=EDGE_CURVE ( 'NONE', #4846, #8548, #480, .T. ) ;
#4792=CARTESIAN_POINT ( 'NONE',  ( -2.000000000000015543, 20.00000000000000355, 98.29316153445363113 ) ) ;
#4794=CARTESIAN_POINT ( 'NONE',  ( 36.17500000054622689, 13.07298590277314254, 93.04388485072563242 ) ) ;
#4796=CARTESIAN_POINT ( 'NONE',  ( 27.09999999999998721, 22.43689772174683128, 83.29316153445365956 ) ) ;
#4799=CARTESIAN_POINT ( 'NONE',  ( 48.45000000109246940, 15.59161060780646046, 84.72553407664153724 ) ) ;
#4800=CARTESIAN_POINT ( 'NONE',  ( 49.47500000054623115, 26.92701409722686634, 93.04388485072563242 ) ) ;
#4804=CARTESIAN_POINT ( 'NONE',  ( -2.000000000000015543, 20.00000000000000355, 90.79316153445363113 ) ) ;
#4805=EDGE_LOOP ( 'NONE', ( #11057, #1481, #1658, #1558, #2002 ) ) ;
#4808=CARTESIAN_POINT ( 'NONE',  ( 21.89999999999998437, 22.43689772174679575, 98.29316153445363113 ) ) ;
#4813=CARTESIAN_POINT ( 'NONE',  ( 20.87500000054622618, 22.36655054427230382, 83.50966788445364841 ) ) ;
#4816=CARTESIAN_POINT ( 'NONE',  ( 25.65000000109246514, 20.00000000000000355, 98.29316153445363113 ) ) ;
#4822=( BOUNDED_CURVE ( )  B_SPLINE_CURVE ( 2, ( #913, #8403, #2559, #1790, #1854, #7573, #12273, #12455, #11441, #5677, #7510 ),
 .UNSPECIFIED., .F., .F. ) 
 B_SPLINE_CURVE_WITH_KNOTS ( ( 3, 2, 2, 2, 2, 3 ),
 ( 0.2666666666666666630, 0.2733333333333333171, 0.2800000000000000266, 0.2866666666666666807, 0.2933333333333333348, 0.2999999999999999889 ),
 .UNSPECIFIED. ) 
 CURVE ( )  GEOMETRIC_REPRESENTATION_ITEM ( )  RATIONAL_B_SPLINE_CURVE ( ( 1.000000000000000000, 0.9510565162951535312, 1.000000000000000000, 0.9510565162951535312, 1.000000000000000000, 0.9510565162951535312, 1.000000000000000000, 0.9510565162951535312, 1.000000000000000000, 0.9510565162951535312, 1.000000000000000000 ) ) 
 REPRESENTATION_ITEM ( '' )  );
#4825=CARTESIAN_POINT ( 'NONE',  ( 41.27500000054622831, 27.65831843345427998, 90.79316153445363113 ) ) ;
#4827=CARTESIAN_POINT ( 'NONE',  ( 27.37500000054622262, 27.65831843345427998, 90.79316153445363113 ) ) ;
#4828=CARTESIAN_POINT ( 'NONE',  ( 20.59999999999998721, 12.86707612778636012, 88.47553407664152303 ) ) ;
#4830=CARTESIAN_POINT ( 'NONE',  ( 35.67500000054623399, 22.36655054427230027, 98.07665518445361386 ) ) ;
#4832=EDGE_CURVE ( 'NONE', #5989, #12402, #12210, .T. ) ;
#4834=ORIENTED_EDGE ( 'NONE', *, *, #4474, .F. ) ;
#4835=LINE ( 'NONE', #8821, #2661 ) ;
#4838=CARTESIAN_POINT ( 'NONE',  ( 43.69999999999998863, 26.37988106264029398, 95.42841645007781892 ) ) ;
#4839=DIRECTION ( 'NONE',  ( 0.000000000000000000, 0.000000000000000000, -1.000000000000000000 ) ) ;
#4840=CARTESIAN_POINT ( 'NONE',  ( 45.17500000054621268, 26.19570976099943849, 86.29171490190961435 ) ) ;
#4842=CARTESIAN_POINT ( 'NONE',  ( 20.47500000054622404, 13.07298590277314432, 88.54243821818161564 ) ) ;
#4843=CARTESIAN_POINT ( 'NONE',  ( 39.39999999999999147, 27.13292387221364876, 88.47553407664153724 ) ) ;
#4846=VERTEX_POINT ( 'NONE', #6612 ) ;
#4847=CARTESIAN_POINT ( 'NONE',  ( 31.95000000109245875, 13.62011893735971135, 95.42841645007781892 ) ) ;
#4850=AXIS2_PLACEMENT_3D ( 'NONE', #793, #7832, #7645 ) ;
#4851=ORIENTED_EDGE ( 'NONE', *, *, #8252, .T. ) ;
#4855=AXIS2_PLACEMENT_3D ( 'NONE', #9928, #10055, #8972 ) ;
#4856=CARTESIAN_POINT ( 'NONE',  ( 38.87500000054623683, 22.36655054427230382, 83.50966788445364841 ) ) ;
#4857=CARTESIAN_POINT ( 'NONE',  ( 36.37500000054623683, 12.34168156654572535, 90.79316153445363113 ) ) ;
#4859=CARTESIAN_POINT ( 'NONE',  ( 34.05000000109246372, 12.86707612778636012, 93.11078899226572503 ) ) ;
#4860=ORIENTED_EDGE ( 'NONE', *, *, #4791, .F. ) ;
#4865=EDGE_CURVE ( 'NONE', #3559, #7152, #12456, .T. ) ;
#4866=CARTESIAN_POINT ( 'NONE',  ( -50.00000000000001421, 22.00000000000000000, 152.2284161474004520 ) ) ;
#4873=CARTESIAN_POINT ( 'NONE',  ( 10.00000000000000355, 20.00000000000000355, 83.29316153445363113 ) ) ;
#4874=DIRECTION ( 'NONE',  ( 0.000000000000000000, 1.000000000000000000, 0.000000000000000000 ) ) ;
#4879=ORIENTED_EDGE ( 'NONE', *, *, #5104, .F. ) ;
#4884=CARTESIAN_POINT ( 'NONE',  ( 21.17500000054622689, 26.19570976099943849, 86.29171490190961435 ) ) ;
#4885=CARTESIAN_POINT ( 'NONE',  ( 49.27500000054622120, 26.92701409722686634, 88.54243821818162985 ) ) ;
#4887=CARTESIAN_POINT ( 'NONE',  ( 41.07500000054622546, 26.19570976099943849, 86.29171490190961435 ) ) ;
#4888=CARTESIAN_POINT ( 'NONE',  ( 26.57500000054622191, 13.80429023900056684, 86.29171490190961435 ) ) ;
#4889=CARTESIAN_POINT ( 'NONE',  ( 22.49999999999998934, 12.11403331821300533, 90.79316153445363113 ) ) ;
#4890=CIRCLE ( 'NONE', #1246, 10.00000000000000355 ) ;
#4891=CARTESIAN_POINT ( 'NONE',  ( 34.10000000000000142, 17.56310227825320425, 98.29316153445363113 ) ) ;
#4892=CARTESIAN_POINT ( 'NONE',  ( 31.67500000054622689, 22.36655054427230027, 98.07665518445361386 ) ) ;
#4896=CARTESIAN_POINT ( 'NONE',  ( 49.25000000109246656, 27.13292387221364876, 93.11078899226573924 ) ) ;
#4897=ORIENTED_EDGE ( 'NONE', *, *, #9100, .T. ) ;
#4898=SHAPE_REPRESENTATION_RELATIONSHIP ( 'NONE' , 'NONE' ,  #7408, #7483 ) ;
#4899=CARTESIAN_POINT ( 'NONE',  ( 32.19999999999999574, 15.59161060780645691, 96.86078899226572503 ) ) ;
#4900=DIRECTION ( 'NONE',  ( 1.000000000000000000, -0.000000000000000000, -0.000000000000000000 ) ) ;
#4902=CARTESIAN_POINT ( 'NONE',  ( 46.07500000054622546, 15.71886984736413417, 96.68563167572563088 ) ) ;
#4903=PLANE ( 'NONE',  #4930 ) ;
#4904=EDGE_CURVE ( 'NONE', #7736, #1411, #5553, .T. ) ;
#4906=CARTESIAN_POINT ( 'NONE',  ( 45.07500000054622546, 24.28113015263587471, 84.90069139318163138 ) ) ;
#4907=CARTESIAN_POINT ( 'NONE',  ( 42.29999999999998295, 13.62011893735971135, 95.42841645007781892 ) ) ;
#4908=CARTESIAN_POINT ( 'NONE',  ( 45.29999999999999005, 26.37988106264029398, 86.15790661882942914 ) ) ;
#4911=CARTESIAN_POINT ( 'NONE',  ( 33.75000000109246656, 17.56310227825320425, 98.29316153445363113 ) ) ;
#4913=ORIENTED_EDGE ( 'NONE', *, *, #9568, .T. ) ;
#4915=ORIENTED_EDGE ( 'NONE', *, *, #11465, .F. ) ;
#4919=CARTESIAN_POINT ( 'NONE',  ( 36.77500000054622831, 20.00000000000000355, 83.50966788445364841 ) ) ;
#4920=CARTESIAN_POINT ( 'NONE',  ( 30.57500000054622191, 13.80429023900056684, 86.29171490190961435 ) ) ;
#4921=AXIS2_PLACEMENT_3D ( 'NONE', #10102, #8076, #7114 ) ;
#4927=CARTESIAN_POINT ( 'NONE',  ( 46.65000000109246514, 20.00000000000000355, 83.29316153445364534 ) ) ;
#4928=ORIENTED_EDGE ( 'NONE', *, *, #189, .F. ) ;
#4929=ORIENTED_EDGE ( 'NONE', *, *, #10015, .T. ) ;
#4930=AXIS2_PLACEMENT_3D ( 'NONE', #8763, #1099, #3306 ) ;
#4931=LINE ( 'NONE', #8927, #1554 ) ;
#4932=CARTESIAN_POINT ( 'NONE',  ( 8.248483781669884607, 25.66706883268630079, 85.85796419627257592 ) ) ;
#4933=CARTESIAN_POINT ( 'NONE',  ( 37.59999999999998721, 27.13292387221364876, 93.11078899226573924 ) ) ;
#4937=CARTESIAN_POINT ( 'NONE',  ( 26.55000000109246372, 17.56310227825324333, 83.29316153445360271 ) ) ;
#4939=CARTESIAN_POINT ( 'NONE',  ( -28.50000000000001066, 77.00000000000000000, 166.8533255156881694 ) ) ;
#4940=ORIENTED_EDGE ( 'NONE', *, *, #10326, .T. ) ;
#4946=CARTESIAN_POINT ( 'NONE',  ( 23.77500000054622475, 22.36655054427230027, 98.07665518445361386 ) ) ;
#4947=CARTESIAN_POINT ( 'NONE',  ( 24.15000000109246159, 12.11403331821300533, 90.79316153445363113 ) ) ;
#4948=CARTESIAN_POINT ( 'NONE',  ( 35.57500000054622546, 24.28113015263587116, 96.68563167572563088 ) ) ;
#4950=CARTESIAN_POINT ( 'NONE',  ( 20.39999999999998792, 12.86707612778636012, 93.11078899226572503 ) ) ;
#4951=EDGE_CURVE ( 'NONE', #11209, #7418, #5114, .T. ) ;
#4953=CARTESIAN_POINT ( 'NONE',  ( 29.97500000054622760, 15.71886984736413417, 96.68563167572563088 ) ) ;
#4955=DIRECTION ( 'NONE',  ( -0.000000000000000000, 0.000000000000000000, 1.000000000000000000 ) ) ;
#4957=VECTOR ( 'NONE', #2071, 1000.000000000000000 ) ;
#4958=CARTESIAN_POINT ( 'NONE',  ( 4.999999999999999112, 18.00000000000000355, 218.7511230907454944 ) ) ;
#4960=( BOUNDED_CURVE ( )  B_SPLINE_CURVE ( 2, ( #7754, #3187, #4965, #211, #3119, #3944, #1166, #81, #11881, #10788, #7820 ),
 .UNSPECIFIED., .F., .F. ) 
 B_SPLINE_CURVE_WITH_KNOTS ( ( 3, 2, 2, 2, 2, 3 ),
 ( 0.2999999999999999889, 0.3066666666666666430, 0.3133333333333333526, 0.3200000000000000622, 0.3266666666666667163, 0.3333333333333333703 ),
 .UNSPECIFIED. ) 
 CURVE ( )  GEOMETRIC_REPRESENTATION_ITEM ( )  RATIONAL_B_SPLINE_CURVE ( ( 1.000000000000000000, 0.9510565162951535312, 1.000000000000000000, 0.9510565162951535312, 1.000000000000000000, 0.9510565162951535312, 1.000000000000000000, 0.9510565162951535312, 1.000000000000000000, 0.9510565162951530871, 1.000000000000000444 ) ) 
 REPRESENTATION_ITEM ( '' )  );
#4961=PLANE ( 'NONE',  #2540 ) ;
#4963=ADVANCED_FACE ( 'NONE', ( #7574 ), #11503, .F. ) ;
#4964=CARTESIAN_POINT ( 'NONE',  ( 36.27500000054622120, 13.07298590277314254, 93.04388485072563242 ) ) ;
#4965=CARTESIAN_POINT ( 'NONE',  ( 40.45000000109246940, 15.59161060780646046, 84.72553407664153724 ) ) ;
#4967=CARTESIAN_POINT ( 'NONE',  ( 37.17500000054620557, 26.19570976099943493, 86.29171490190961435 ) ) ;
#4968=CARTESIAN_POINT ( 'NONE',  ( 42.99999999999999289, 20.00000000000000355, 83.29316153445364534 ) ) ;
#4970=EDGE_CURVE ( 'NONE', #7888, #5428, #6726, .T. ) ;
#4971=CARTESIAN_POINT ( 'NONE',  ( 39.09999999999999432, 22.43689772174678509, 83.29316153445363113 ) ) ;
#4974=CARTESIAN_POINT ( 'NONE',  ( 30.45000000109246585, 15.59161060780646046, 84.72553407664153724 ) ) ;
#4979=PLANE ( 'NONE',  #5471 ) ;
#4983=CARTESIAN_POINT ( 'NONE',  ( 32.37500000054622973, 13.07298590277314432, 88.54243821818161564 ) ) ;
#4984=CARTESIAN_POINT ( 'NONE',  ( 30.07500000054622546, 15.71886984736413417, 96.68563167572563088 ) ) ;
#4989=CARTESIAN_POINT ( 'NONE',  ( 48.67500000054622689, 15.71886984736413773, 84.90069139318163138 ) ) ;
#4993=CARTESIAN_POINT ( 'NONE',  ( -34.99999999999999289, 24.39339828220178674, 137.5000000000000000 ) ) ;
#4994=EDGE_CURVE ( 'NONE', #1035, #9150, #9859, .T. ) ;
#4997=ORIENTED_EDGE ( 'NONE', *, *, #1944, .T. ) ;
#5000=CARTESIAN_POINT ( 'NONE',  ( -21.00000000000001066, 77.00000000000000000, 154.3533255156881978 ) ) ;
#5003=CARTESIAN_POINT ( 'NONE',  ( -2.000000000000015543, 20.00000000000000355, 83.29316153445364534 ) ) ;
#5005=CARTESIAN_POINT ( 'NONE',  ( 40.97500000054622404, 24.28113015263587471, 84.90069139318163138 ) ) ;
#5011=CARTESIAN_POINT ( 'NONE',  ( 23.87500000054622262, 20.00000000000000355, 98.07665518445361386 ) ) ;
#5012=CARTESIAN_POINT ( 'NONE',  ( -6.999999999999999112, 77.00000000000000000, 101.8533255156881978 ) ) ;
#5013=CARTESIAN_POINT ( 'NONE',  ( 32.47500000054623115, 13.80429023900056684, 86.29171490190961435 ) ) ;
#5014=CARTESIAN_POINT ( 'NONE',  ( 22.57500000054622546, 13.80429023900056684, 86.29171490190961435 ) ) ;
#5015=CARTESIAN_POINT ( 'NONE',  ( 21.09999999999998010, 22.43689772174679575, 83.29316153445363113 ) ) ;
#5017=CARTESIAN_POINT ( 'NONE',  ( 33.17500000054622689, 26.92701409722686634, 88.54243821818162985 ) ) ;
#5018=EDGE_LOOP ( 'NONE', ( #7627, #9468, #10483, #3518, #2467, #4211 ) ) ;
#5024=CARTESIAN_POINT ( 'NONE',  ( 48.75000000109245946, 22.43689772174678509, 83.29316153445363113 ) ) ;
#5025=ORIENTED_EDGE ( 'NONE', *, *, #9864, .F. ) ;
#5027=CARTESIAN_POINT ( 'NONE',  ( 20.65000000109246514, 20.00000000000000355, 83.29316153445364534 ) ) ;
#5029=AXIS2_PLACEMENT_3D ( 'NONE', #7966, #11834, #6752 ) ;
#5030=CARTESIAN_POINT ( 'NONE',  ( 40.97500000054621694, 22.36655054427230382, 83.50966788445364841 ) ) ;
#5031=LINE ( 'NONE', #8960, #63 ) ;
#5032=CARTESIAN_POINT ( 'NONE',  ( 40.07500000054623257, 15.71886984736413417, 96.68563167572563088 ) ) ;
#5033=CARTESIAN_POINT ( 'NONE',  ( 40.69999999999999574, 13.62011893735971135, 86.15790661882942914 ) ) ;
#5034=CARTESIAN_POINT ( 'NONE',  ( 45.89999999999999147, 22.43689772174683128, 98.29316153445361692 ) ) ;
#5035=FACE_OUTER_BOUND ( 'NONE', #6789, .T. ) ;
#5037=CARTESIAN_POINT ( 'NONE',  ( 28.35000000109246443, 13.62011893735971135, 86.15790661882942914 ) ) ;
#5038=PLANE ( 'NONE',  #10955 ) ;
#5039=ORIENTED_EDGE ( 'NONE', *, *, #1653, .F. ) ;
#5040=( BOUNDED_CURVE ( )  B_SPLINE_CURVE ( 2, ( #6091, #2282, #5901, #5141, #9009, #8746, #1080, #8810, #129, #3988, #7865 ),
 .UNSPECIFIED., .F., .F. ) 
 B_SPLINE_CURVE_WITH_KNOTS ( ( 3, 2, 2, 2, 2, 3 ),
 ( 0.1000000000000000888, 0.1066666666666667568, 0.1133333333333334247, 0.1200000000000000927, 0.1266666666666667884, 0.1333333333333334425 ),
 .UNSPECIFIED. ) 
 CURVE ( )  GEOMETRIC_REPRESENTATION_ITEM ( )  RATIONAL_B_SPLINE_CURVE ( ( 0.9999999999999994449, 0.9510565162951540863, 1.000000000000000000, 0.9510565162951535312, 1.000000000000000000, 0.9510565162951535312, 1.000000000000000000, 0.9510565162951535312, 1.000000000000000000, 0.9510565162951527540, 1.000000000000000888 ) ) 
 REPRESENTATION_ITEM ( '' )  );
#5044=LINE ( 'NONE', #6120, #8704 ) ;
#5049=CARTESIAN_POINT ( 'NONE',  ( 30.67500000054622689, 17.63344945572770328, 83.50966788445364841 ) ) ;
#5050=CARTESIAN_POINT ( 'NONE',  ( 29.67500000054622333, 24.28113015263587116, 96.68563167572563088 ) ) ;
#5053=CARTESIAN_POINT ( 'NONE',  ( 33.65000000109246514, 20.00000000000000355, 98.29316153445363113 ) ) ;
#5055=CARTESIAN_POINT ( 'NONE',  ( 49.35000000109246798, 26.37988106264029398, 95.42841645007781892 ) ) ;
#5060=AXIS2_PLACEMENT_3D ( 'NONE', #3423, #4310, #632 ) ;
#5061=CARTESIAN_POINT ( 'NONE',  ( -33.79382810696421302, 14.62220435867159374, 151.2938281069642130 ) ) ;
#5067=CARTESIAN_POINT ( 'NONE',  ( 8.962237153663121347, 24.44132309231766698, 84.74490591176112275 ) ) ;
#5072=CARTESIAN_POINT ( 'NONE',  ( 45.07500000054621836, 26.19570976099943493, 86.29171490190961435 ) ) ;
#5074=VERTEX_POINT ( 'NONE', #3000 ) ;
#5078=CARTESIAN_POINT ( 'NONE',  ( 22.87500000054622618, 20.00000000000000355, 83.50966788445364841 ) ) ;
#5079=CARTESIAN_POINT ( 'NONE',  ( 48.47500000054622404, 13.07298590277314432, 88.54243821818161564 ) ) ;
#5080=CARTESIAN_POINT ( 'NONE',  ( 31.07500000054622546, 26.19570976099943849, 86.29171490190961435 ) ) ;
#5081=CARTESIAN_POINT ( 'NONE',  ( 23.97500000054622049, 17.63344945572769973, 98.07665518445361386 ) ) ;
#5082=CARTESIAN_POINT ( 'NONE',  ( 20.99999999999998579, 20.00000000000000355, 83.29316153445364534 ) ) ;
#5083=LINE ( 'NONE', #1275, #5458 ) ;
#5084=CARTESIAN_POINT ( 'NONE',  ( 28.67500000054623044, 17.63344945572770328, 83.50966788445364841 ) ) ;
#5085=EDGE_LOOP ( 'NONE', ( #1191, #11076, #3447, #586, #4702 ) ) ;
#5087=CARTESIAN_POINT ( 'NONE',  ( 33.55000000109246372, 22.43689772174679575, 98.29316153445363113 ) ) ;
#5093=CARTESIAN_POINT ( 'NONE',  ( 35.37500000054622973, 27.65831843345427998, 90.79316153445363113 ) ) ;
#5094=DIRECTION ( 'NONE',  ( -1.000000000000000000, 0.000000000000000000, 0.000000000000000000 ) ) ;
#5096=CARTESIAN_POINT ( 'NONE',  ( 20.55000000109246372, 17.56310227825320425, 83.29316153445363113 ) ) ;
#5097=CARTESIAN_POINT ( 'NONE',  ( 39.17500000054621978, 26.19570976099943493, 86.29171490190961435 ) ) ;
#5098=CARTESIAN_POINT ( 'NONE',  ( 44.39999999999999147, 12.86707612778636012, 93.11078899226572503 ) ) ;
#5099=CARTESIAN_POINT ( 'NONE',  ( 46.87500000054622262, 22.36655054427230382, 83.50966788445364841 ) ) ;
#5101=CARTESIAN_POINT ( 'NONE',  ( 28.75000000109245946, 22.43689772174679575, 83.29316153445363113 ) ) ;
#5103=ORIENTED_EDGE ( 'NONE', *, *, #11448, .F. ) ;
#5104=EDGE_CURVE ( 'NONE', #5277, #3559, #1978, .T. ) ;
#5105=FACE_OUTER_BOUND ( 'NONE', #5682, .T. ) ;
#5106=ORIENTED_EDGE ( 'NONE', *, *, #4009, .T. ) ;
#5109=DIRECTION ( 'NONE',  ( 1.000000000000000000, -0.000000000000000000, -0.000000000000000000 ) ) ;
#5111=EDGE_CURVE ( 'NONE', #10641, #2251, #8041, .T. ) ;
#5112=CARTESIAN_POINT ( 'NONE',  ( 29.57500000054622546, 24.28113015263587116, 96.68563167572563088 ) ) ;
#5113=CARTESIAN_POINT ( 'NONE',  ( 32.17500000054621978, 13.80429023900056507, 95.29460816699764791 ) ) ;
#5114=( BOUNDED_CURVE ( )  B_SPLINE_CURVE ( 2, ( #10420, #4528, #784, #5493, #7384, #9548, #2811, #8523, #3694, #3758, #7638 ),
 .UNSPECIFIED., .F., .F. ) 
 B_SPLINE_CURVE_WITH_KNOTS ( ( 3, 2, 2, 2, 2, 3 ),
 ( 0.3333333333333333703, 0.3400000000000000799, 0.3466666666666667340, 0.3533333333333333881, 0.3600000000000000422, 0.3666666666666666963 ),
 .UNSPECIFIED. ) 
 CURVE ( )  GEOMETRIC_REPRESENTATION_ITEM ( )  RATIONAL_B_SPLINE_CURVE ( ( 0.9999999999999995559, 0.9510565162951539753, 1.000000000000000000, 0.9510565162951535312, 1.000000000000000000, 0.9510565162951535312, 1.000000000000000000, 0.9510565162951535312, 1.000000000000000000, 0.9510565162951530871, 1.000000000000000444 ) ) 
 REPRESENTATION_ITEM ( '' )  );
#5117=ADVANCED_FACE ( 'NONE', ( #5035 ), #10217, .F. ) ;
#5118=CARTESIAN_POINT ( 'NONE',  ( 47.87500000054622262, 20.00000000000000355, 98.07665518445361386 ) ) ;
#5119=CARTESIAN_POINT ( 'NONE',  ( 48.15000000109246514, 12.11403331821300533, 90.79316153445363113 ) ) ;
#5120=DIRECTION ( 'NONE',  ( -1.000000000000000000, 0.000000000000000000, 0.000000000000000000 ) ) ;
#5122=DIRECTION ( 'NONE',  ( 0.000000000000000000, -0.000000000000000000, 1.000000000000000000 ) ) ;
#5123=ORIENTED_EDGE ( 'NONE', *, *, #720, .T. ) ;
#5128=CARTESIAN_POINT ( 'NONE',  ( 34.72841614740047333, 22.00000000000000000, 152.2284161474004520 ) ) ;
#5129=CARTESIAN_POINT ( 'NONE',  ( 9.682803526473488631, 22.51080964628191339, 83.72143117422299952 ) ) ;
#5130=CARTESIAN_POINT ( 'NONE',  ( 49.99999999999998579, 0.000000000000000000, 169.9999999999999716 ) ) ;
#5133=DIRECTION ( 'NONE',  ( -0.000000000000000000, -1.000000000000000000, -0.000000000000000000 ) ) ;
#5134=CARTESIAN_POINT ( 'NONE',  ( 42.77500000054622831, 20.00000000000000355, 83.50966788445364841 ) ) ;
#5137=ORIENTED_EDGE ( 'NONE', *, *, #8445, .T. ) ;
#5141=CARTESIAN_POINT ( 'NONE',  ( 46.69999999999998153, 13.62011893735970958, 86.15790661882942914 ) ) ;
#5142=CARTESIAN_POINT ( 'NONE',  ( 46.87500000054622262, 20.00000000000000355, 83.50966788445364841 ) ) ;
#5144=CARTESIAN_POINT ( 'NONE',  ( 33.07500000054623257, 26.19570976099943849, 86.29171490190961435 ) ) ;
#5146=CARTESIAN_POINT ( 'NONE',  ( 22.47500000054622404, 13.07298590277314432, 88.54243821818161564 ) ) ;
#5147=CARTESIAN_POINT ( 'NONE',  ( 49.99999999999998579, 0.000000000000000000, 82.99999999999995737 ) ) ;
#5148=CYLINDRICAL_SURFACE ( 'NONE', #3431, 7.499999999999992895 ) ;
#5149=CARTESIAN_POINT ( 'NONE',  ( 28.97500000054622760, 24.28113015263587471, 84.90069139318163138 ) ) ;
#5150=VERTEX_POINT ( 'NONE', #6462 ) ;
#5151=CARTESIAN_POINT ( 'NONE',  ( 22.95000000109246230, 26.37988106264029398, 86.15790661882942914 ) ) ;
#5153=VERTEX_POINT ( 'NONE', #8368 ) ;
#5154=CARTESIAN_POINT ( 'NONE',  ( -6.999999999999999112, 69.50000000000000000, 146.8533255156881978 ) ) ;
#5155=ORIENTED_EDGE ( 'NONE', *, *, #4592, .T. ) ;
#5159=CARTESIAN_POINT ( 'NONE',  ( 37.97500000054621694, 17.63344945572769973, 98.07665518445361386 ) ) ;
#5162=CARTESIAN_POINT ( 'NONE',  ( 40.57500000054621836, 13.80429023900056684, 86.29171490190961435 ) ) ;
#5163=CARTESIAN_POINT ( 'NONE',  ( 43.69999999999998863, 26.37988106264029398, 95.42841645007781892 ) ) ;
#5164=CARTESIAN_POINT ( 'NONE',  ( 44.37500000054622973, 13.07298590277314432, 88.54243821818161564 ) ) ;
#5165=ORIENTED_EDGE ( 'NONE', *, *, #6521, .T. ) ;
#5167=CARTESIAN_POINT ( 'NONE',  ( 24.85000000109246443, 24.40838939219355197, 84.72553407664153724 ) ) ;
#5169=ORIENTED_EDGE ( 'NONE', *, *, #647, .T. ) ;
#5172=FACE_OUTER_BOUND ( 'NONE', #8817, .T. ) ;
#5173=CARTESIAN_POINT ( 'NONE',  ( 41.25000000109246656, 27.13292387221364876, 93.11078899226573924 ) ) ;
#5174=CARTESIAN_POINT ( 'NONE',  ( 48.59999999999998721, 12.86707612778636012, 88.47553407664152303 ) ) ;
#5176=CARTESIAN_POINT ( 'NONE',  ( 31.17500000054622689, 26.92701409722686634, 88.54243821818162985 ) ) ;
#5177=CARTESIAN_POINT ( 'NONE',  ( 34.37500000054622973, 12.34168156654572535, 90.79316153445363113 ) ) ;
#5178=DIRECTION ( 'NONE',  ( 0.000000000000000000, 1.000000000000000000, -0.000000000000000000 ) ) ;
#5180=CARTESIAN_POINT ( 'NONE',  ( 22.05000000109246372, 12.86707612778636012, 93.11078899226572503 ) ) ;
#5182=CARTESIAN_POINT ( 'NONE',  ( 43.95000000109245519, 13.62011893735971135, 95.42841645007781892 ) ) ;
#5185=CARTESIAN_POINT ( 'NONE',  ( -28.50000000000001066, 84.49999999999998579, 146.8533255156881978 ) ) ;
#5188=EDGE_CURVE ( 'NONE', #4064, #10, #10206, .T. ) ;
#5194=CARTESIAN_POINT ( 'NONE',  ( 22.69999999999998153, 13.62011893735970958, 86.15790661882942914 ) ) ;
#5199=ORIENTED_EDGE ( 'NONE', *, *, #418, .T. ) ;
#5202=EDGE_CURVE ( 'NONE', #3966, #10690, #9956, .T. ) ;
#5203=PLANE ( 'NONE',  #744 ) ;
#5204=CARTESIAN_POINT ( 'NONE',  ( 47.17500000054622689, 26.19570976099943493, 86.29171490190961435 ) ) ;
#5206=CARTESIAN_POINT ( 'NONE',  ( 33.47500000054622404, 26.19570976099943849, 95.29460816699764791 ) ) ;
#5207=CARTESIAN_POINT ( 'NONE',  ( 7.417742579741789299, 13.28838962888333342, 94.17527653944314636 ) ) ;
#5208=CARTESIAN_POINT ( 'NONE',  ( 45.25000000109246656, 27.13292387221364876, 93.11078899226573924 ) ) ;
#5209=CARTESIAN_POINT ( 'NONE',  ( 24.77500000054622831, 20.00000000000000355, 83.50966788445364841 ) ) ;
#5211=CYLINDRICAL_SURFACE ( 'NONE', #11560, 7.499999999999992895 ) ;
#5212=VERTEX_POINT ( 'NONE', #3600 ) ;
#5218=EDGE_CURVE ( 'NONE', #9799, #652, #5520, .T. ) ;
#5219=CARTESIAN_POINT ( 'NONE',  ( 38.27500000054622831, 13.07298590277314254, 93.04388485072563242 ) ) ;
#5220=CARTESIAN_POINT ( 'NONE',  ( 36.79999999999998295, 15.59161060780646046, 84.72553407664153724 ) ) ;
#5221=DIRECTION ( 'NONE',  ( 0.000000000000000000, 0.000000000000000000, -1.000000000000000000 ) ) ;
#5222=CARTESIAN_POINT ( 'NONE',  ( 40.27500000054622120, 13.07298590277314254, 93.04388485072563242 ) ) ;
#5223=CARTESIAN_POINT ( 'NONE',  ( 37.69999999999998153, 26.37988106264029398, 95.42841645007781892 ) ) ;
#5224=EDGE_CURVE ( 'NONE', #5153, #6070, #6705, .T. ) ;
#5225=CARTESIAN_POINT ( 'NONE',  ( 43.77500000054622831, 20.00000000000000355, 98.07665518445361386 ) ) ;
#5227=CARTESIAN_POINT ( 'NONE',  ( 27.05000000109246372, 27.13292387221364876, 88.47553407664153724 ) ) ;
#5229=VERTEX_POINT ( 'NONE', #6519 ) ;
#5232=EDGE_CURVE ( 'NONE', #2033, #8953, #6259, .T. ) ;
#5235=LINE ( 'NONE', #9106, #8183 ) ;
#5236=CARTESIAN_POINT ( 'NONE',  ( 30.07500000054622546, 13.80429023900056507, 95.29460816699764791 ) ) ;
#5237=CARTESIAN_POINT ( 'NONE',  ( 22.57500000054622546, 13.80429023900056684, 86.29171490190961435 ) ) ;
#5239=DIRECTION ( 'NONE',  ( 0.000000000000000000, 0.000000000000000000, -1.000000000000000000 ) ) ;
#5241=VERTEX_POINT ( 'NONE', #12422 ) ;
#5242=CARTESIAN_POINT ( 'NONE',  ( 45.25000000109246656, 27.13292387221364876, 93.11078899226573924 ) ) ;
#5243=ORIENTED_EDGE ( 'NONE', *, *, #8754, .T. ) ;
#5249=VECTOR ( 'NONE', #6926, 1000.000000000000000 ) ;
#5250=CARTESIAN_POINT ( 'NONE',  ( 29.69999999999998508, 26.37988106264029398, 95.42841645007781892 ) ) ;
#5252=DIRECTION ( 'NONE',  ( 1.000000000000000000, 0.000000000000000000, 0.000000000000000000 ) ) ;
#5253=EDGE_CURVE ( 'NONE', #5929, #9442, #3009, .T. ) ;
#5254=CARTESIAN_POINT ( 'NONE',  ( 22.39999999999998437, 12.86707612778636012, 93.11078899226572503 ) ) ;
#5265=CARTESIAN_POINT ( 'NONE',  ( 42.87500000054622262, 20.00000000000000355, 83.50966788445364841 ) ) ;
#5266=CARTESIAN_POINT ( 'NONE',  ( 25.27500000054622475, 27.65831843345427998, 90.79316153445363113 ) ) ;
#5267=CARTESIAN_POINT ( 'NONE',  ( 9.684959410070431929, 17.49741726564071698, 83.71847969554855240 ) ) ;
#5268=CARTESIAN_POINT ( 'NONE',  ( 45.35000000109246088, 26.37988106264029398, 95.42841645007781892 ) ) ;
#5270=CARTESIAN_POINT ( 'NONE',  ( 31.59999999999999076, 27.13292387221364876, 93.11078899226573924 ) ) ;
#5271=CARTESIAN_POINT ( 'NONE',  ( 28.87500000054622262, 22.36655054427230382, 83.50966788445364841 ) ) ;
#5274=DIRECTION ( 'NONE',  ( 0.000000000000000000, 0.000000000000000000, -1.000000000000000000 ) ) ;
#5275=VERTEX_POINT ( 'NONE', #10386 ) ;
#5277=VERTEX_POINT ( 'NONE', #4684 ) ;
#5281=CARTESIAN_POINT ( 'NONE',  ( 33.27500000054622831, 26.92701409722686634, 88.54243821818162985 ) ) ;
#5282=CARTESIAN_POINT ( 'NONE',  ( 49.99999999999998579, 18.00000000000000355, 69.99999999999998579 ) ) ;
#5283=CARTESIAN_POINT ( 'NONE',  ( 48.77500000054622831, 20.00000000000000355, 83.50966788445364841 ) ) ;
#5284=CARTESIAN_POINT ( 'NONE',  ( 32.77500000054622831, 17.63344945572770328, 83.50966788445364841 ) ) ;
#5285=CARTESIAN_POINT ( 'NONE',  ( 36.99999999999999289, 20.00000000000000355, 83.29316153445364534 ) ) ;
#5287=CARTESIAN_POINT ( 'NONE',  ( 45.57500000054622546, 24.28113015263587116, 96.68563167572563088 ) ) ;
#5289=CARTESIAN_POINT ( 'NONE',  ( 21.75000000109246656, 17.56310227825320425, 98.29316153445363113 ) ) ;
#5295=CARTESIAN_POINT ( 'NONE',  ( 20.75000000109246301, 22.43689772174679575, 83.29316153445363113 ) ) ;
#5298=CARTESIAN_POINT ( 'NONE',  ( -2.000000000000015543, 20.00000000000000355, 98.29316153445363113 ) ) ;
#5300=CARTESIAN_POINT ( 'NONE',  ( 24.07500000054622902, 13.80429023900056507, 95.29460816699764791 ) ) ;
#5301=CARTESIAN_POINT ( 'NONE',  ( 23.67500000054622333, 24.28113015263587116, 96.68563167572563088 ) ) ;
#5304=LINE ( 'NONE', #10241, #9088 ) ;
#5306=VECTOR ( 'NONE', #11225, 1000.000000000000000 ) ;
#5307=CARTESIAN_POINT ( 'NONE',  ( 43.15000000109247225, 27.88596668178699645, 90.79316153445363113 ) ) ;
#5309=ORIENTED_EDGE ( 'NONE', *, *, #8252, .F. ) ;
#5315=CARTESIAN_POINT ( 'NONE',  ( 20.97500000054622760, 24.28113015263587471, 84.90069139318163138 ) ) ;
#5320=CARTESIAN_POINT ( 'NONE',  ( -6.999999999999999112, 40.00000000000000000, 69.99999999999998579 ) ) ;
#5323=ORIENTED_EDGE ( 'NONE', *, *, #2474, .T. ) ;
#5327=CARTESIAN_POINT ( 'NONE',  ( 28.19999999999998863, 15.59161060780645691, 96.86078899226572503 ) ) ;
#5328=CARTESIAN_POINT ( 'NONE',  ( 47.07500000054622546, 24.28113015263587471, 84.90069139318163138 ) ) ;
#5329=CARTESIAN_POINT ( 'NONE',  ( 23.97500000054623115, 15.71886984736413417, 96.68563167572563088 ) ) ;
#5331=CARTESIAN_POINT ( 'NONE',  ( 45.05000000109246372, 27.13292387221364876, 88.47553407664153724 ) ) ;
#5333=CARTESIAN_POINT ( 'NONE',  ( 39.99999999999998579, 20.00000000000000355, 98.29316153445363113 ) ) ;
#5334=CYLINDRICAL_SURFACE ( 'NONE', #2822, 7.499999999999978684 ) ;
#5336=CARTESIAN_POINT ( 'NONE',  ( -2.000000000000015543, 20.00000000000000355, 90.79316153445363113 ) ) ;
#5338=CARTESIAN_POINT ( 'NONE',  ( -2.000000000000015543, 20.00000000000000355, 90.79316153445363113 ) ) ;
#5339=ORIENTED_EDGE ( 'NONE', *, *, #7376, .T. ) ;
#5341=AXIS2_PLACEMENT_3D ( 'NONE', #9574, #755, #1949 ) ;
#5342=CARTESIAN_POINT ( 'NONE',  ( 33.37500000054621552, 27.65831843345427998, 90.79316153445363113 ) ) ;
#5344=CARTESIAN_POINT ( 'NONE',  ( 49.07500000054622546, 26.19570976099943849, 86.29171490190961435 ) ) ;
#5345=CARTESIAN_POINT ( 'NONE',  ( 36.87500000054622262, 20.00000000000000355, 83.50966788445364841 ) ) ;
#5346=CARTESIAN_POINT ( 'NONE',  ( 38.09999999999999432, 17.56310227825320425, 98.29316153445363113 ) ) ;
#5347=CARTESIAN_POINT ( 'NONE',  ( 44.67500000054623399, 17.63344945572770328, 83.50966788445364841 ) ) ;
#5350=CARTESIAN_POINT ( 'NONE',  ( 27.15000000109245804, 27.88596668178699645, 90.79316153445363113 ) ) ;
#5354=LINE ( 'NONE', #11471, #7688 ) ;
#5357=CARTESIAN_POINT ( 'NONE',  ( 20.65000000109246514, 20.00000000000000355, 83.29316153445364534 ) ) ;
#5358=CARTESIAN_POINT ( 'NONE',  ( 35.75000000109246656, 17.56310227825319004, 98.29316153445361692 ) ) ;
#5359=CARTESIAN_POINT ( 'NONE',  ( 25.39999999999998792, 27.13292387221364876, 88.47553407664153724 ) ) ;
#5362=CARTESIAN_POINT ( 'NONE',  ( 26.17500000054623044, 13.07298590277314254, 93.04388485072563242 ) ) ;
#5363=CARTESIAN_POINT ( 'NONE',  ( 27.47500000054622404, 26.92701409722686634, 93.04388485072563242 ) ) ;
#5366=CARTESIAN_POINT ( 'NONE',  ( 22.65000000109246514, 20.00000000000000355, 83.29316153445364534 ) ) ;
#5367=ORIENTED_EDGE ( 'NONE', *, *, #12541, .T. ) ;
#5369=CARTESIAN_POINT ( 'NONE',  ( 45.65000000109247225, 20.00000000000000355, 98.29316153445363113 ) ) ;
#5379=DIRECTION ( 'NONE',  ( 0.000000000000000000, 0.000000000000000000, 1.000000000000000000 ) ) ;
#5386=CARTESIAN_POINT ( 'NONE',  ( 47.15000000109245804, 27.88596668178699645, 90.79316153445363113 ) ) ;
#5387=ORIENTED_EDGE ( 'NONE', *, *, #6227, .F. ) ;
#5388=PLANE ( 'NONE',  #3980 ) ;
#5389=VECTOR ( 'NONE', #5756, 1000.000000000000000 ) ;
#5391=CARTESIAN_POINT ( 'NONE',  ( 0.000000000000000000, 20.00000000000000355, 109.9999999999999858 ) ) ;
#5392=CARTESIAN_POINT ( 'NONE',  ( 42.17500000054623399, 13.80429023900056507, 95.29460816699764791 ) ) ;
#5393=CARTESIAN_POINT ( 'NONE',  ( 27.27500000054622475, 27.65831843345427998, 90.79316153445363113 ) ) ;
#5394=CARTESIAN_POINT ( 'NONE',  ( 9.403487956461118458, 16.59018621808800020, 84.10865954674225975 ) ) ;
#5395=CARTESIAN_POINT ( 'NONE',  ( 44.95000000109246230, 26.37988106264029398, 86.15790661882942914 ) ) ;
#5396=DIRECTION ( 'NONE',  ( 1.000000000000000000, -0.000000000000000000, -0.000000000000000000 ) ) ;
#5397=DIRECTION ( 'NONE',  ( 0.000000000000000000, 0.000000000000000000, -1.000000000000000000 ) ) ;
#5399=CARTESIAN_POINT ( 'NONE',  ( -6.999999999999999112, 55.00000000000000000, 166.8533255156881694 ) ) ;
#5400=ORIENTED_EDGE ( 'NONE', *, *, #1713, .T. ) ;
#5401=DIRECTION ( 'NONE',  ( 0.000000000000000000, 0.000000000000000000, -1.000000000000000000 ) ) ;
#5404=CARTESIAN_POINT ( 'NONE',  ( 33.87500000054622262, 20.00000000000000355, 98.07665518445361386 ) ) ;
#5406=CARTESIAN_POINT ( 'NONE',  ( 47.87500000054622973, 17.63344945572769973, 98.07665518445361386 ) ) ;
#5407=CARTESIAN_POINT ( 'NONE',  ( 31.67500000054622333, 24.28113015263587116, 96.68563167572563088 ) ) ;
#5408=CARTESIAN_POINT ( 'NONE',  ( 33.39999999999998437, 27.13292387221364876, 88.47553407664153724 ) ) ;
#5411=CARTESIAN_POINT ( 'NONE',  ( 41.87500000054622262, 17.63344945572769973, 98.07665518445361386 ) ) ;
#5413=CARTESIAN_POINT ( 'NONE',  ( 25.15000000109246159, 27.88596668178699645, 90.79316153445363113 ) ) ;
#5416=VERTEX_POINT ( 'NONE', #7855 ) ;
#5418=ORIENTED_EDGE ( 'NONE', *, *, #2500, .T. ) ;
#5419=DIRECTION ( 'NONE',  ( 1.000000000000000000, -0.000000000000000000, -0.000000000000000000 ) ) ;
#5421=CARTESIAN_POINT ( 'NONE',  ( 36.25000000109246656, 12.86707612778636012, 88.47553407664152303 ) ) ;
#5422=CARTESIAN_POINT ( 'NONE',  ( 32.35000000109246088, 13.62011893735970958, 86.15790661882942914 ) ) ;
#5424=CARTESIAN_POINT ( 'NONE',  ( 26.27500000054622475, 12.34168156654572535, 90.79316153445363113 ) ) ;
#5425=CARTESIAN_POINT ( 'NONE',  ( 25.87500000054622618, 20.00000000000000355, 98.07665518445361386 ) ) ;
#5427=CARTESIAN_POINT ( 'NONE',  ( 0.000000000000000000, 18.00000000000000355, 169.9999999999999716 ) ) ;
#5428=VERTEX_POINT ( 'NONE', #2070 ) ;
#5429=CARTESIAN_POINT ( 'NONE',  ( 43.85000000109246798, 15.59161060780645691, 96.86078899226572503 ) ) ;
#5432=CARTESIAN_POINT ( 'NONE',  ( 29.75000000109246301, 17.56310227825320425, 98.29316153445363113 ) ) ;
#5433=EDGE_CURVE ( 'NONE', #5434, #10300, #6836, .T. ) ;
#5434=VERTEX_POINT ( 'NONE', #5130 ) ;
#5435=VECTOR ( 'NONE', #7316, 1000.000000000000000 ) ;
#5439=CARTESIAN_POINT ( 'NONE',  ( 28.99999999999998934, 20.00000000000000355, 83.29316153445364534 ) ) ;
#5441=AXIS2_PLACEMENT_3D ( 'NONE', #10545, #1855, #9362 ) ;
#5442=CARTESIAN_POINT ( 'NONE',  ( 38.25000000109246656, 12.86707612778636012, 88.47553407664152303 ) ) ;
#5444=CARTESIAN_POINT ( 'NONE',  ( 42.79999999999999005, 15.59161060780646046, 84.72553407664153724 ) ) ;
#5449=( BOUNDED_CURVE ( )  B_SPLINE_CURVE ( 2, ( #6329, #10200, #1510, #8302, #3474, #7339, #3846, #8607, #3197, #10937, #2898 ),
 .UNSPECIFIED., .F., .F. ) 
 B_SPLINE_CURVE_WITH_KNOTS ( ( 3, 2, 2, 2, 2, 3 ),
 ( 0.8666666666666666963, 0.8733333333333332948, 0.8800000000000000044, 0.8866666666666667140, 0.8933333333333333126, 0.9000000000000000222 ),
 .UNSPECIFIED. ) 
 CURVE ( )  GEOMETRIC_REPRESENTATION_ITEM ( )  RATIONAL_B_SPLINE_CURVE ( ( 1.000000000000000000, 0.9510565162951535312, 1.000000000000000000, 0.9510565162951535312, 1.000000000000000000, 0.9510565162951535312, 1.000000000000000000, 0.9510565162951535312, 1.000000000000000000, 0.9510565162951535312, 1.000000000000000000 ) ) 
 REPRESENTATION_ITEM ( '' )  );
#5456=CARTESIAN_POINT ( 'NONE',  ( 39.37500000054622262, 27.65831843345427998, 90.79316153445363113 ) ) ;
#5457=CARTESIAN_POINT ( 'NONE',  ( 28.27500000054622475, 12.34168156654572357, 90.79316153445363113 ) ) ;
#5458=VECTOR ( 'NONE', #3993, 1000.000000000000000 ) ;
#5459=CARTESIAN_POINT ( 'NONE',  ( 6.687975528478859566, 12.56545023609454681, 91.81450773486812977 ) ) ;
#5462=CARTESIAN_POINT ( 'NONE',  ( 33.99999999999998579, 20.00000000000000355, 98.29316153445363113 ) ) ;
#5463=DIRECTION ( 'NONE',  ( 1.000000000000000000, -0.000000000000000000, -0.000000000000000000 ) ) ;
#5464=ADVANCED_FACE ( 'NONE', ( #10635 ), #5890, .F. ) ;
#5465=VERTEX_POINT ( 'NONE', #4172 ) ;
#5467=VERTEX_POINT ( 'NONE', #5827 ) ;
#5468=DIRECTION ( 'NONE',  ( -1.000000000000000000, -0.000000000000000000, -0.000000000000000000 ) ) ;
#5470=VECTOR ( 'NONE', #7607, 1000.000000000000000 ) ;
#5471=AXIS2_PLACEMENT_3D ( 'NONE', #8907, #2253, #3261 ) ;
#5472=CARTESIAN_POINT ( 'NONE',  ( 34.97500000054622404, 22.36655054427230382, 83.50966788445364841 ) ) ;
#5473=DIRECTION ( 'NONE',  ( 0.000000000000000000, 0.000000000000000000, 1.000000000000000000 ) ) ;
#5474=CARTESIAN_POINT ( 'NONE',  ( 46.87500000054622262, 22.36655054427230382, 83.50966788445364841 ) ) ;
#5475=CARTESIAN_POINT ( 'NONE',  ( 35.17500000054621268, 26.19570976099943493, 86.29171490190961435 ) ) ;
#5476=CARTESIAN_POINT ( 'NONE',  ( 36.09999999999999432, 17.56310227825320425, 98.29316153445363113 ) ) ;
#5478=CARTESIAN_POINT ( 'NONE',  ( 37.67500000054623399, 22.36655054427230027, 98.07665518445361386 ) ) ;
#5480=CARTESIAN_POINT ( 'NONE',  ( 47.67500000054622689, 22.36655054427230027, 98.07665518445361386 ) ) ;
#5481=LINE ( 'NONE', #6597, #9943 ) ;
#5484=ORIENTED_EDGE ( 'NONE', *, *, #4134, .F. ) ;
#5487=EDGE_CURVE ( 'NONE', #513, #574, #7141, .T. ) ;
#5490=CARTESIAN_POINT ( 'NONE',  ( 25.97500000054622760, 15.71886984736413417, 96.68563167572563088 ) ) ;
#5491=CARTESIAN_POINT ( 'NONE',  ( 23.97500000054622049, 17.63344945572769973, 98.07665518445361386 ) ) ;
#5493=CARTESIAN_POINT ( 'NONE',  ( 39.35000000109246088, 26.37988106264029398, 95.42841645007781892 ) ) ;
#5495=CARTESIAN_POINT ( 'NONE',  ( 40.75000000109245946, 22.43689772174679575, 83.29316153445363113 ) ) ;
#5498=LINE ( 'NONE', #1495, #9311 ) ;
#5503=EDGE_CURVE ( 'NONE', #2004, #589, #181, .T. ) ;
#5504=DIRECTION ( 'NONE',  ( 0.000000000000000000, 0.000000000000000000, -1.000000000000000000 ) ) ;
#5505=EDGE_CURVE ( 'NONE', #11823, #6070, #6014, .T. ) ;
#5508=CARTESIAN_POINT ( 'NONE',  ( 42.89999999999998437, 17.56310227825321491, 83.29316153445364534 ) ) ;
#5510=CARTESIAN_POINT ( 'NONE',  ( 29.67500000054623044, 22.36655054427230027, 98.07665518445361386 ) ) ;
#5511=CARTESIAN_POINT ( 'NONE',  ( -50.00000000000001421, 20.00000000000000000, 137.5000000000000000 ) ) ;
#5516=CARTESIAN_POINT ( 'NONE',  ( 37.27500000054622831, 27.65831843345427998, 90.79316153445363113 ) ) ;
#5517=CARTESIAN_POINT ( 'NONE',  ( 40.07500000054623257, 15.71886984736413417, 96.68563167572563088 ) ) ;
#5518=ADVANCED_FACE ( 'NONE', ( #7334 ), #6325, .F. ) ;
#5519=CARTESIAN_POINT ( 'NONE',  ( 27.47500000054622049, 26.19570976099943849, 95.29460816699764791 ) ) ;
#5520=LINE ( 'NONE', #8555, #8890 ) ;
#5521=DIRECTION ( 'NONE',  ( 0.000000000000000000, 0.000000000000000000, -1.000000000000000000 ) ) ;
#5522=CARTESIAN_POINT ( 'NONE',  ( 33.89999999999998437, 22.43689772174679575, 98.29316153445363113 ) ) ;
#5524=( BOUNDED_CURVE ( )  B_SPLINE_CURVE ( 3, ( #5810, #11770, #1060, #6941 ),
 .UNSPECIFIED., .F., .F. ) 
 B_SPLINE_CURVE_WITH_KNOTS ( ( 4, 4 ),
 ( 4.712388980384689674, 6.013252511346182771 ),
 .UNSPECIFIED. ) 
 CURVE ( )  GEOMETRIC_REPRESENTATION_ITEM ( )  RATIONAL_B_SPLINE_CURVE ( ( 1.000000000000000000, 0.8638816171694809753, 0.8638816171694809753, 1.000000000000000000 ) ) 
 REPRESENTATION_ITEM ( '' )  );
#5525=VERTEX_POINT ( 'NONE', #12164 ) ;
#5529=CARTESIAN_POINT ( 'NONE',  ( 27.50000000000000355, 12.50000000000001066, 145.0000000000000000 ) ) ;
#5532=CARTESIAN_POINT ( 'NONE',  ( 34.17500000054622689, 13.80429023900056507, 95.29460816699764791 ) ) ;
#5534=CARTESIAN_POINT ( 'NONE',  ( 45.07500000054621836, 26.19570976099943849, 86.29171490190961435 ) ) ;
#5535=CARTESIAN_POINT ( 'NONE',  ( 36.27500000054622120, 13.07298590277314254, 93.04388485072563242 ) ) ;
#5536=CARTESIAN_POINT ( 'NONE',  ( 32.79999999999999005, 15.59161060780646046, 84.72553407664153724 ) ) ;
#5538=CARTESIAN_POINT ( 'NONE',  ( 39.87500000054622262, 17.63344945572769973, 98.07665518445361386 ) ) ;
#5540=CARTESIAN_POINT ( 'NONE',  ( 49.27500000054623541, 27.65831843345427998, 90.79316153445363113 ) ) ;
#5541=DIRECTION ( 'NONE',  ( 0.000000000000000000, 1.000000000000000000, 0.000000000000000000 ) ) ;
#5544=VERTEX_POINT ( 'NONE', #7273 ) ;
#5545=AXIS2_PLACEMENT_3D ( 'NONE', #1463, #511, #4373 ) ;
#5549=CARTESIAN_POINT ( 'NONE',  ( -2.000000000000015543, 20.00000000000000355, 90.79316153445363113 ) ) ;
#5550=CARTESIAN_POINT ( 'NONE',  ( 25.87500000054622262, 17.63344945572769973, 98.07665518445361386 ) ) ;
#5551=CARTESIAN_POINT ( 'NONE',  ( 49.39999999999998437, 27.13292387221364876, 88.47553407664153724 ) ) ;
#5552=CARTESIAN_POINT ( 'NONE',  ( -28.50000000000001066, 77.00000000000000000, 166.8533255156881694 ) ) ;
#5553=LINE ( 'NONE', #10295, #4414 ) ;
#5555=CARTESIAN_POINT ( 'NONE',  ( 36.65000000109245804, 20.00000000000000355, 83.29316153445364534 ) ) ;
#5557=VERTEX_POINT ( 'NONE', #4296 ) ;
#5558=CYLINDRICAL_SURFACE ( 'NONE', #10041, 7.500000000000000000 ) ;
#5568=CARTESIAN_POINT ( 'NONE',  ( 20.57500000054622902, 15.71886984736413773, 84.90069139318163138 ) ) ;
#5575=CARTESIAN_POINT ( 'NONE',  ( -50.00000000000001421, 18.00000000000000355, 152.2284161474004520 ) ) ;
#5576=CARTESIAN_POINT ( 'NONE',  ( 37.17500000054620557, 26.19570976099943493, 86.29171490190961435 ) ) ;
#5578=CARTESIAN_POINT ( 'NONE',  ( 23.17500000054622689, 26.92701409722686634, 88.54243821818162985 ) ) ;
#5579=AXIS2_PLACEMENT_3D ( 'NONE', #1249, #7970, #5120 ) ;
#5585=ORIENTED_EDGE ( 'NONE', *, *, #729, .F. ) ;
#5590=CARTESIAN_POINT ( 'NONE',  ( 25.37500000054622618, 27.65831843345427998, 90.79316153445363113 ) ) ;
#5592=CARTESIAN_POINT ( 'NONE',  ( 42.77500000054622831, 20.00000000000000355, 83.50966788445364841 ) ) ;
#5593=CARTESIAN_POINT ( 'NONE',  ( 30.27500000054622475, 13.07298590277314254, 93.04388485072563242 ) ) ;
#5594=CARTESIAN_POINT ( 'NONE',  ( 31.79999999999998650, 24.40838939219354842, 96.86078899226572503 ) ) ;
#5596=CARTESIAN_POINT ( 'NONE',  ( 41.57500000054623257, 24.28113015263587116, 96.68563167572563088 ) ) ;
#5598=CARTESIAN_POINT ( 'NONE',  ( 48.27500000054622120, 12.34168156654572535, 90.79316153445363113 ) ) ;
#5604=CARTESIAN_POINT ( 'NONE',  ( 42.15000000109246514, 12.11403331821300533, 90.79316153445363113 ) ) ;
#5605=FACE_OUTER_BOUND ( 'NONE', #4160, .T. ) ;
#5606=CARTESIAN_POINT ( 'NONE',  ( 47.07500000054622546, 24.28113015263587471, 84.90069139318163138 ) ) ;
#5609=CARTESIAN_POINT ( 'NONE',  ( 43.67500000054621978, 24.28113015263587116, 96.68563167572563088 ) ) ;
#5610=CARTESIAN_POINT ( 'NONE',  ( 46.19999999999998863, 15.59161060780645691, 96.86078899226572503 ) ) ;
#5613=ORIENTED_EDGE ( 'NONE', *, *, #2508, .F. ) ;
#5614=CARTESIAN_POINT ( 'NONE',  ( 38.35000000109246798, 13.62011893735971135, 86.15790661882942914 ) ) ;
#5618=EDGE_LOOP ( 'NONE', ( #11934, #1049, #4639, #4047, #4517, #7195, #515, #4913, #9332, #9986, #4179, #10997, #11224, #9748, #4457, #4788, #2862, #8223, #1919, #5243, #4122, #301, #5323, #2356, #8550, #5199, #4851, #4312, #12445, #12001, #423, #201, #11164 ) ) ;
#5620=VECTOR ( 'NONE', #11403, 1000.000000000000000 ) ;
#5621=CARTESIAN_POINT ( 'NONE',  ( 30.95000000109246940, 26.37988106264029398, 86.15790661882942914 ) ) ;
#5624=DIRECTION ( 'NONE',  ( 0.000000000000000000, 0.000000000000000000, 1.000000000000000000 ) ) ;
#5625=DIRECTION ( 'NONE',  ( 0.000000000000000000, 0.000000000000000000, -1.000000000000000000 ) ) ;
#5627=CARTESIAN_POINT ( 'NONE',  ( 48.97500000054622404, 22.36655054427230382, 83.50966788445364841 ) ) ;
#5628=VECTOR ( 'NONE', #11218, 1000.000000000000000 ) ;
#5635=( BOUNDED_CURVE ( )  B_SPLINE_CURVE ( 2, ( #11944, #5096, #3307, #11052, #7883, #2360, #6109, #9979, #1288, #1100, #3249 ),
 .UNSPECIFIED., .F., .F. ) 
 B_SPLINE_CURVE_WITH_KNOTS ( ( 3, 2, 2, 2, 2, 3 ),
 ( 0.9666666666666666741, 0.9733333333333333837, 0.9799999999999999822, 0.9866666666666666918, 0.9933333333333332904, 1.000000000000000000 ),
 .UNSPECIFIED. ) 
 CURVE ( )  GEOMETRIC_REPRESENTATION_ITEM ( )  RATIONAL_B_SPLINE_CURVE ( ( 1.000000000000000000, 0.9510565162951535312, 1.000000000000000000, 0.9510565162951535312, 1.000000000000000000, 0.9510565162951535312, 1.000000000000000000, 0.9510565162951535312, 1.000000000000000000, 0.9510565162951535312, 1.000000000000000000 ) ) 
 REPRESENTATION_ITEM ( '' )  );
#5637=CARTESIAN_POINT ( 'NONE',  ( 34.87500000054622262, 20.00000000000000355, 83.50966788445364841 ) ) ;
#5638=CARTESIAN_POINT ( 'NONE',  ( 19.87500000054622618, 17.63344945572769973, 98.07665518445361386 ) ) ;
#5640=PLANE ( 'NONE',  #10226 ) ;
#5644=CARTESIAN_POINT ( 'NONE',  ( -2.000000000000015543, 20.00000000000000355, 90.79316153445363113 ) ) ;
#5650=CARTESIAN_POINT ( 'NONE',  ( 26.87500000054622618, 20.00000000000000355, 83.50966788445364841 ) ) ;
#5652=CARTESIAN_POINT ( 'NONE',  ( 42.67500000054622689, 17.63344945572770328, 83.50966788445364841 ) ) ;
#5653=CARTESIAN_POINT ( 'NONE',  ( 25.57500000054621836, 26.19570976099943493, 95.29460816699764791 ) ) ;
#5654=CARTESIAN_POINT ( 'NONE',  ( 28.09999999999999076, 17.56310227825320425, 98.29316153445363113 ) ) ;
#5657=CARTESIAN_POINT ( 'NONE',  ( 41.17500000054623399, 26.92701409722686634, 88.54243821818162985 ) ) ;
#5659=CARTESIAN_POINT ( 'NONE',  ( 46.67500000054623399, 17.63344945572770328, 83.50966788445364841 ) ) ;
#5662=VECTOR ( 'NONE', #10650, 1000.000000000000000 ) ;
#5668=CARTESIAN_POINT ( 'NONE',  ( 42.65000000109246514, 20.00000000000000355, 83.29316153445364534 ) ) ;
#5671=CARTESIAN_POINT ( 'NONE',  ( 44.57500000054622546, 13.80429023900056684, 86.29171490190961435 ) ) ;
#5672=DIRECTION ( 'NONE',  ( 1.000000000000000000, -0.000000000000000000, -0.000000000000000000 ) ) ;
#5674=CARTESIAN_POINT ( 'NONE',  ( 45.97500000054623115, 17.63344945572769973, 98.07665518445361386 ) ) ;
#5675=CARTESIAN_POINT ( 'NONE',  ( 47.09999999999999432, 22.43689772174679575, 83.29316153445363113 ) ) ;
#5676=EDGE_CURVE ( 'NONE', #6680, #9812, #10075, .T. ) ;
#5677=CARTESIAN_POINT ( 'NONE',  ( 41.09999999999998721, 22.43689772174679575, 83.29316153445363113 ) ) ;
#5680=CARTESIAN_POINT ( 'NONE',  ( 34.65000000109246514, 20.00000000000000355, 83.29316153445364534 ) ) ;
#5682=EDGE_LOOP ( 'NONE', ( #7404, #10172, #5991, #9860, #2960, #1874 ) ) ;
#5683=EDGE_CURVE ( 'NONE', #12416, #1942, #6403, .T. ) ;
#5689=EDGE_CURVE ( 'NONE', #10115, #707, #928, .T. ) ;
#5692=CARTESIAN_POINT ( 'NONE',  ( 21.99999999999998934, 20.00000000000000355, 98.29316153445363113 ) ) ;
#5693=EDGE_LOOP ( 'NONE', ( #10189, #7109, #8456, #154 ) ) ;
#5694=AXIS2_PLACEMENT_3D ( 'NONE', #5336, #2469, #392 ) ;
#5696=FACE_OUTER_BOUND ( 'NONE', #6366, .T. ) ;
#5697=CARTESIAN_POINT ( 'NONE',  ( 49.07500000054622546, 24.28113015263587471, 84.90069139318163138 ) ) ;
#5700=FACE_OUTER_BOUND ( 'NONE', #10852, .T. ) ;
#5703=CARTESIAN_POINT ( 'NONE',  ( 21.39999999999998792, 27.13292387221364876, 88.47553407664153724 ) ) ;
#5708=CARTESIAN_POINT ( 'NONE',  ( -21.00000000000001066, 77.00000000000000000, 154.3533255156881978 ) ) ;
#5709=CARTESIAN_POINT ( 'NONE',  ( 25.85000000109246443, 15.59161060780645691, 96.86078899226572503 ) ) ;
#5712=DIRECTION ( 'NONE',  ( -1.000000000000000000, 0.000000000000000000, 0.000000000000000000 ) ) ;
#5714=CARTESIAN_POINT ( 'NONE',  ( 27.07500000054622546, 24.28113015263587471, 84.90069139318163138 ) ) ;
#5715=CARTESIAN_POINT ( 'NONE',  ( 0.000000000000000000, 20.00000000000000355, 109.9999999999999858 ) ) ;
#5716=CARTESIAN_POINT ( 'NONE',  ( 40.47500000054621694, 13.80429023900056684, 86.29171490190961435 ) ) ;
#5717=CARTESIAN_POINT ( 'NONE',  ( 25.27500000054622475, 26.92701409722686634, 88.54243821818162985 ) ) ;
#5718=CARTESIAN_POINT ( 'NONE',  ( 29.59999999999998721, 27.13292387221364876, 93.11078899226573924 ) ) ;
#5720=CARTESIAN_POINT ( 'NONE',  ( 34.47500000054623115, 13.80429023900056684, 86.29171490190961435 ) ) ;
#5722=CARTESIAN_POINT ( 'NONE',  ( 46.17500000054623399, 13.07298590277314254, 93.04388485072563242 ) ) ;
#5728=VERTEX_POINT ( 'NONE', #8416 ) ;
#5730=LINE ( 'NONE', #11313, #6034 ) ;
#5731=CARTESIAN_POINT ( 'NONE',  ( 47.27500000054622831, 26.92701409722686634, 88.54243821818162985 ) ) ;
#5732=CARTESIAN_POINT ( 'NONE',  ( 20.19999999999998863, 15.59161060780645691, 96.86078899226572503 ) ) ;
#5734=CARTESIAN_POINT ( 'NONE',  ( 44.77500000054622831, 17.63344945572770328, 83.50966788445364841 ) ) ;
#5735=CARTESIAN_POINT ( 'NONE',  ( 48.99999999999998579, 20.00000000000000355, 83.29316153445364534 ) ) ;
#5736=DIRECTION ( 'NONE',  ( 0.000000000000000000, -0.000000000000000000, -1.000000000000000000 ) ) ;
#5738=VERTEX_POINT ( 'NONE', #8478 ) ;
#5740=CARTESIAN_POINT ( 'NONE',  ( 39.65000000109246514, 20.00000000000000355, 98.29316153445363113 ) ) ;
#5748=CARTESIAN_POINT ( 'NONE',  ( 36.47500000054622404, 13.80429023900056684, 86.29171490190961435 ) ) ;
#5749=CARTESIAN_POINT ( 'NONE',  ( 34.72841614740048044, 22.00000000000000000, 169.9999999999999716 ) ) ;
#5750=CARTESIAN_POINT ( 'NONE',  ( 27.19999999999998863, 24.40838939219355197, 84.72553407664153724 ) ) ;
#5754=CARTESIAN_POINT ( 'NONE',  ( 23.17500000054622689, 26.92701409722686634, 88.54243821818162985 ) ) ;
#5756=DIRECTION ( 'NONE',  ( 1.000000000000000000, -0.000000000000000000, -0.000000000000000000 ) ) ;
#5758=CYLINDRICAL_SURFACE ( 'NONE', #4282, 7.499999999999992895 ) ;
#5759=ORIENTED_EDGE ( 'NONE', *, *, #4726, .T. ) ;
#5764=EDGE_CURVE ( 'NONE', #5277, #9148, #6446, .T. ) ;
#5765=CARTESIAN_POINT ( 'NONE',  ( 23.37500000054622973, 26.92701409722686634, 93.04388485072563242 ) ) ;
#5766=CARTESIAN_POINT ( 'NONE',  ( -5.000000000000004441, 20.00000000000000000, 145.0000000000000000 ) ) ;
#5768=CARTESIAN_POINT ( 'NONE',  ( -27.49999999999999645, 27.49999999999999645, 145.0000000000000000 ) ) ;
#5771=CYLINDRICAL_SURFACE ( 'NONE', #11762, 7.499999999999992895 ) ;
#5772=EDGE_LOOP ( 'NONE', ( #7767, #7420, #4230, #3336 ) ) ;
#5777=CARTESIAN_POINT ( 'NONE',  ( 39.17500000054623399, 26.92701409722686634, 88.54243821818162985 ) ) ;
#5778=CARTESIAN_POINT ( 'NONE',  ( 24.67500000054622689, 15.71886984736413773, 84.90069139318163138 ) ) ;
#5779=CARTESIAN_POINT ( 'NONE',  ( 28.99999999999998934, 20.00000000000000355, 83.29316153445364534 ) ) ;
#5780=DIRECTION ( 'NONE',  ( 1.000000000000000000, 0.000000000000000000, 0.000000000000000000 ) ) ;
#5781=CARTESIAN_POINT ( 'NONE',  ( 35.47500000054623115, 26.19570976099943493, 95.29460816699764791 ) ) ;
#5784=AXIS2_PLACEMENT_3D ( 'NONE', #432, #8171, #5379 ) ;
#5786=ORIENTED_EDGE ( 'NONE', *, *, #3179, .T. ) ;
#5789=CARTESIAN_POINT ( 'NONE',  ( 20.00000000000003908, 20.00000000000000000, 137.5000000000000000 ) ) ;
#5792=EDGE_CURVE ( 'NONE', #9392, #2848, #11391, .T. ) ;
#5793=CARTESIAN_POINT ( 'NONE',  ( 44.47500000054622404, 13.07298590277314432, 88.54243821818161564 ) ) ;
#5794=CYLINDRICAL_SURFACE ( 'NONE', #496, 7.499999999999992895 ) ;
#5795=EDGE_CURVE ( 'NONE', #5802, #1127, #9742, .T. ) ;
#5796=CARTESIAN_POINT ( 'NONE',  ( 45.27500000054622831, 26.92701409722686634, 88.54243821818162985 ) ) ;
#5797=CARTESIAN_POINT ( 'NONE',  ( 20.77500000054622120, 17.63344945572770328, 83.50966788445364841 ) ) ;
#5798=CARTESIAN_POINT ( 'NONE',  ( 44.39999999999999147, 12.86707612778636012, 93.11078899226572503 ) ) ;
#5800=CARTESIAN_POINT ( 'NONE',  ( 30.15000000109246159, 12.11403331821300533, 90.79316153445363113 ) ) ;
#5802=VERTEX_POINT ( 'NONE', #7461 ) ;
#5803=ORIENTED_EDGE ( 'NONE', *, *, #5689, .F. ) ;
#5804=CYLINDRICAL_SURFACE ( 'NONE', #4850, 7.499999999999992895 ) ;
#5806=DIRECTION ( 'NONE',  ( 1.000000000000000000, -0.000000000000000000, -0.000000000000000000 ) ) ;
#5808=CARTESIAN_POINT ( 'NONE',  ( 35.37500000054622973, 26.92701409722686634, 93.04388485072563242 ) ) ;
#5810=CARTESIAN_POINT ( 'NONE',  ( 27.50000000000000355, 27.49999999999999645, 145.0000000000000000 ) ) ;
#5811=ORIENTED_EDGE ( 'NONE', *, *, #261, .T. ) ;
#5815=CARTESIAN_POINT ( 'NONE',  ( 48.07500000054622546, 15.71886984736413417, 96.68563167572563088 ) ) ;
#5818=VERTEX_POINT ( 'NONE', #6567 ) ;
#5819=VECTOR ( 'NONE', #3754, 1000.000000000000000 ) ;
#5822=EDGE_CURVE ( 'NONE', #1088, #6810, #2214, .T. ) ;
#5826=CARTESIAN_POINT ( 'NONE',  ( 23.47500000054622760, 26.19570976099943849, 95.29460816699764791 ) ) ;
#5827=CARTESIAN_POINT ( 'NONE',  ( 29.99999999999998934, 20.00000000000000355, 98.29316153445363113 ) ) ;
#5828=FACE_OUTER_BOUND ( 'NONE', #984, .T. ) ;
#5829=LINE ( 'NONE', #11535, #10199 ) ;
#5834=EDGE_CURVE ( 'NONE', #10526, #9490, #4668, .T. ) ;
#5836=CARTESIAN_POINT ( 'NONE',  ( 27.67500000054622333, 24.28113015263587116, 96.68563167572563088 ) ) ;
#5838=CARTESIAN_POINT ( 'NONE',  ( 41.37500000054622262, 26.92701409722686634, 93.04388485072563242 ) ) ;
#5841=CARTESIAN_POINT ( 'NONE',  ( 28.87500000054622262, 20.00000000000000355, 83.50966788445364841 ) ) ;
#5842=CARTESIAN_POINT ( 'NONE',  ( 23.99999999999998579, 20.00000000000000355, 98.29316153445363113 ) ) ;
#5844=CARTESIAN_POINT ( 'NONE',  ( 33.27500000054621410, 27.65831843345427998, 90.79316153445363113 ) ) ;
#5846=FACE_OUTER_BOUND ( 'NONE', #1437, .T. ) ;
#5847=VERTEX_POINT ( 'NONE', #12531 ) ;
#5850=( BOUNDED_CURVE ( )  B_SPLINE_CURVE ( 2, ( #10360, #1796, #12279, #12338, #7702, #3698, #7641, #9426, #4657, #3636, #4785 ),
 .UNSPECIFIED., .F., .F. ) 
 B_SPLINE_CURVE_WITH_KNOTS ( ( 3, 2, 2, 2, 2, 3 ),
 ( 0.8333333333333333703, 0.8399999999999999689, 0.8466666666666666785, 0.8533333333333333881, 0.8599999999999999867, 0.8666666666666666963 ),
 .UNSPECIFIED. ) 
 CURVE ( )  GEOMETRIC_REPRESENTATION_ITEM ( )  RATIONAL_B_SPLINE_CURVE ( ( 1.000000000000000000, 0.9510565162951535312, 1.000000000000000000, 0.9510565162951535312, 1.000000000000000000, 0.9510565162951535312, 1.000000000000000000, 0.9510565162951535312, 1.000000000000000000, 0.9510565162951535312, 1.000000000000000000 ) ) 
 REPRESENTATION_ITEM ( '' )  );
#5852=VECTOR ( 'NONE', #11756, 1000.000000000000000 ) ;
#5853=CARTESIAN_POINT ( 'NONE',  ( 43.19999999999998863, 24.40838939219355197, 84.72553407664153724 ) ) ;
#5856=CARTESIAN_POINT ( 'NONE',  ( 46.77500000054622831, 17.63344945572770328, 83.50966788445364841 ) ) ;
#5858=CARTESIAN_POINT ( 'NONE',  ( 0.000000000000000000, 0.000000000000000000, 169.9999999999999716 ) ) ;
#5859=CARTESIAN_POINT ( 'NONE',  ( 46.27500000054622831, 13.07298590277314254, 93.04388485072563242 ) ) ;
#5860=CARTESIAN_POINT ( 'NONE',  ( 44.69999999999998153, 13.62011893735971135, 86.15790661882942914 ) ) ;
#5861=CARTESIAN_POINT ( 'NONE',  ( 38.99999999999998579, 20.00000000000000355, 83.29316153445364534 ) ) ;
#5862=CARTESIAN_POINT ( 'NONE',  ( -6.999999999999999112, 84.49999999999998579, 146.8533255156881978 ) ) ;
#5864=CARTESIAN_POINT ( 'NONE',  ( 31.45000000109246585, 24.40838939219354842, 96.86078899226572503 ) ) ;
#5866=ORIENTED_EDGE ( 'NONE', *, *, #4562, .F. ) ;
#5868=ORIENTED_EDGE ( 'NONE', *, *, #4791, .T. ) ;
#5871=CARTESIAN_POINT ( 'NONE',  ( 37.97500000054623115, 15.71886984736413417, 96.68563167572563088 ) ) ;
#5872=CARTESIAN_POINT ( 'NONE',  ( 41.07500000054622546, 24.28113015263587471, 84.90069139318163138 ) ) ;
#5875=DIRECTION ( 'NONE',  ( 1.000000000000000000, -0.000000000000000000, -0.000000000000000000 ) ) ;
#5878=CARTESIAN_POINT ( 'NONE',  ( 46.99999999999998579, 20.00000000000000355, 83.29316153445364534 ) ) ;
#5882=VERTEX_POINT ( 'NONE', #6064 ) ;
#5886=EDGE_CURVE ( 'NONE', #113, #5882, #9337, .T. ) ;
#5889=DIRECTION ( 'NONE',  ( -1.000000000000000000, -0.000000000000000000, -0.000000000000000000 ) ) ;
#5890=CYLINDRICAL_SURFACE ( 'NONE', #1205, 7.499999999999992895 ) ;
#5895=DIRECTION ( 'NONE',  ( 1.000000000000000000, -0.000000000000000000, -0.000000000000000000 ) ) ;
#5901=CARTESIAN_POINT ( 'NONE',  ( 46.79999999999999005, 15.59161060780646046, 84.72553407664153724 ) ) ;
#5902=CARTESIAN_POINT ( 'NONE',  ( 48.67500000054622689, 15.71886984736413773, 84.90069139318163138 ) ) ;
#5903=CARTESIAN_POINT ( 'NONE',  ( 33.67500000054622689, 22.36655054427230027, 98.07665518445361386 ) ) ;
#5904=CARTESIAN_POINT ( 'NONE',  ( 20.77500000054622120, 17.63344945572770328, 83.50966788445364841 ) ) ;
#5905=CARTESIAN_POINT ( 'NONE',  ( 22.99999999999998934, 20.00000000000000355, 83.29316153445364534 ) ) ;
#5908=CARTESIAN_POINT ( 'NONE',  ( 48.99999999999998579, 20.00000000000000355, 83.29316153445364534 ) ) ;
#5909=CARTESIAN_POINT ( 'NONE',  ( 30.17500000054623044, 13.07298590277314254, 93.04388485072563242 ) ) ;
#5914=EDGE_CURVE ( 'NONE', #10184, #3396, #3655, .T. ) ;
#5915=LINE ( 'NONE', #9784, #10639 ) ;
#5917=CARTESIAN_POINT ( 'NONE',  ( 37.07500000054622546, 24.28113015263587471, 84.90069139318163138 ) ) ;
#5918=CYLINDRICAL_SURFACE ( 'NONE', #6740, 7.499999999999992895 ) ;
#5920=CARTESIAN_POINT ( 'NONE',  ( 37.37500000054622262, 27.65831843345427998, 90.79316153445363113 ) ) ;
#5921=CARTESIAN_POINT ( 'NONE',  ( 44.79999999999998295, 15.59161060780646046, 84.72553407664153724 ) ) ;
#5925=CARTESIAN_POINT ( 'NONE',  ( 28.45000000109246585, 15.59161060780646046, 84.72553407664153724 ) ) ;
#5928=( BOUNDED_CURVE ( )  B_SPLINE_CURVE ( 2, ( #12389, #6667, #969, #4838, #9722, #7751, #8705, #13, #5853, #9476, #7815 ),
 .UNSPECIFIED., .F., .F. ) 
 B_SPLINE_CURVE_WITH_KNOTS ( ( 3, 2, 2, 2, 2, 3 ),
 ( 0.1999999999999999278, 0.2066666666666665819, 0.2133333333333332915, 0.2199999999999999456, 0.2266666666666666274, 0.2333333333333333093 ),
 .UNSPECIFIED. ) 
 CURVE ( )  GEOMETRIC_REPRESENTATION_ITEM ( )  RATIONAL_B_SPLINE_CURVE ( ( 1.000000000000000666, 0.9510565162951528650, 1.000000000000000000, 0.9510565162951535312, 1.000000000000000000, 0.9510565162951535312, 1.000000000000000000, 0.9510565162951535312, 1.000000000000000000, 0.9510565162951537532, 0.9999999999999997780 ) ) 
 REPRESENTATION_ITEM ( '' )  );
#5929=VERTEX_POINT ( 'NONE', #2606 ) ;
#5933=CARTESIAN_POINT ( 'NONE',  ( 35.87500000054622262, 17.63344945572769973, 98.07665518445361386 ) ) ;
#5934=CARTESIAN_POINT ( 'NONE',  ( 34.07500000054622546, 15.71886984736413417, 96.68563167572563088 ) ) ;
#5935=CIRCLE ( 'NONE', #4921, 7.499999999999978684 ) ;
#5939=CARTESIAN_POINT ( 'NONE',  ( 47.65000000109246514, 20.00000000000000355, 98.29316153445363113 ) ) ;
#5945=LINE ( 'NONE', #10821, #3171 ) ;
#5946=DIRECTION ( 'NONE',  ( 0.000000000000000000, 0.000000000000000000, -1.000000000000000000 ) ) ;
#5947=CARTESIAN_POINT ( 'NONE',  ( 20.27158385259953377, 22.00000000000000000, 152.2284161474004520 ) ) ;
#5954=CARTESIAN_POINT ( 'NONE',  ( 41.07500000054622546, 26.19570976099943493, 86.29171490190961435 ) ) ;
#5957=ORIENTED_EDGE ( 'NONE', *, *, #4429, .T. ) ;
#5959=SHAPE_DEFINITION_REPRESENTATION ( #4059, #7408 ) ;
#5962=CARTESIAN_POINT ( 'NONE',  ( 32.67500000054622689, 17.63344945572770328, 83.50966788445364841 ) ) ;
#5964=CARTESIAN_POINT ( 'NONE',  ( 23.39999999999998792, 27.13292387221364876, 88.47553407664153724 ) ) ;
#5965=CYLINDRICAL_SURFACE ( 'NONE', #3021, 7.499999999999992895 ) ;
#5966=CARTESIAN_POINT ( 'NONE',  ( 34.57500000054623257, 15.71886984736413773, 84.90069139318163138 ) ) ;
#5967=ORIENTED_EDGE ( 'NONE', *, *, #1568, .T. ) ;
#5968=EDGE_CURVE ( 'NONE', #4064, #7564, #12194, .T. ) ;
#5972=CARTESIAN_POINT ( 'NONE',  ( 49.35000000109246798, 26.37988106264029398, 95.42841645007781892 ) ) ;
#5975=DIRECTION ( 'NONE',  ( 1.000000000000000000, -0.000000000000000000, -0.000000000000000000 ) ) ;
#5976=CARTESIAN_POINT ( 'NONE',  ( 35.77500000054622831, 22.36655054427230027, 98.07665518445361386 ) ) ;
#5979=CARTESIAN_POINT ( 'NONE',  ( 49.57500000054623257, 24.28113015263587116, 96.68563167572563088 ) ) ;
#5980=CARTESIAN_POINT ( 'NONE',  ( 41.97500000054623115, 17.63344945572769973, 98.07665518445361386 ) ) ;
#5981=CARTESIAN_POINT ( 'NONE',  ( 45.49999999999997868, 27.88596668178699645, 90.79316153445363113 ) ) ;
#5982=VECTOR ( 'NONE', #4416, 1000.000000000000000 ) ;
#5983=DIRECTION ( 'NONE',  ( -0.000000000000000000, -0.000000000000000000, 1.000000000000000000 ) ) ;
#5987=CARTESIAN_POINT ( 'NONE',  ( 29.25000000109246301, 27.13292387221364876, 93.11078899226573924 ) ) ;
#5989=VERTEX_POINT ( 'NONE', #2260 ) ;
#5991=ORIENTED_EDGE ( 'NONE', *, *, #10351, .T. ) ;
#5995=DIRECTION ( 'NONE',  ( 0.000000000000000000, 0.000000000000000000, 1.000000000000000000 ) ) ;
#5996=LINE ( 'NONE', #10678, #7170 ) ;
#5997=CARTESIAN_POINT ( 'NONE',  ( 28.37500000054622618, 13.07298590277314432, 88.54243821818161564 ) ) ;
#5998=CARTESIAN_POINT ( 'NONE',  ( 32.37500000054621552, 12.34168156654572535, 90.79316153445363113 ) ) ;
#5999=CARTESIAN_POINT ( 'NONE',  ( 46.65000000109246514, 20.00000000000000355, 83.29316153445364534 ) ) ;
#6000=EDGE_CURVE ( 'NONE', #4846, #12355, #8263, .T. ) ;
#6005=CARTESIAN_POINT ( 'NONE',  ( -50.00000000000001421, 0.000000000000000000, 169.9999999999999716 ) ) ;
#6007=FACE_OUTER_BOUND ( 'NONE', #9286, .T. ) ;
#6009=LINE ( 'NONE', #6424, #1708 ) ;
#6011=DIRECTION ( 'NONE',  ( 0.000000000000000000, 0.000000000000000000, -1.000000000000000000 ) ) ;
#6013=CARTESIAN_POINT ( 'NONE',  ( 9.949532711038518329, 21.03606021117587233, 83.36056314470675943 ) ) ;
#6014=LINE ( 'NONE', #9888, #3419 ) ;
#6019=CARTESIAN_POINT ( 'NONE',  ( 42.97500000054623115, 24.28113015263587471, 84.90069139318163138 ) ) ;
#6021=ORIENTED_EDGE ( 'NONE', *, *, #729, .T. ) ;
#6022=CARTESIAN_POINT ( 'NONE',  ( 37.15000000109246514, 27.88596668178699645, 90.79316153445363113 ) ) ;
#6023=EDGE_CURVE ( 'NONE', #527, #10184, #8695, .T. ) ;
#6025=CARTESIAN_POINT ( 'NONE',  ( 23.27500000054622475, 26.92701409722686634, 88.54243821818162985 ) ) ;
#6027=CARTESIAN_POINT ( 'NONE',  ( 32.87500000054622973, 22.36655054427230382, 83.50966788445364841 ) ) ;
#6029=CARTESIAN_POINT ( 'NONE',  ( 24.69999999999998508, 13.62011893735971135, 86.15790661882942914 ) ) ;
#6030=DIRECTION ( 'NONE',  ( 1.000000000000000000, -0.000000000000000000, -0.000000000000000000 ) ) ;
#6031=CARTESIAN_POINT ( 'NONE',  ( 24.37500000054622618, 13.07298590277314432, 88.54243821818161564 ) ) ;
#6033=ORIENTED_EDGE ( 'NONE', *, *, #4314, .F. ) ;
#6034=VECTOR ( 'NONE', #2620, 1000.000000000000000 ) ;
#6037=ORIENTED_EDGE ( 'NONE', *, *, #2113, .T. ) ;
#6040=CARTESIAN_POINT ( 'NONE',  ( 37.47500000054622404, 26.92701409722686634, 93.04388485072563242 ) ) ;
#6044=CARTESIAN_POINT ( 'NONE',  ( 39.37500000054622262, 27.65831843345427998, 90.79316153445363113 ) ) ;
#6045=CARTESIAN_POINT ( 'NONE',  ( 39.89999999999999858, 22.43689772174679575, 98.29316153445363113 ) ) ;
#6047=CARTESIAN_POINT ( 'NONE',  ( 45.97500000054623115, 15.71886984736413417, 96.68563167572563088 ) ) ;
#6048=ORIENTED_EDGE ( 'NONE', *, *, #12350, .F. ) ;
#6049=EDGE_CURVE ( 'NONE', #7736, #5467, #11036, .T. ) ;
#6050=CARTESIAN_POINT ( 'NONE',  ( 29.55000000109246727, 22.43689772174679575, 98.29316153445363113 ) ) ;
#6054=ORIENTED_EDGE ( 'NONE', *, *, #3099, .F. ) ;
#6058=MANIFOLD_SOLID_BREP ( 'Thread1', #8096 ) ;
#6060=CARTESIAN_POINT ( 'NONE',  ( 30.37500000054622973, 13.07298590277314432, 88.54243821818161564 ) ) ;
#6061=CARTESIAN_POINT ( 'NONE',  ( 33.37500000054621552, 27.65831843345427998, 90.79316153445363113 ) ) ;
#6064=CARTESIAN_POINT ( 'NONE',  ( 43.65000000109246514, 20.00000000000000355, 98.29316153445363113 ) ) ;
#6066=VERTEX_POINT ( 'NONE', #11547 ) ;
#6067=CARTESIAN_POINT ( 'NONE',  ( 47.97500000054622404, 17.63344945572769973, 98.07665518445361386 ) ) ;
#6068=EDGE_CURVE ( 'NONE', #12402, #1690, #6851, .T. ) ;
#6070=VERTEX_POINT ( 'NONE', #2858 ) ;
#6076=EDGE_CURVE ( 'NONE', #9736, #3312, #4146, .T. ) ;
#6078=EDGE_CURVE ( 'NONE', #11262, #11877, #8514, .T. ) ;
#6081=CARTESIAN_POINT ( 'NONE',  ( 7.723680589930663309, 26.35394802911231693, 86.80164316431257987 ) ) ;
#6086=CARTESIAN_POINT ( 'NONE',  ( 41.37500000054622262, 26.92701409722686634, 93.04388485072563242 ) ) ;
#6090=AXIS2_PLACEMENT_3D ( 'NONE', #11368, #2611, #831 ) ;
#6091=CARTESIAN_POINT ( 'NONE',  ( 46.99999999999998579, 20.00000000000000355, 83.29316153445364534 ) ) ;
#6092=CARTESIAN_POINT ( 'NONE',  ( 44.87500000054622973, 20.00000000000000355, 83.50966788445364841 ) ) ;
#6093=CARTESIAN_POINT ( 'NONE',  ( 33.97500000054623115, 15.71886984736413417, 96.68563167572563088 ) ) ;
#6094=CARTESIAN_POINT ( 'NONE',  ( 20.67500000054622689, 15.71886984736413773, 84.90069139318163138 ) ) ;
#6095=CARTESIAN_POINT ( 'NONE',  ( 26.39999999999998792, 12.86707612778636012, 93.11078899226572503 ) ) ;
#6097=CARTESIAN_POINT ( 'NONE',  ( 24.67500000054622689, 17.63344945572770328, 83.50966788445364841 ) ) ;
#6100=CARTESIAN_POINT ( 'NONE',  ( 22.65000000109246514, 20.00000000000000355, 83.29316153445364534 ) ) ;
#6104=VERTEX_POINT ( 'NONE', #3106 ) ;
#6107=CARTESIAN_POINT ( 'NONE',  ( 39.17500000054621978, 26.19570976099943849, 86.29171490190961435 ) ) ;
#6109=CARTESIAN_POINT ( 'NONE',  ( 20.05000000109246372, 12.86707612778636012, 93.11078899226572503 ) ) ;
#6110=CARTESIAN_POINT ( 'NONE',  ( 41.39999999999999147, 27.13292387221364876, 88.47553407664153724 ) ) ;
#6112=CARTESIAN_POINT ( 'NONE',  ( 48.37500000054622973, 13.07298590277314432, 88.54243821818161564 ) ) ;
#6114=CARTESIAN_POINT ( 'NONE',  ( 23.25000000109246656, 27.13292387221364876, 93.11078899226573924 ) ) ;
#6120=CARTESIAN_POINT ( 'NONE',  ( -2.000000000000015543, 20.00000000000000355, 83.29316153445364534 ) ) ;
#6121=CARTESIAN_POINT ( 'NONE',  ( 41.65000000109246514, 20.00000000000000355, 98.29316153445363113 ) ) ;
#6123=CARTESIAN_POINT ( 'NONE',  ( 48.89999999999998437, 17.56310227825320069, 83.29316153445363113 ) ) ;
#6125=CARTESIAN_POINT ( 'NONE',  ( 30.87500000054622618, 22.36655054427230382, 83.50966788445364841 ) ) ;
#6126=CARTESIAN_POINT ( 'NONE',  ( 33.97500000054620983, 17.63344945572769973, 98.07665518445361386 ) ) ;
#6129=FACE_OUTER_BOUND ( 'NONE', #4612, .T. ) ;
#6131=CARTESIAN_POINT ( 'NONE',  ( 44.05000000109246372, 12.86707612778636012, 93.11078899226572503 ) ) ;
#6133=CARTESIAN_POINT ( 'NONE',  ( -36.00000000000001421, 77.00000000000000000, 154.3533255156881978 ) ) ;
#6134=EDGE_CURVE ( 'NONE', #3276, #5557, #264, .T. ) ;
#6139=CARTESIAN_POINT ( 'NONE',  ( 9.989732752402098015, 20.52140336093278350, 83.30683545822255098 ) ) ;
#6144=ADVANCED_FACE ( 'NONE', ( #3175 ), #5965, .F. ) ;
#6145=CARTESIAN_POINT ( 'NONE',  ( 43.07500000054622546, 26.19570976099943493, 86.29171490190961435 ) ) ;
#6152=CARTESIAN_POINT ( 'NONE',  ( 46.07500000054622546, 15.71886984736413417, 96.68563167572563088 ) ) ;
#6154=CARTESIAN_POINT ( 'NONE',  ( 31.37500000054622973, 26.92701409722686634, 93.04388485072563242 ) ) ;
#6155=CARTESIAN_POINT ( 'NONE',  ( 24.07500000054622546, 15.71886984736413417, 96.68563167572563088 ) ) ;
#6158=CARTESIAN_POINT ( 'NONE',  ( 27.67500000054623044, 22.36655054427230027, 98.07665518445361386 ) ) ;
#6160=CARTESIAN_POINT ( 'NONE',  ( 33.05000000109247082, 27.13292387221364876, 88.47553407664153724 ) ) ;
#6161=ORIENTED_EDGE ( 'NONE', *, *, #10279, .F. ) ;
#6162=ORIENTED_EDGE ( 'NONE', *, *, #11334, .T. ) ;
#6168=CARTESIAN_POINT ( 'NONE',  ( 36.57500000054621125, 13.80429023900056684, 86.29171490190961435 ) ) ;
#6170=CARTESIAN_POINT ( 'NONE',  ( 38.79999999999999005, 15.59161060780646046, 84.72553407664153724 ) ) ;
#6171=CARTESIAN_POINT ( 'NONE',  ( 44.87500000054623683, 22.36655054427230382, 83.50966788445364841 ) ) ;
#6174=CARTESIAN_POINT ( 'NONE',  ( 22.15000000109246869, 12.11403331821300533, 90.79316153445363113 ) ) ;
#6180=CARTESIAN_POINT ( 'NONE',  ( 40.75000000109245946, 22.43689772174679575, 83.29316153445363113 ) ) ;
#6183=CARTESIAN_POINT ( 'NONE',  ( -6.999999999999999112, 40.00000000000000000, 69.99999999999998579 ) ) ;
#6184=CARTESIAN_POINT ( 'NONE',  ( 27.87500000054622618, 17.63344945572769973, 98.07665518445361386 ) ) ;
#6185=CARTESIAN_POINT ( 'NONE',  ( 30.67500000054622333, 15.71886984736413773, 84.90069139318163138 ) ) ;
#6187=CARTESIAN_POINT ( 'NONE',  ( 22.35000000109246443, 13.62011893735970958, 86.15790661882942914 ) ) ;
#6189=CARTESIAN_POINT ( 'NONE',  ( 43.35000000109246088, 26.37988106264029398, 95.42841645007781892 ) ) ;
#6200=ADVANCED_FACE ( 'NONE', ( #1341 ), #387, .F. ) ;
#6207=EDGE_CURVE ( 'NONE', #11695, #527, #10121, .T. ) ;
#6209=ORIENTED_EDGE ( 'NONE', *, *, #10552, .T. ) ;
#6211=DIRECTION ( 'NONE',  ( 1.000000000000000000, -0.000000000000000000, -0.000000000000000000 ) ) ;
#6212=CARTESIAN_POINT ( 'NONE',  ( 43.77500000054622120, 22.36655054427230027, 98.07665518445361386 ) ) ;
#6214=CARTESIAN_POINT ( 'NONE',  ( 25.47500000054622760, 26.19570976099943849, 95.29460816699764791 ) ) ;
#6215=CARTESIAN_POINT ( 'NONE',  ( 7.617757055713122227, 13.51299916189778649, 86.99997826776774446 ) ) ;
#6218=CARTESIAN_POINT ( 'NONE',  ( 25.47500000054622760, 26.19570976099943493, 95.29460816699764791 ) ) ;
#6223=CARTESIAN_POINT ( 'NONE',  ( 10.00000000000000355, 20.00000000000000355, 83.29316153445363113 ) ) ;
#6227=EDGE_CURVE ( 'NONE', #9270, #3052, #5083, .T. ) ;
#6228=CARTESIAN_POINT ( 'NONE',  ( 34.37500000054621552, 12.34168156654572357, 90.79316153445363113 ) ) ;
#6229=CARTESIAN_POINT ( 'NONE',  ( -111.8465843842649292, 69.50000000000000000, 101.8533255156881978 ) ) ;
#6231=CARTESIAN_POINT ( 'NONE',  ( 34.67500000054622689, 15.71886984736413773, 84.90069139318163138 ) ) ;
#6232=CARTESIAN_POINT ( 'NONE',  ( 35.69999999999997442, 26.37988106264029398, 95.42841645007781892 ) ) ;
#6234=CARTESIAN_POINT ( 'NONE',  ( 44.77500000054623541, 20.00000000000000355, 83.50966788445364841 ) ) ;
#6236=CARTESIAN_POINT ( 'NONE',  ( 25.55000000109246372, 22.43689772174679575, 98.29316153445363113 ) ) ;
#6238=ORIENTED_EDGE ( 'NONE', *, *, #4994, .F. ) ;
#6240=ORIENTED_EDGE ( 'NONE', *, *, #6546, .F. ) ;
#6241=CARTESIAN_POINT ( 'NONE',  ( 21.35000000109246443, 26.37988106264029398, 95.42841645007781892 ) ) ;
#6243=CARTESIAN_POINT ( 'NONE',  ( -27.49999999999999645, 20.00000000000000355, 170.0000119999999697 ) ) ;
#6244=CARTESIAN_POINT ( 'NONE',  ( 33.17500000054622689, 26.92701409722686634, 88.54243821818162985 ) ) ;
#6245=CARTESIAN_POINT ( 'NONE',  ( 24.47500000054622404, 13.07298590277314432, 88.54243821818161564 ) ) ;
#6246=FACE_OUTER_BOUND ( 'NONE', #5085, .T. ) ;
#6247=DIRECTION ( 'NONE',  ( 0.000000000000000000, 1.000000000000000000, 0.000000000000000000 ) ) ;
#6249=EDGE_LOOP ( 'NONE', ( #4466, #503, #4141, #8285 ) ) ;
#6250=CARTESIAN_POINT ( 'NONE',  ( 43.25000000109246656, 27.13292387221364876, 93.11078899226573924 ) ) ;
#6258=( BOUNDED_CURVE ( )  B_SPLINE_CURVE ( 2, ( #6965, #1891, #2912, #6843, #59, #6022, #2978, #3922, #3318, #3985, #10704 ),
 .UNSPECIFIED., .F., .F. ) 
 B_SPLINE_CURVE_WITH_KNOTS ( ( 3, 2, 2, 2, 2, 3 ),
 ( 0.4000000000000001332, 0.4066666666666667873, 0.4133333333333334414, 0.4200000000000000955, 0.4266666666666668051, 0.4333333333333334592 ),
 .UNSPECIFIED. ) 
 CURVE ( )  GEOMETRIC_REPRESENTATION_ITEM ( )  RATIONAL_B_SPLINE_CURVE ( ( 0.9999999999999992228, 0.9510565162951543083, 1.000000000000000000, 0.9510565162951535312, 1.000000000000000000, 0.9510565162951535312, 1.000000000000000000, 0.9510565162951535312, 1.000000000000000000, 0.9510565162951527540, 1.000000000000000888 ) ) 
 REPRESENTATION_ITEM ( '' )  );
#6259=CIRCLE ( 'NONE', #6643, 7.499999999999978684 ) ;
#6267=ADVANCED_FACE ( 'NONE', ( #7290 ), #5148, .F. ) ;
#6274=CARTESIAN_POINT ( 'NONE',  ( 27.49999999999999645, 20.00000000000000355, 99.99999999999997158 ) ) ;
#6276=CARTESIAN_POINT ( 'NONE',  ( 43.87500000054622973, 20.00000000000000355, 98.07665518445361386 ) ) ;
#6277=EDGE_CURVE ( 'NONE', #10865, #7736, #12333, .T. ) ;
#6278=CARTESIAN_POINT ( 'NONE',  ( 24.27500000054622475, 12.34168156654572357, 90.79316153445363113 ) ) ;
#6281=FACE_OUTER_BOUND ( 'NONE', #3580, .T. ) ;
#6282=DIRECTION ( 'NONE',  ( 0.000000000000000000, 0.000000000000000000, -1.000000000000000000 ) ) ;
#6285=EDGE_LOOP ( 'NONE', ( #6054, #12478, #2676, #1661, #7264, #8513 ) ) ;
#6289=EDGE_LOOP ( 'NONE', ( #5957, #11835, #5106, #7017, #10949 ) ) ;
#6290=ADVANCED_FACE ( 'NONE', ( #4434 ), #2592, .F. ) ;
#6291=CARTESIAN_POINT ( 'NONE',  ( 31.37500000054622262, 27.65831843345427998, 90.79316153445363113 ) ) ;
#6293=ADVANCED_FACE ( 'NONE', ( #4375 ), #5334, .F. ) ;
#6294=CARTESIAN_POINT ( 'NONE',  ( 48.17500000054623399, 13.07298590277314254, 93.04388485072563242 ) ) ;
#6295=CARTESIAN_POINT ( 'NONE',  ( 36.77500000054622831, 17.63344945572770328, 83.50966788445364841 ) ) ;
#6296=CARTESIAN_POINT ( 'NONE',  ( 33.69999999999997442, 26.37988106264029398, 95.42841645007781892 ) ) ;
#6297=AXIS2_PLACEMENT_3D ( 'NONE', #5644, #11473, #636 ) ;
#6298=CARTESIAN_POINT ( 'NONE',  ( 46.77500000054622831, 20.00000000000000355, 83.50966788445364841 ) ) ;
#6300=CARTESIAN_POINT ( 'NONE',  ( 23.85000000109246443, 15.59161060780645691, 96.86078899226572503 ) ) ;
#6305=ORIENTED_EDGE ( 'NONE', *, *, #9707, .F. ) ;
#6308=DIRECTION ( 'NONE',  ( 0.000000000000000000, 0.000000000000000000, -1.000000000000000000 ) ) ;
#6310=DIRECTION ( 'NONE',  ( 1.000000000000000000, -0.000000000000000000, -0.000000000000000000 ) ) ;
#6312=CARTESIAN_POINT ( 'NONE',  ( 22.27500000054622475, 12.34168156654572535, 90.79316153445363113 ) ) ;
#6313=CARTESIAN_POINT ( 'NONE',  ( 28.17500000054621978, 13.80429023900056507, 95.29460816699764791 ) ) ;
#6315=DIRECTION ( 'NONE',  ( -1.000000000000000000, 0.000000000000000000, 0.000000000000000000 ) ) ;
#6316=EDGE_LOOP ( 'NONE', ( #715, #3759, #7183, #1539 ) ) ;
#6317=CARTESIAN_POINT ( 'NONE',  ( 44.45000000109246230, 15.59161060780646046, 84.72553407664153724 ) ) ;
#6323=CARTESIAN_POINT ( 'NONE',  ( 19.87500000054622973, 17.63344945572769973, 98.07665518445361386 ) ) ;
#6325=CYLINDRICAL_SURFACE ( 'NONE', #10701, 7.499999999999978684 ) ;
#6329=CARTESIAN_POINT ( 'NONE',  ( 23.99999999999998579, 20.00000000000000355, 98.29316153445363113 ) ) ;
#6330=ORIENTED_EDGE ( 'NONE', *, *, #4009, .F. ) ;
#6331=( BOUNDED_CURVE ( )  B_SPLINE_CURVE ( 3, ( #9764, #3981, #7858, #880 ),
 .UNSPECIFIED., .F., .F. ) 
 B_SPLINE_CURVE_WITH_KNOTS ( ( 4, 4 ),
 ( 4.712388980384689674, 6.283185307179586232 ),
 .UNSPECIFIED. ) 
 CURVE ( )  GEOMETRIC_REPRESENTATION_ITEM ( )  RATIONAL_B_SPLINE_CURVE ( ( 1.000000000000000000, 0.8047378541243649375, 0.8047378541243649375, 1.000000000000000000 ) ) 
 REPRESENTATION_ITEM ( '' )  );
#6334=ADVANCED_FACE ( 'NONE', ( #6465 ), #8189, .F. ) ;
#6336=CARTESIAN_POINT ( 'NONE',  ( 43.67500000054621978, 24.28113015263587116, 96.68563167572563088 ) ) ;
#6337=CARTESIAN_POINT ( 'NONE',  ( 28.37500000054622618, 13.07298590277314432, 88.54243821818161564 ) ) ;
#6338=DIRECTION ( 'NONE',  ( 0.000000000000000000, -1.000000000000000000, 0.000000000000000000 ) ) ;
#6339=CARTESIAN_POINT ( 'NONE',  ( -111.8465843842649292, 84.49999999999998579, 146.8533255156881978 ) ) ;
#6342=LINE ( 'NONE', #569, #7065 ) ;
#6347=ORIENTED_EDGE ( 'NONE', *, *, #1089, .T. ) ;
#6350=CARTESIAN_POINT ( 'NONE',  ( 35.07500000054622546, 24.28113015263587471, 84.90069139318163138 ) ) ;
#6352=CARTESIAN_POINT ( 'NONE',  ( 45.77500000054622831, 20.00000000000000355, 98.07665518445361386 ) ) ;
#6353=CARTESIAN_POINT ( 'NONE',  ( 34.77500000054622831, 17.63344945572770328, 83.50966788445364841 ) ) ;
#6354=CARTESIAN_POINT ( 'NONE',  ( 34.39999999999998437, 12.86707612778636012, 93.11078899226572503 ) ) ;
#6355=EDGE_CURVE ( 'NONE', #7325, #10212, #3328, .T. ) ;
#6357=CARTESIAN_POINT ( 'NONE',  ( 41.97500000054623115, 15.71886984736413417, 96.68563167572563088 ) ) ;
#6359=VECTOR ( 'NONE', #5806, 1000.000000000000000 ) ;
#6360=CARTESIAN_POINT ( 'NONE',  ( 26.35000000109246443, 13.62011893735971135, 86.15790661882942914 ) ) ;
#6366=EDGE_LOOP ( 'NONE', ( #3427, #4897, #3364, #7810, #8268, #4404 ) ) ;
#6368=CARTESIAN_POINT ( 'NONE',  ( 21.15000000109246514, 27.88596668178699645, 90.79316153445363113 ) ) ;
#6369=CARTESIAN_POINT ( 'NONE',  ( 34.72841614740047333, 18.00000000000000355, 170.0000119999999697 ) ) ;
#6370=CARTESIAN_POINT ( 'NONE',  ( 32.45000000109246940, 15.59161060780646046, 84.72553407664153724 ) ) ;
#6371=CARTESIAN_POINT ( 'NONE',  ( 21.57500000054622546, 24.28113015263587116, 96.68563167572563088 ) ) ;
#6372=CARTESIAN_POINT ( 'NONE',  ( 26.37500000054622618, 12.34168156654572535, 90.79316153445363113 ) ) ;
#6375=DIRECTION ( 'NONE',  ( 1.000000000000000000, -0.000000000000000000, -0.000000000000000000 ) ) ;
#6377=CARTESIAN_POINT ( 'NONE',  ( 43.65000000109246514, 20.00000000000000355, 98.29316153445363113 ) ) ;
#6378=ORIENTED_EDGE ( 'NONE', *, *, #9618, .T. ) ;
#6380=EDGE_CURVE ( 'NONE', #5465, #12457, #6342, .T. ) ;
#6381=ORIENTED_EDGE ( 'NONE', *, *, #1939, .F. ) ;
#6389=CARTESIAN_POINT ( 'NONE',  ( 41.99999999999998579, 20.00000000000000355, 98.29316153445363113 ) ) ;
#6393=ORIENTED_EDGE ( 'NONE', *, *, #9543, .F. ) ;
#6395=DIRECTION ( 'NONE',  ( 1.000000000000000000, -0.000000000000000000, -0.000000000000000000 ) ) ;
#6396=CARTESIAN_POINT ( 'NONE',  ( 28.79999999999999005, 15.59161060780646046, 84.72553407664153724 ) ) ;
#6397=CARTESIAN_POINT ( 'NONE',  ( 36.17500000054623399, 13.80429023900056507, 95.29460816699764791 ) ) ;
#6398=CARTESIAN_POINT ( 'NONE',  ( 25.87500000054622618, 17.63344945572769973, 98.07665518445361386 ) ) ;
#6400=CARTESIAN_POINT ( 'NONE',  ( 21.65000000109246514, 20.00000000000000355, 98.29316153445363113 ) ) ;
#6401=CYLINDRICAL_SURFACE ( 'NONE', #9818, 7.499999999999992895 ) ;
#6402=CARTESIAN_POINT ( 'NONE',  ( 31.19999999999998863, 24.40838939219355197, 84.72553407664153724 ) ) ;
#6403=( BOUNDED_CURVE ( )  B_SPLINE_CURVE ( 2, ( #2273, #8234, #1323, #5194, #9062, #1385, #5254, #1449, #3525, #11515, #5692 ),
 .UNSPECIFIED., .F., .F. ) 
 B_SPLINE_CURVE_WITH_KNOTS ( ( 3, 2, 2, 2, 2, 3 ),
 ( 0.9000000000000000222, 0.9066666666666666208, 0.9133333333333333304, 0.9200000000000000400, 0.9266666666666666385, 0.9333333333333333481 ),
 .UNSPECIFIED. ) 
 CURVE ( )  GEOMETRIC_REPRESENTATION_ITEM ( )  RATIONAL_B_SPLINE_CURVE ( ( 1.000000000000000000, 0.9510565162951535312, 1.000000000000000000, 0.9510565162951535312, 1.000000000000000000, 0.9510565162951535312, 1.000000000000000000, 0.9510565162951535312, 1.000000000000000000, 0.9510565162951535312, 1.000000000000000000 ) ) 
 REPRESENTATION_ITEM ( '' )  );
#6410=EDGE_CURVE ( 'NONE', #4126, #11823, #5354, .T. ) ;
#6411=CARTESIAN_POINT ( 'NONE',  ( 32.07500000054622546, 15.71886984736413417, 96.68563167572563088 ) ) ;
#6412=CARTESIAN_POINT ( 'NONE',  ( 47.27500000054622831, 27.65831843345427998, 90.79316153445363113 ) ) ;
#6413=CARTESIAN_POINT ( 'NONE',  ( 32.57500000054621836, 13.80429023900056684, 86.29171490190961435 ) ) ;
#6414=CARTESIAN_POINT ( 'NONE',  ( 38.39999999999999147, 12.86707612778636012, 93.11078899226572503 ) ) ;
#6416=CARTESIAN_POINT ( 'NONE',  ( 38.27500000054623541, 12.34168156654572535, 90.79316153445363113 ) ) ;
#6418=CARTESIAN_POINT ( 'NONE',  ( 19.95000000109246230, 13.62011893735971135, 95.42841645007781892 ) ) ;
#6421=EDGE_CURVE ( 'NONE', #3740, #8586, #3834, .T. ) ;
#6423=EDGE_LOOP ( 'NONE', ( #8068, #6775, #12029, #6305, #1921 ) ) ;
#6424=CARTESIAN_POINT ( 'NONE',  ( -50.00000000000001421, 69.50000000000000000, 146.8533255156881978 ) ) ;
#6425=CARTESIAN_POINT ( 'NONE',  ( 20.95000000109246230, 26.37988106264029398, 86.15790661882942914 ) ) ;
#6426=EDGE_CURVE ( 'NONE', #5428, #1420, #6523, .T. ) ;
#6430=CARTESIAN_POINT ( 'NONE',  ( 27.07500000054622902, 26.19570976099943493, 86.29171490190961435 ) ) ;
#6431=CARTESIAN_POINT ( 'NONE',  ( 25.37500000054622618, 27.65831843345427998, 90.79316153445363113 ) ) ;
#6433=ORIENTED_EDGE ( 'NONE', *, *, #11782, .F. ) ;
#6434=CARTESIAN_POINT ( 'NONE',  ( 37.75000000109246656, 17.56310227825320425, 98.29316153445363113 ) ) ;
#6442=CARTESIAN_POINT ( 'NONE',  ( 29.09999999999998721, 22.43689772174679575, 83.29316153445363113 ) ) ;
#6445=CARTESIAN_POINT ( 'NONE',  ( 38.65000000109246514, 20.00000000000000355, 83.29316153445364534 ) ) ;
#6446=LINE ( 'NONE', #1868, #4430 ) ;
#6449=CARTESIAN_POINT ( 'NONE',  ( 25.57500000054622546, 24.28113015263587116, 96.68563167572563088 ) ) ;
#6451=EDGE_CURVE ( 'NONE', #3740, #8002, #2659, .T. ) ;
#6453=VERTEX_POINT ( 'NONE', #11598 ) ;
#6458=CARTESIAN_POINT ( 'NONE',  ( 38.57500000054622546, 15.71886984736413773, 84.90069139318163138 ) ) ;
#6459=CARTESIAN_POINT ( 'NONE',  ( 35.67500000054622689, 24.28113015263587116, 96.68563167572563088 ) ) ;
#6460=CARTESIAN_POINT ( 'NONE',  ( 29.67500000054623044, 22.36655054427230027, 98.07665518445361386 ) ) ;
#6461=AXIS2_PLACEMENT_3D ( 'NONE', #199, #7162, #4055 ) ;
#6462=CARTESIAN_POINT ( 'NONE',  ( -50.00000000000001421, 40.00000000000000000, 169.9999999999999716 ) ) ;
#6464=CARTESIAN_POINT ( 'NONE',  ( 33.59999999999999432, 27.13292387221364876, 93.11078899226573924 ) ) ;
#6465=FACE_OUTER_BOUND ( 'NONE', #12460, .T. ) ;
#6471=CARTESIAN_POINT ( 'NONE',  ( 29.77500000054621765, 22.36655054427230027, 98.07665518445361386 ) ) ;
#6472=DIRECTION ( 'NONE',  ( 1.000000000000000000, -0.000000000000000000, -0.000000000000000000 ) ) ;
#6473=CARTESIAN_POINT ( 'NONE',  ( 43.87500000054622973, 17.63344945572769973, 98.07665518445361386 ) ) ;
#6474=CARTESIAN_POINT ( 'NONE',  ( 31.97500000054622760, 17.63344945572769973, 98.07665518445361386 ) ) ;
#6475=CARTESIAN_POINT ( 'NONE',  ( 30.99999999999998934, 20.00000000000000355, 83.29316153445364534 ) ) ;
#6477=CARTESIAN_POINT ( 'NONE',  ( 38.67500000054623399, 17.63344945572770328, 83.50966788445364841 ) ) ;
#6479=CARTESIAN_POINT ( 'NONE',  ( 48.97500000054622404, 24.28113015263587471, 84.90069139318163138 ) ) ;
#6483=ORIENTED_EDGE ( 'NONE', *, *, #7695, .F. ) ;
#6490=CARTESIAN_POINT ( 'NONE',  ( 24.67500000054622689, 17.63344945572770328, 83.50966788445364841 ) ) ;
#6491=CARTESIAN_POINT ( 'NONE',  ( 48.89999999999999147, 17.56310227825321135, 83.29316153445363113 ) ) ;
#6494=ORIENTED_EDGE ( 'NONE', *, *, #6380, .F. ) ;
#6495=CARTESIAN_POINT ( 'NONE',  ( 36.95000000109246230, 26.37988106264029398, 86.15790661882942914 ) ) ;
#6496=DIRECTION ( 'NONE',  ( 1.000000000000000000, -0.000000000000000000, 0.000000000000000000 ) ) ;
#6497=ORIENTED_EDGE ( 'NONE', *, *, #8153, .F. ) ;
#6498=DIRECTION ( 'NONE',  ( 0.000000000000000000, 0.000000000000000000, -1.000000000000000000 ) ) ;
#6507=DIRECTION ( 'NONE',  ( 0.000000000000000000, 0.000000000000000000, -1.000000000000000000 ) ) ;
#6509=CARTESIAN_POINT ( 'NONE',  ( 47.57500000054621125, 26.19570976099943493, 95.29460816699764791 ) ) ;
#6512=ORIENTED_EDGE ( 'NONE', *, *, #5253, .T. ) ;
#6514=( BOUNDED_CURVE ( )  B_SPLINE_CURVE ( 3, ( #5947, #8865, #1136, #9887 ),
 .UNSPECIFIED., .F., .F. ) 
 B_SPLINE_CURVE_WITH_KNOTS ( ( 4, 4 ),
 ( 3.411525449423196132, 4.712388980384689674 ),
 .UNSPECIFIED. ) 
 CURVE ( )  GEOMETRIC_REPRESENTATION_ITEM ( )  RATIONAL_B_SPLINE_CURVE ( ( 1.000000000000000000, 0.8638816171694809753, 0.8638816171694809753, 1.000000000000000000 ) ) 
 REPRESENTATION_ITEM ( '' )  );
#6516=CARTESIAN_POINT ( 'NONE',  ( 34.37500000054622973, 13.07298590277314432, 88.54243821818161564 ) ) ;
#6517=CARTESIAN_POINT ( 'NONE',  ( 40.17500000054622689, 13.80429023900056507, 95.29460816699764791 ) ) ;
#6518=CARTESIAN_POINT ( 'NONE',  ( 10.00000000000000355, 20.00000000000000355, 98.29316153445363113 ) ) ;
#6519=CARTESIAN_POINT ( 'NONE',  ( 35.65000000109246514, 20.00000000000000355, 98.29316153445363113 ) ) ;
#6521=EDGE_CURVE ( 'NONE', #10832, #8002, #10614, .T. ) ;
#6522=CARTESIAN_POINT ( 'NONE',  ( 33.09999999999998010, 22.43689772174679575, 83.29316153445363113 ) ) ;
#6523=LINE ( 'NONE', #7733, #9921 ) ;
#6525=FACE_OUTER_BOUND ( 'NONE', #2393, .T. ) ;
#6527=CARTESIAN_POINT ( 'NONE',  ( 24.77500000054622475, 17.63344945572770328, 83.50966788445364841 ) ) ;
#6529=VECTOR ( 'NONE', #8310, 1000.000000000000000 ) ;
#6530=CARTESIAN_POINT ( 'NONE',  ( 38.77500000054622831, 20.00000000000000355, 83.50966788445364841 ) ) ;
#6531=ADVANCED_FACE ( 'NONE', ( #4686 ), #10637, .F. ) ;
#6532=CARTESIAN_POINT ( 'NONE',  ( 26.17500000054622689, 13.80429023900056507, 95.29460816699764791 ) ) ;
#6533=CARTESIAN_POINT ( 'NONE',  ( 31.19999999999998863, 24.40838939219355197, 84.72553407664153724 ) ) ;
#6535=CARTESIAN_POINT ( 'NONE',  ( 42.57500000054623257, 15.71886984736413773, 84.90069139318163138 ) ) ;
#6537=CARTESIAN_POINT ( 'NONE',  ( 47.27500000054622831, 27.65831843345427998, 90.79316153445363113 ) ) ;
#6539=EDGE_LOOP ( 'NONE', ( #5967, #8270, #253, #10169, #12196 ) ) ;
#6545=CARTESIAN_POINT ( 'NONE',  ( 20.27158385259953377, 22.00000000000000000, 152.2284161474004520 ) ) ;
#6546=EDGE_CURVE ( 'NONE', #5153, #4064, #5829, .T. ) ;
#6547=CARTESIAN_POINT ( 'NONE',  ( 43.17500000054621978, 26.19570976099943849, 86.29171490190961435 ) ) ;
#6548=CARTESIAN_POINT ( 'NONE',  ( 20.59999999999998721, 12.86707612778636012, 88.47553407664152303 ) ) ;
#6549=CARTESIAN_POINT ( 'NONE',  ( 23.87500000054622973, 17.63344945572769973, 98.07665518445361386 ) ) ;
#6550=CARTESIAN_POINT ( 'NONE',  ( 47.19999999999998863, 24.40838939219355197, 84.72553407664153724 ) ) ;
#6554=ORIENTED_EDGE ( 'NONE', *, *, #879, .F. ) ;
#6555=CARTESIAN_POINT ( 'NONE',  ( 36.45000000109246940, 15.59161060780646046, 84.72553407664153724 ) ) ;
#6558=CARTESIAN_POINT ( 'NONE',  ( 49.99999999999998579, 0.000000000000000000, 69.99999999999998579 ) ) ;
#6559=EDGE_LOOP ( 'NONE', ( #3130, #7501, #8055, #6586 ) ) ;
#6562=AXIS2_PLACEMENT_3D ( 'NONE', #6243, #2374, #3322 ) ;
#6563=FACE_OUTER_BOUND ( 'NONE', #10549, .T. ) ;
#6567=CARTESIAN_POINT ( 'NONE',  ( -5.000000000000004441, 40.00000000000000000, 169.9999999999999716 ) ) ;
#6568=CARTESIAN_POINT ( 'NONE',  ( -2.000000000000015543, 20.00000000000000355, 98.29316153445363113 ) ) ;
#6570=CARTESIAN_POINT ( 'NONE',  ( 21.57500000054622546, 24.28113015263587116, 96.68563167572563088 ) ) ;
#6571=CARTESIAN_POINT ( 'NONE',  ( 46.25000000109246656, 12.86707612778636012, 88.47553407664152303 ) ) ;
#6579=CARTESIAN_POINT ( 'NONE',  ( 37.67500000054621978, 24.28113015263587116, 96.68563167572563088 ) ) ;
#6580=CARTESIAN_POINT ( 'NONE',  ( 20.47500000054622760, 13.80429023900056684, 86.29171490190961435 ) ) ;
#6584=DIRECTION ( 'NONE',  ( -0.7071067811865489050, -0.000000000000000000, -0.7071067811865460184 ) ) ;
#6585=CARTESIAN_POINT ( 'NONE',  ( 34.65000000109246514, 20.00000000000000355, 83.29316153445364534 ) ) ;
#6586=ORIENTED_EDGE ( 'NONE', *, *, #11552, .F. ) ;
#6588=DIRECTION ( 'NONE',  ( -0.000000000000000000, -0.000000000000000000, 1.000000000000000000 ) ) ;
#6589=CARTESIAN_POINT ( 'NONE',  ( 37.77500000054623541, 20.00000000000000355, 98.07665518445361386 ) ) ;
#6590=CARTESIAN_POINT ( 'NONE',  ( 28.67500000054622689, 15.71886984736413773, 84.90069139318163138 ) ) ;
#6591=CARTESIAN_POINT ( 'NONE',  ( 29.09999999999998721, 22.43689772174679575, 83.29316153445363113 ) ) ;
#6593=CARTESIAN_POINT ( 'NONE',  ( 33.99999999999998579, 20.00000000000000355, 98.29316153445363113 ) ) ;
#6594=CARTESIAN_POINT ( 'NONE',  ( 39.17500000054623399, 26.92701409722686634, 88.54243821818162985 ) ) ;
#6595=ORIENTED_EDGE ( 'NONE', *, *, #1352, .F. ) ;
#6596=CARTESIAN_POINT ( 'NONE',  ( 48.37500000054622973, 13.07298590277314432, 88.54243821818161564 ) ) ;
#6597=CARTESIAN_POINT ( 'NONE',  ( -5.000000000000000888, 0.000000000000000000, 169.9999999999999716 ) ) ;
#6598=ORIENTED_EDGE ( 'NONE', *, *, #1939, .T. ) ;
#6601=EDGE_CURVE ( 'NONE', #9736, #3374, #2072, .T. ) ;
#6602=CARTESIAN_POINT ( 'NONE',  ( 42.35000000109246798, 13.62011893735970958, 86.15790661882942914 ) ) ;
#6605=CARTESIAN_POINT ( 'NONE',  ( 43.07500000054622546, 24.28113015263587471, 84.90069139318163138 ) ) ;
#6606=CARTESIAN_POINT ( 'NONE',  ( 20.29999999999998650, 13.62011893735970958, 95.42841645007781892 ) ) ;
#6608=CARTESIAN_POINT ( 'NONE',  ( 45.77500000054622120, 22.36655054427230027, 98.07665518445361386 ) ) ;
#6609=CARTESIAN_POINT ( 'NONE',  ( 20.17500000054622689, 13.80429023900056507, 95.29460816699764791 ) ) ;
#6612=CARTESIAN_POINT ( 'NONE',  ( 19.99999999999998579, 20.00000000000000355, 98.29316153445363113 ) ) ;
#6614=CARTESIAN_POINT ( 'NONE',  ( 40.35000000109246798, 13.62011893735971135, 86.15790661882942914 ) ) ;
#6628=CARTESIAN_POINT ( 'NONE',  ( 21.27500000054622831, 27.65831843345427998, 90.79316153445363113 ) ) ;
#6631=DIRECTION ( 'NONE',  ( 0.000000000000000000, 0.000000000000000000, -1.000000000000000000 ) ) ;
#6635=DIRECTION ( 'NONE',  ( 1.000000000000000000, -0.000000000000000000, -0.000000000000000000 ) ) ;
#6638=ADVANCED_FACE ( 'NONE', ( #3979 ), #8868, .F. ) ;
#6639=CARTESIAN_POINT ( 'NONE',  ( 9.685273772782807100, 17.49881738785535745, 97.86827095828408574 ) ) ;
#6640=DIRECTION ( 'NONE',  ( 0.000000000000000000, 0.000000000000000000, -1.000000000000000000 ) ) ;
#6642=CARTESIAN_POINT ( 'NONE',  ( 26.05000000109246727, 12.86707612778636012, 93.11078899226572503 ) ) ;
#6643=AXIS2_PLACEMENT_3D ( 'NONE', #5766, #9635, #690 ) ;
#6645=ORIENTED_EDGE ( 'NONE', *, *, #12180, .T. ) ;
#6649=CARTESIAN_POINT ( 'NONE',  ( 27.77500000054622475, 22.36655054427230027, 98.07665518445361386 ) ) ;
#6650=CARTESIAN_POINT ( 'NONE',  ( 35.99999999999999289, 20.00000000000000355, 98.29316153445363113 ) ) ;
#6651=CARTESIAN_POINT ( 'NONE',  ( 40.77500000054622831, 20.00000000000000355, 83.50966788445364841 ) ) ;
#6653=CARTESIAN_POINT ( 'NONE',  ( 29.97500000054622404, 17.63344945572769973, 98.07665518445361386 ) ) ;
#6654=CARTESIAN_POINT ( 'NONE',  ( 29.19999999999998508, 24.40838939219355197, 84.72553407664153724 ) ) ;
#6655=CARTESIAN_POINT ( 'NONE',  ( 30.09999999999998721, 17.56310227825320425, 98.29316153445363113 ) ) ;
#6656=CARTESIAN_POINT ( 'NONE',  ( 32.67500000054622689, 17.63344945572770328, 83.50966788445364841 ) ) ;
#6657=EDGE_CURVE ( 'NONE', #3847, #2033, #1325, .T. ) ;
#6659=CARTESIAN_POINT ( 'NONE',  ( 46.47500000054623115, 13.80429023900056684, 86.29171490190961435 ) ) ;
#6660=CARTESIAN_POINT ( 'NONE',  ( 28.35000000109246443, 13.62011893735970958, 86.15790661882942914 ) ) ;
#6662=VECTOR ( 'NONE', #7070, 1000.000000000000000 ) ;
#6664=ORIENTED_EDGE ( 'NONE', *, *, #9294, .T. ) ;
#6667=CARTESIAN_POINT ( 'NONE',  ( 43.89999999999999147, 22.43689772174677088, 98.29316153445365956 ) ) ;
#6669=CARTESIAN_POINT ( 'NONE',  ( 45.77500000054622120, 22.36655054427230027, 98.07665518445361386 ) ) ;
#6670=CARTESIAN_POINT ( 'NONE',  ( -50.00000000000001421, 20.00000000000000000, 145.0000000000000000 ) ) ;
#6671=LINE ( 'NONE', #12515, #5819 ) ;
#6672=CARTESIAN_POINT ( 'NONE',  ( 42.67500000054622689, 15.71886984736413773, 84.90069139318163138 ) ) ;
#6673=CARTESIAN_POINT ( 'NONE',  ( 47.69999999999999574, 26.37988106264029398, 95.42841645007781892 ) ) ;
#6675=EDGE_CURVE ( 'NONE', #2798, #2989, #7794, .T. ) ;
#6677=ORIENTED_EDGE ( 'NONE', *, *, #4049, .T. ) ;
#6678=CARTESIAN_POINT ( 'NONE',  ( 39.45000000109246230, 24.40838939219354842, 96.86078899226572503 ) ) ;
#6680=VERTEX_POINT ( 'NONE', #10699 ) ;
#6684=CARTESIAN_POINT ( 'NONE',  ( -50.00000000000001421, 55.00000000000000000, 166.8533255156881694 ) ) ;
#6685=EDGE_CURVE ( 'NONE', #5212, #9148, #7920, .T. ) ;
#6688=EDGE_CURVE ( 'NONE', #2848, #5434, #1451, .T. ) ;
#6691=ORIENTED_EDGE ( 'NONE', *, *, #10824, .F. ) ;
#6695=CARTESIAN_POINT ( 'NONE',  ( 22.07500000054622546, 13.80429023900056507, 95.29460816699764791 ) ) ;
#6697=DIRECTION ( 'NONE',  ( 1.000000000000000000, -0.000000000000000000, -0.000000000000000000 ) ) ;
#6698=DIRECTION ( 'NONE',  ( -0.000000000000000000, -0.000000000000000000, 1.000000000000000000 ) ) ;
#6699=ORIENTED_EDGE ( 'NONE', *, *, #6227, .T. ) ;
#6704=CARTESIAN_POINT ( 'NONE',  ( 20.97500000054622760, 24.28113015263587471, 84.90069139318163138 ) ) ;
#6705=LINE ( 'NONE', #4617, #7469 ) ;
#6708=CARTESIAN_POINT ( 'NONE',  ( 25.95000000109246230, 13.62011893735970958, 95.42841645007781892 ) ) ;
#6714=CARTESIAN_POINT ( 'NONE',  ( 27.17500000054621623, 26.19570976099943849, 86.29171490190961435 ) ) ;
#6715=CARTESIAN_POINT ( 'NONE',  ( 47.97500000054623115, 17.63344945572769973, 98.07665518445361386 ) ) ;
#6716=CARTESIAN_POINT ( 'NONE',  ( 40.37500000054622973, 13.07298590277314432, 88.54243821818161564 ) ) ;
#6717=CARTESIAN_POINT ( 'NONE',  ( 25.47500000054622404, 26.92701409722686634, 93.04388485072563242 ) ) ;
#6718=CARTESIAN_POINT ( 'NONE',  ( 29.89999999999998437, 22.43689772174679575, 98.29316153445363113 ) ) ;
#6719=CARTESIAN_POINT ( 'NONE',  ( 34.89999999999997726, 17.56310227825320425, 83.29316153445363113 ) ) ;
#6720=CARTESIAN_POINT ( 'NONE',  ( 30.77500000054622831, 20.00000000000000355, 83.50966788445364841 ) ) ;
#6724=CARTESIAN_POINT ( 'NONE',  ( -50.00000000000001421, 18.00000000000000355, 152.2284161474004520 ) ) ;
#6726=( BOUNDED_CURVE ( )  B_SPLINE_CURVE ( 2, ( #1614, #663, #2875, #8711, #6736, #8833, #5798, #23, #6867, #88, #1048 ),
 .UNSPECIFIED., .F., .F. ) 
 B_SPLINE_CURVE_WITH_KNOTS ( ( 3, 2, 2, 2, 2, 3 ),
 ( 0.1666666666666665741, 0.1733333333333332560, 0.1799999999999999101, 0.1866666666666665919, 0.1933333333333332460, 0.1999999999999999278 ),
 .UNSPECIFIED. ) 
 CURVE ( )  GEOMETRIC_REPRESENTATION_ITEM ( )  RATIONAL_B_SPLINE_CURVE ( ( 1.000000000000000666, 0.9510565162951529761, 1.000000000000000000, 0.9510565162951535312, 1.000000000000000000, 0.9510565162951535312, 1.000000000000000000, 0.9510565162951535312, 1.000000000000000000, 0.9510565162951540863, 0.9999999999999994449 ) ) 
 REPRESENTATION_ITEM ( '' )  );
#6729=CARTESIAN_POINT ( 'NONE',  ( 44.77500000054622831, 17.63344945572770328, 83.50966788445364841 ) ) ;
#6730=CARTESIAN_POINT ( 'NONE',  ( 20.39999999999998792, 12.86707612778636012, 93.11078899226572503 ) ) ;
#6733=CARTESIAN_POINT ( 'NONE',  ( 44.07500000054622546, 15.71886984736413417, 96.68563167572563088 ) ) ;
#6734=CARTESIAN_POINT ( 'NONE',  ( 46.59999999999998721, 12.86707612778636012, 88.47553407664152303 ) ) ;
#6735=CARTESIAN_POINT ( 'NONE',  ( 45.99999999999998579, 20.00000000000000355, 98.29316153445363113 ) ) ;
#6736=CARTESIAN_POINT ( 'NONE',  ( 44.59999999999998721, 12.86707612778636012, 88.47553407664152303 ) ) ;
#6739=ADVANCED_FACE ( 'NONE', ( #11024 ), #11086, .F. ) ;
#6740=AXIS2_PLACEMENT_3D ( 'NONE', #11625, #2240, #973 ) ;
#6741=CARTESIAN_POINT ( 'NONE',  ( 32.95000000109246230, 26.37988106264029398, 86.15790661882942914 ) ) ;
#6743=ORIENTED_EDGE ( 'NONE', *, *, #8159, .F. ) ;
#6747=DIRECTION ( 'NONE',  ( 0.000000000000000000, 0.000000000000000000, -1.000000000000000000 ) ) ;
#6750=CARTESIAN_POINT ( 'NONE',  ( 37.47500000054623825, 26.19570976099943493, 95.29460816699764791 ) ) ;
#6752=DIRECTION ( 'NONE',  ( 1.000000000000000000, 0.000000000000000000, 0.000000000000000000 ) ) ;
#6753=ORIENTED_EDGE ( 'NONE', *, *, #4865, .F. ) ;
#6757=CARTESIAN_POINT ( 'NONE',  ( 47.97500000054623115, 17.63344945572769973, 98.07665518445361386 ) ) ;
#6758=ORIENTED_EDGE ( 'NONE', *, *, #952, .T. ) ;
#6759=CYLINDRICAL_SURFACE ( 'NONE', #7000, 7.500000000000000000 ) ;
#6761=EDGE_LOOP ( 'NONE', ( #8609, #12094, #3108, #6033 ) ) ;
#6762=VECTOR ( 'NONE', #1404, 1000.000000000000000 ) ;
#6763=VERTEX_POINT ( 'NONE', #8237 ) ;
#6765=ADVANCED_FACE ( 'NONE', ( #7337 ), #7148, .F. ) ;
#6766=CARTESIAN_POINT ( 'NONE',  ( 21.79999999999998650, 24.40838939219354842, 96.86078899226572503 ) ) ;
#6772=CARTESIAN_POINT ( 'NONE',  ( -24.10660171779822747, 84.49999999999998579, 151.2467237978899846 ) ) ;
#6775=ORIENTED_EDGE ( 'NONE', *, *, #2850, .T. ) ;
#6778=CARTESIAN_POINT ( 'NONE',  ( 28.07500000054622546, 15.71886984736413417, 96.68563167572563088 ) ) ;
#6780=CARTESIAN_POINT ( 'NONE',  ( 37.97500000054623115, 15.71886984736413417, 96.68563167572563088 ) ) ;
#6781=CARTESIAN_POINT ( 'NONE',  ( 29.87500000054622618, 20.00000000000000355, 98.07665518445361386 ) ) ;
#6782=CARTESIAN_POINT ( 'NONE',  ( 20.19999999999998863, 15.59161060780645691, 96.86078899226572503 ) ) ;
#6784=CARTESIAN_POINT ( 'NONE',  ( 32.77500000054622831, 20.00000000000000355, 83.50966788445364841 ) ) ;
#6789=EDGE_LOOP ( 'NONE', ( #4326, #7309, #4351, #5025 ) ) ;
#6790=VECTOR ( 'NONE', #6884, 1000.000000000000000 ) ;
#6793=DIRECTION ( 'NONE',  ( 0.000000000000000000, 0.000000000000000000, -1.000000000000000000 ) ) ;
#6796=CARTESIAN_POINT ( 'NONE',  ( 45.57500000054621125, 26.19570976099943849, 95.29460816699764791 ) ) ;
#6797=FACE_OUTER_BOUND ( 'NONE', #7166, .T. ) ;
#6799=CARTESIAN_POINT ( 'NONE',  ( 45.17500000054621978, 26.19570976099943493, 86.29171490190961435 ) ) ;
#6800=CARTESIAN_POINT ( 'NONE',  ( 42.49999999999999289, 12.11403331821300533, 90.79316153445363113 ) ) ;
#6801=CARTESIAN_POINT ( 'NONE',  ( 40.69999999999998863, 13.62011893735970958, 86.15790661882942914 ) ) ;
#6802=EDGE_CURVE ( 'NONE', #12457, #7564, #8111, .T. ) ;
#6805=CARTESIAN_POINT ( 'NONE',  ( 32.45000000109246940, 15.59161060780646046, 84.72553407664153724 ) ) ;
#6807=ORIENTED_EDGE ( 'NONE', *, *, #4196, .F. ) ;
#6808=( BOUNDED_CURVE ( )  B_SPLINE_CURVE ( 2, ( #4250, #11097, #8186, #5268, #5208, #4432, #5331, #5395, #2348, #7097, #9267 ),
 .UNSPECIFIED., .F., .F. ) 
 B_SPLINE_CURVE_WITH_KNOTS ( ( 3, 2, 2, 2, 2, 3 ),
 ( 0.1333333333333332205, 0.1399999999999999023, 0.1466666666666665564, 0.1533333333333332382, 0.1599999999999999201, 0.1666666666666665741 ),
 .UNSPECIFIED. ) 
 CURVE ( )  GEOMETRIC_REPRESENTATION_ITEM ( )  RATIONAL_B_SPLINE_CURVE ( ( 1.000000000000000888, 0.9510565162951527540, 1.000000000000000000, 0.9510565162951535312, 1.000000000000000000, 0.9510565162951535312, 1.000000000000000000, 0.9510565162951535312, 1.000000000000000000, 0.9510565162951541973, 0.9999999999999993339 ) ) 
 REPRESENTATION_ITEM ( '' )  );
#6810=VERTEX_POINT ( 'NONE', #3344 ) ;
#6814=CIRCLE ( 'NONE', #8246, 7.499999999999992895 ) ;
#6816=CARTESIAN_POINT ( 'NONE',  ( 37.57500000054622546, 24.28113015263587116, 96.68563167572563088 ) ) ;
#6817=CARTESIAN_POINT ( 'NONE',  ( 38.27500000054622831, 13.07298590277314254, 93.04388485072563242 ) ) ;
#6818=CARTESIAN_POINT ( 'NONE',  ( 44.15000000109246514, 12.11403331821300533, 90.79316153445363113 ) ) ;
#6819=CARTESIAN_POINT ( 'NONE',  ( 4.999999999999997335, 20.00000000000000000, 145.0000000000000000 ) ) ;
#6820=EDGE_LOOP ( 'NONE', ( #12489, #1277, #8350, #9794 ) ) ;
#6822=CARTESIAN_POINT ( 'NONE',  ( 48.85000000109246088, 24.40838939219355197, 84.72553407664153724 ) ) ;
#6830=ORIENTED_EDGE ( 'NONE', *, *, #9294, .F. ) ;
#6832=ADVANCED_FACE ( 'NONE', ( #5696 ), #12289, .F. ) ;
#6834=AXIS2_PLACEMENT_3D ( 'NONE', #7005, #162, #4019 ) ;
#6835=CARTESIAN_POINT ( 'NONE',  ( 9.238455078247341135, 23.85215916112258228, 84.34042123683411774 ) ) ;
#6836=LINE ( 'NONE', #9952, #11513 ) ;
#6838=DIRECTION ( 'NONE',  ( -0.000000000000000000, -1.000000000000000000, -0.000000000000000000 ) ) ;
#6839=EDGE_CURVE ( 'NONE', #589, #9944, #1151, .T. ) ;
#6840=CARTESIAN_POINT ( 'NONE',  ( 26.25000000109246656, 12.86707612778636012, 88.47553407664152303 ) ) ;
#6843=CARTESIAN_POINT ( 'NONE',  ( 37.35000000109246088, 26.37988106264029398, 95.42841645007781892 ) ) ;
#6845=CARTESIAN_POINT ( 'NONE',  ( 19.97500000054622404, 17.63344945572769973, 98.07665518445361386 ) ) ;
#6846=CARTESIAN_POINT ( 'NONE',  ( 49.67500000054622689, 24.28113015263587116, 96.68563167572563088 ) ) ;
#6847=CARTESIAN_POINT ( 'NONE',  ( 34.47500000054623115, 13.80429023900056684, 86.29171490190961435 ) ) ;
#6849=CARTESIAN_POINT ( 'NONE',  ( 24.17500000054622689, 13.80429023900056507, 95.29460816699764791 ) ) ;
#6850=CARTESIAN_POINT ( 'NONE',  ( 25.29999999999998650, 26.37988106264029398, 86.15790661882942914 ) ) ;
#6851=LINE ( 'NONE', #10524, #10707 ) ;
#6852=CARTESIAN_POINT ( 'NONE',  ( 30.27500000054623186, 12.34168156654572535, 90.79316153445363113 ) ) ;
#6853=ORIENTED_EDGE ( 'NONE', *, *, #5914, .F. ) ;
#6856=DIRECTION ( 'NONE',  ( 1.000000000000000000, -0.000000000000000000, -0.000000000000000000 ) ) ;
#6857=ORIENTED_EDGE ( 'NONE', *, *, #10906, .T. ) ;
#6861=CARTESIAN_POINT ( 'NONE',  ( 38.07500000054622546, 15.71886984736413417, 96.68563167572563088 ) ) ;
#6862=FACE_OUTER_BOUND ( 'NONE', #114, .T. ) ;
#6863=PLANE ( 'NONE',  #10262 ) ;
#6864=CARTESIAN_POINT ( 'NONE',  ( 39.57500000054623257, 26.19570976099943493, 95.29460816699764791 ) ) ;
#6865=CARTESIAN_POINT ( 'NONE',  ( 45.69999999999999574, 26.37988106264029398, 95.42841645007781892 ) ) ;
#6866=CARTESIAN_POINT ( 'NONE',  ( 40.39999999999999147, 12.86707612778636012, 93.11078899226572503 ) ) ;
#6867=CARTESIAN_POINT ( 'NONE',  ( 44.19999999999998863, 15.59161060780645691, 96.86078899226572503 ) ) ;
#6870=CARTESIAN_POINT ( 'NONE',  ( 30.75000000109246301, 22.43689772174679575, 83.29316153445363113 ) ) ;
#6872=ORIENTED_EDGE ( 'NONE', *, *, #7376, .F. ) ;
#6878=CARTESIAN_POINT ( 'NONE',  ( 37.37500000054622973, 26.92701409722686634, 93.04388485072563242 ) ) ;
#6879=CARTESIAN_POINT ( 'NONE',  ( 30.27500000054622475, 13.07298590277314254, 93.04388485072563242 ) ) ;
#6884=DIRECTION ( 'NONE',  ( 1.000000000000000000, 0.000000000000000000, 0.000000000000000000 ) ) ;
#6885=ORIENTED_EDGE ( 'NONE', *, *, #6657, .T. ) ;
#6888=ORIENTED_EDGE ( 'NONE', *, *, #6000, .F. ) ;
#6891=VECTOR ( 'NONE', #8315, 1000.000000000000000 ) ;
#6892=CARTESIAN_POINT ( 'NONE',  ( -34.99999999999997868, 20.00000000000000000, 137.5000000000000000 ) ) ;
#6894=CARTESIAN_POINT ( 'NONE',  ( 37.39999999999999147, 27.13292387221364876, 88.47553407664153724 ) ) ;
#6898=CARTESIAN_POINT ( 'NONE',  ( 41.27500000054622831, 27.65831843345427998, 90.79316153445363113 ) ) ;
#6899=CARTESIAN_POINT ( 'NONE',  ( -6.999999999999999112, 77.00000000000000000, 94.35332551568819781 ) ) ;
#6903=ADVANCED_FACE ( 'NONE', ( #803 ), #2893, .F. ) ;
#6906=CARTESIAN_POINT ( 'NONE',  ( 33.27500000054622120, 27.65831843345427998, 90.79316153445363113 ) ) ;
#6908=CARTESIAN_POINT ( 'NONE',  ( 25.49999999999998934, 27.88596668178699645, 90.79316153445363113 ) ) ;
#6910=CARTESIAN_POINT ( 'NONE',  ( 34.37500000054622973, 13.07298590277314432, 88.54243821818161564 ) ) ;
#6914=ORIENTED_EDGE ( 'NONE', *, *, #2881, .T. ) ;
#6915=CARTESIAN_POINT ( 'NONE',  ( 49.55000000109246372, 22.43689772174679575, 98.29316153445363113 ) ) ;
#6917=DIRECTION ( 'NONE',  ( 0.000000000000000000, -0.000000000000000000, 1.000000000000000000 ) ) ;
#6920=CARTESIAN_POINT ( 'NONE',  ( 39.67500000054622689, 24.28113015263587116, 96.68563167572563088 ) ) ;
#6921=CARTESIAN_POINT ( 'NONE',  ( 44.99999999999999289, 20.00000000000000355, 83.29316153445364534 ) ) ;
#6923=( BOUNDED_CURVE ( )  B_SPLINE_CURVE ( 2, ( #9028, #3120, #148, #7175, #11814, #10860, #4203, #10044, #7049, #2170, #10789 ),
 .UNSPECIFIED., .F., .F. ) 
 B_SPLINE_CURVE_WITH_KNOTS ( ( 3, 2, 2, 2, 2, 3 ),
 ( 0.7666666666666666075, 0.7733333333333332060, 0.7799999999999999156, 0.7866666666666666252, 0.7933333333333333348, 0.8000000000000000444 ),
 .UNSPECIFIED. ) 
 CURVE ( )  GEOMETRIC_REPRESENTATION_ITEM ( )  RATIONAL_B_SPLINE_CURVE ( ( 1.000000000000000888, 0.9510565162951527540, 1.000000000000000000, 0.9510565162951535312, 1.000000000000000000, 0.9510565162951535312, 1.000000000000000000, 0.9510565162951535312, 1.000000000000000000, 0.9510565162951535312, 1.000000000000000000 ) ) 
 REPRESENTATION_ITEM ( '' )  );
#6924=CARTESIAN_POINT ( 'NONE',  ( 42.89999999999998437, 17.56310227825321135, 83.29316153445363113 ) ) ;
#6926=DIRECTION ( 'NONE',  ( -0.000000000000000000, -0.000000000000000000, 1.000000000000000000 ) ) ;
#6928=CARTESIAN_POINT ( 'NONE',  ( 34.35000000109246798, 13.62011893735971135, 86.15790661882942914 ) ) ;
#6934=LINE ( 'NONE', #7895, #965 ) ;
#6936=CARTESIAN_POINT ( 'NONE',  ( 29.77500000054622831, 20.00000000000000355, 98.07665518445361386 ) ) ;
#6937=CARTESIAN_POINT ( 'NONE',  ( 29.17500000054622333, 26.19570976099943493, 86.29171490190961435 ) ) ;
#6938=AXIS2_PLACEMENT_3D ( 'NONE', #5715, #5473, #8501 ) ;
#6941=CARTESIAN_POINT ( 'NONE',  ( 34.72841614740047333, 22.00000000000000000, 152.2284161474004520 ) ) ;
#6943=CARTESIAN_POINT ( 'NONE',  ( 49.17500000054622689, 26.19570976099943849, 86.29171490190961435 ) ) ;
#6947=ADVANCED_FACE ( 'NONE', ( #10499 ), #12534, .F. ) ;
#6952=AXIS2_PLACEMENT_3D ( 'NONE', #7984, #4105, #9954 ) ;
#6955=CARTESIAN_POINT ( 'NONE',  ( 7.621040678280055047, 26.47631533951529192, 87.00314373824969039 ) ) ;
#6959=DIRECTION ( 'NONE',  ( 0.000000000000000000, 0.000000000000000000, 1.000000000000000000 ) ) ;
#6960=CARTESIAN_POINT ( 'NONE',  ( 10.00000000000000355, 20.00000000000000355, 109.9999999999999858 ) ) ;
#6961=CARTESIAN_POINT ( 'NONE',  ( 40.37500000054622973, 13.07298590277314432, 88.54243821818161564 ) ) ;
#6964=EDGE_LOOP ( 'NONE', ( #11747, #8178, #4208, #2427 ) ) ;
#6965=CARTESIAN_POINT ( 'NONE',  ( 37.65000000109246514, 20.00000000000000355, 98.29316153445363113 ) ) ;
#6968=AXIS2_PLACEMENT_3D ( 'NONE', #5552, #10294, #12209 ) ;
#6969=CARTESIAN_POINT ( 'NONE',  ( 28.99999999999998934, 20.00000000000000355, 83.29316153445364534 ) ) ;
#6972=CARTESIAN_POINT ( 'NONE',  ( 32.17500000054622689, 13.07298590277314254, 93.04388485072563242 ) ) ;
#6973=CARTESIAN_POINT ( 'NONE',  ( 21.07500000054622191, 24.28113015263587471, 84.90069139318163138 ) ) ;
#6974=CARTESIAN_POINT ( 'NONE',  ( 24.09999999999998366, 17.56310227825320425, 98.29316153445363113 ) ) ;
#6975=DIRECTION ( 'NONE',  ( -0.000000000000000000, -0.000000000000000000, 1.000000000000000000 ) ) ;
#6976=CARTESIAN_POINT ( 'NONE',  ( 26.37500000054622973, 13.07298590277314432, 88.54243821818161564 ) ) ;
#6980=ORIENTED_EDGE ( 'NONE', *, *, #2474, .F. ) ;
#6982=CARTESIAN_POINT ( 'NONE',  ( -2.000000000000015543, 20.00000000000000355, 83.29316153445364534 ) ) ;
#6987=CARTESIAN_POINT ( 'NONE',  ( 38.87500000054622262, 20.00000000000000355, 83.50966788445364841 ) ) ;
#6988=DIRECTION ( 'NONE',  ( 0.000000000000000000, 0.000000000000000000, 1.000000000000000000 ) ) ;
#6991=CARTESIAN_POINT ( 'NONE',  ( 42.69999999999998863, 13.62011893735971135, 86.15790661882942914 ) ) ;
#6992=CARTESIAN_POINT ( 'NONE',  ( 45.39999999999999147, 27.13292387221364876, 88.47553407664153724 ) ) ;
#6995=CARTESIAN_POINT ( 'NONE',  ( 32.85000000109246088, 24.40838939219355197, 84.72553407664153724 ) ) ;
#6997=ORIENTED_EDGE ( 'NONE', *, *, #6685, .T. ) ;
#6999=CARTESIAN_POINT ( 'NONE',  ( 4.999999999999999112, 40.00000000000000000, 121.2488769092545198 ) ) ;
#7000=AXIS2_PLACEMENT_3D ( 'NONE', #9753, #44, #2832 ) ;
#7001=ORIENTED_EDGE ( 'NONE', *, *, #9929, .T. ) ;
#7002=LINE ( 'NONE', #10873, #2225 ) ;
#7005=CARTESIAN_POINT ( 'NONE',  ( -50.00000000000001421, 20.00000000000000000, 145.0000000000000000 ) ) ;
#7006=CARTESIAN_POINT ( 'NONE',  ( -50.00000000000001421, 92.00000000000000000, 69.99999999999998579 ) ) ;
#7008=CARTESIAN_POINT ( 'NONE',  ( 30.77500000054622831, 20.00000000000000355, 83.50966788445364841 ) ) ;
#7009=CARTESIAN_POINT ( 'NONE',  ( 33.57500000054622546, 26.19570976099943493, 95.29460816699764791 ) ) ;
#7012=CARTESIAN_POINT ( 'NONE',  ( 33.75000000109245946, 17.56310227825320425, 98.29316153445363113 ) ) ;
#7014=CARTESIAN_POINT ( 'NONE',  ( 48.35000000109246798, 13.62011893735971135, 86.15790661882942914 ) ) ;
#7017=ORIENTED_EDGE ( 'NONE', *, *, #8043, .F. ) ;
#7022=CARTESIAN_POINT ( 'NONE',  ( 6.629604629042566089, 27.48664723726108505, 90.27812524726596166 ) ) ;
#7024=DIRECTION ( 'NONE',  ( 0.000000000000000000, 0.000000000000000000, -1.000000000000000000 ) ) ;
#7027=CARTESIAN_POINT ( 'NONE',  ( 42.87500000054622973, 22.36655054427230382, 83.50966788445364841 ) ) ;
#7028=CARTESIAN_POINT ( 'NONE',  ( -27.49999999999999645, 27.49999999999999645, 145.0000000000000000 ) ) ;
#7032=ADVANCED_FACE ( 'NONE', ( #10951 ), #1073, .F. ) ;
#7033=CARTESIAN_POINT ( 'NONE',  ( 22.77500000054622120, 17.63344945572770328, 83.50966788445364841 ) ) ;
#7034=CARTESIAN_POINT ( 'NONE',  ( 41.77500000054621410, 22.36655054427230027, 98.07665518445361386 ) ) ;
#7035=CARTESIAN_POINT ( 'NONE',  ( 35.07500000054622546, 26.19570976099943849, 86.29171490190961435 ) ) ;
#7036=CARTESIAN_POINT ( 'NONE',  ( 20.97500000054622404, 22.36655054427230382, 83.50966788445364841 ) ) ;
#7037=CARTESIAN_POINT ( 'NONE',  ( 20.89999999999999147, 17.56310227825321135, 83.29316153445363113 ) ) ;
#7039=CARTESIAN_POINT ( 'NONE',  ( 25.97500000054622760, 15.71886984736413417, 96.68563167572563088 ) ) ;
#7044=CARTESIAN_POINT ( 'NONE',  ( -20.27158385259952667, 18.00000000000000355, 152.2284161474004520 ) ) ;
#7045=ORIENTED_EDGE ( 'NONE', *, *, #11312, .T. ) ;
#7047=CARTESIAN_POINT ( 'NONE',  ( 41.37500000054622262, 27.65831843345427998, 90.79316153445363113 ) ) ;
#7049=CARTESIAN_POINT ( 'NONE',  ( 26.19999999999998863, 15.59161060780645691, 96.86078899226572503 ) ) ;
#7050=CARTESIAN_POINT ( 'NONE',  ( 38.67500000054622689, 15.71886984736413773, 84.90069139318163138 ) ) ;
#7051=CARTESIAN_POINT ( 'NONE',  ( 44.59999999999998721, 12.86707612778636012, 88.47553407664152303 ) ) ;
#7052=EDGE_CURVE ( 'NONE', #5467, #1996, #8926, .T. ) ;
#7053=CARTESIAN_POINT ( 'NONE',  ( 48.07500000054623257, 13.80429023900056507, 95.29460816699764791 ) ) ;
#7055=CARTESIAN_POINT ( 'NONE',  ( 24.15000000109245804, 12.11403331821300533, 90.79316153445363113 ) ) ;
#7059=CARTESIAN_POINT ( 'NONE',  ( 0.000000000000000000, 0.000000000000000000, 169.9999999999999716 ) ) ;
#7062=FACE_OUTER_BOUND ( 'NONE', #6285, .T. ) ;
#7063=CARTESIAN_POINT ( 'NONE',  ( 40.99999999999998579, 20.00000000000000355, 83.29316153445364534 ) ) ;
#7064=CARTESIAN_POINT ( 'NONE',  ( 38.65000000109246514, 20.00000000000000355, 83.29316153445364534 ) ) ;
#7065=VECTOR ( 'NONE', #10209, 999.9999999999998863 ) ;
#7066=CARTESIAN_POINT ( 'NONE',  ( 27.57500000054622902, 24.28113015263587116, 96.68563167572563088 ) ) ;
#7067=CARTESIAN_POINT ( 'NONE',  ( 28.37500000054622618, 12.34168156654572535, 90.79316153445363113 ) ) ;
#7069=FACE_OUTER_BOUND ( 'NONE', #10778, .T. ) ;
#7070=DIRECTION ( 'NONE',  ( -1.000000000000000000, -0.000000000000000000, -0.000000000000000000 ) ) ;
#7075=ORIENTED_EDGE ( 'NONE', *, *, #12541, .F. ) ;
#7077=ADVANCED_FACE ( 'NONE', ( #613 ), #4478, .F. ) ;
#7083=CARTESIAN_POINT ( 'NONE',  ( 9.794823006331467852, 22.03034270180912557, 83.56881077602001540 ) ) ;
#7088=CARTESIAN_POINT ( 'NONE',  ( 42.67500000054623399, 17.63344945572770328, 83.50966788445364841 ) ) ;
#7090=EDGE_LOOP ( 'NONE', ( #3077, #7850, #1365, #6162, #10932 ) ) ;
#7093=CARTESIAN_POINT ( 'NONE',  ( 22.57500000054622546, 13.80429023900056684, 86.29171490190961435 ) ) ;
#7094=CARTESIAN_POINT ( 'NONE',  ( 41.87500000054622262, 20.00000000000000355, 98.07665518445361386 ) ) ;
#7095=CARTESIAN_POINT ( 'NONE',  ( 31.67500000054622333, 22.36655054427230027, 98.07665518445361386 ) ) ;
#7097=CARTESIAN_POINT ( 'NONE',  ( 44.75000000109246656, 22.43689772174682417, 83.29316153445364534 ) ) ;
#7099=CARTESIAN_POINT ( 'NONE',  ( 25.17500000054623044, 26.92701409722686634, 88.54243821818162985 ) ) ;
#7104=CARTESIAN_POINT ( 'NONE',  ( 33.25000000109245946, 27.13292387221364876, 93.11078899226573924 ) ) ;
#7109=ORIENTED_EDGE ( 'NONE', *, *, #7052, .T. ) ;
#7111=EDGE_CURVE ( 'NONE', #3052, #1035, #3114, .T. ) ;
#7112=AXIS2_PLACEMENT_3D ( 'NONE', #9691, #6631, #45 ) ;
#7113=CARTESIAN_POINT ( 'NONE',  ( 40.07500000054623257, 15.71886984736413417, 96.68563167572563088 ) ) ;
#7114=DIRECTION ( 'NONE',  ( 0.000000000000000000, 0.000000000000000000, 1.000000000000000000 ) ) ;
#7116=CARTESIAN_POINT ( 'NONE',  ( 38.47500000054622404, 13.07298590277314432, 88.54243821818161564 ) ) ;
#7117=CARTESIAN_POINT ( 'NONE',  ( 38.99999999999998579, 20.00000000000000355, 83.29316153445364534 ) ) ;
#7118=CARTESIAN_POINT ( 'NONE',  ( 48.77500000054622831, 20.00000000000000355, 83.50966788445364841 ) ) ;
#7119=ORIENTED_EDGE ( 'NONE', *, *, #418, .F. ) ;
#7121=CARTESIAN_POINT ( 'NONE',  ( 23.45000000109246585, 24.40838939219354842, 96.86078899226572503 ) ) ;
#7127=CARTESIAN_POINT ( 'NONE',  ( 36.15000000109245804, 12.11403331821300533, 90.79316153445363113 ) ) ;
#7129=CARTESIAN_POINT ( 'NONE',  ( 33.47500000054623115, 26.19570976099943493, 95.29460816699764791 ) ) ;
#7130=CARTESIAN_POINT ( 'NONE',  ( 33.17500000054622689, 26.19570976099943493, 86.29171490190961435 ) ) ;
#7133=CARTESIAN_POINT ( 'NONE',  ( 21.75000000109246656, 17.56310227825320425, 98.29316153445363113 ) ) ;
#7134=ORIENTED_EDGE ( 'NONE', *, *, #3099, .T. ) ;
#7135=CARTESIAN_POINT ( 'NONE',  ( 47.05000000109247082, 27.13292387221364876, 88.47553407664153724 ) ) ;
#7138=VERTEX_POINT ( 'NONE', #3835 ) ;
#7141=( BOUNDED_CURVE ( )  B_SPLINE_CURVE ( 2, ( #10697, #8739, #52, #9761, #4933, #8801, #6894, #7918, #10759, #8866, #9824 ),
 .UNSPECIFIED., .F., .F. ) 
 B_SPLINE_CURVE_WITH_KNOTS ( ( 3, 2, 2, 2, 2, 3 ),
 ( 0.3999999999999998557, 0.4066666666666665098, 0.4133333333333332194, 0.4199999999999998734, 0.4266666666666666385, 0.4333333333333332926 ),
 .UNSPECIFIED. ) 
 CURVE ( )  GEOMETRIC_REPRESENTATION_ITEM ( )  RATIONAL_B_SPLINE_CURVE ( ( 1.000000000000001332, 0.9510565162951524210, 1.000000000000000000, 0.9510565162951535312, 1.000000000000000000, 0.9510565162951535312, 1.000000000000000000, 0.9510565162951535312, 1.000000000000000000, 0.9510565162951539753, 0.9999999999999995559 ) ) 
 REPRESENTATION_ITEM ( '' )  );
#7144=EDGE_CURVE ( 'NONE', #110, #8158, #12466, .T. ) ;
#7147=DIRECTION ( 'NONE',  ( 0.000000000000000000, 0.000000000000000000, -1.000000000000000000 ) ) ;
#7148=CYLINDRICAL_SURFACE ( 'NONE', #11619, 7.500000000000000000 ) ;
#7150=APPLICATION_CONTEXT ( 'automotive_design' ) ;
#7152=VERTEX_POINT ( 'NONE', #1804 ) ;
#7155=CARTESIAN_POINT ( 'NONE',  ( 28.49999999999998579, 12.11403331821300533, 90.79316153445363113 ) ) ;
#7156=CARTESIAN_POINT ( 'NONE',  ( 43.37500000054622973, 27.65831843345427998, 90.79316153445363113 ) ) ;
#7158=CARTESIAN_POINT ( 'NONE',  ( 26.37500000054622973, 13.07298590277314432, 88.54243821818161564 ) ) ;
#7159=CARTESIAN_POINT ( 'NONE',  ( 9.621890409868294469, 17.26583415636358154, 97.78138982115301303 ) ) ;
#7161=CARTESIAN_POINT ( 'NONE',  ( 34.99999999999999289, 20.00000000000000355, 170.0000119999999697 ) ) ;
#7162=DIRECTION ( 'NONE',  ( 1.000000000000000000, 0.000000000000000000, 0.000000000000000000 ) ) ;
#7163=CARTESIAN_POINT ( 'NONE',  ( 23.97500000054623115, 15.71886984736413417, 96.68563167572563088 ) ) ;
#7165=CARTESIAN_POINT ( 'NONE',  ( 32.85000000109246088, 24.40838939219355197, 84.72553407664153724 ) ) ;
#7166=EDGE_LOOP ( 'NONE', ( #11657, #9689, #10439, #8241 ) ) ;
#7167=LINE ( 'NONE', #5154, #3057 ) ;
#7170=VECTOR ( 'NONE', #5109, 1000.000000000000000 ) ;
#7173=CARTESIAN_POINT ( 'NONE',  ( 34.47500000054622404, 13.07298590277314432, 88.54243821818161564 ) ) ;
#7175=CARTESIAN_POINT ( 'NONE',  ( 26.69999999999998508, 13.62011893735970958, 86.15790661882942914 ) ) ;
#7176=CARTESIAN_POINT ( 'NONE',  ( 34.57500000054621125, 13.80429023900056684, 86.29171490190961435 ) ) ;
#7177=CARTESIAN_POINT ( 'NONE',  ( 39.29999999999999005, 26.37988106264029398, 86.15790661882942914 ) ) ;
#7178=CARTESIAN_POINT ( 'NONE',  ( 42.77500000054622831, 20.00000000000000355, 83.50966788445364841 ) ) ;
#7181=CARTESIAN_POINT ( 'NONE',  ( 26.95000000109246585, 26.37988106264029398, 86.15790661882942914 ) ) ;
#7183=ORIENTED_EDGE ( 'NONE', *, *, #1269, .F. ) ;
#7185=ORIENTED_EDGE ( 'NONE', *, *, #6000, .T. ) ;
#7186=CARTESIAN_POINT ( 'NONE',  ( 25.35000000109246443, 26.37988106264029398, 95.42841645007781892 ) ) ;
#7190=EDGE_CURVE ( 'NONE', #4057, #3460, #2760, .T. ) ;
#7191=CARTESIAN_POINT ( 'NONE',  ( 30.97500000054622760, 24.28113015263587471, 84.90069139318163138 ) ) ;
#7192=CARTESIAN_POINT ( 'NONE',  ( 24.67500000054622689, 15.71886984736413773, 84.90069139318163138 ) ) ;
#7193=DIRECTION ( 'NONE',  ( 0.000000000000000000, -1.000000000000000000, 0.000000000000000000 ) ) ;
#7195=ORIENTED_EDGE ( 'NONE', *, *, #8392, .T. ) ;
#7197=CARTESIAN_POINT ( 'NONE',  ( 47.15000000109245804, 27.88596668178699645, 90.79316153445363113 ) ) ;
#7198=ORIENTED_EDGE ( 'NONE', *, *, #4084, .T. ) ;
#7199=CARTESIAN_POINT ( 'NONE',  ( 47.39999999999999147, 27.13292387221364876, 88.47553407664153724 ) ) ;
#7204=EDGE_CURVE ( 'NONE', #5738, #5882, #8596, .T. ) ;
#7216=( BOUNDED_CURVE ( )  B_SPLINE_CURVE ( 3, ( #2681, #4522, #7377, #2553 ),
 .UNSPECIFIED., .F., .F. ) 
 B_SPLINE_CURVE_WITH_KNOTS ( ( 4, 4 ),
 ( 0.2699327958334041266, 1.570796326794896558 ),
 .UNSPECIFIED. ) 
 CURVE ( )  GEOMETRIC_REPRESENTATION_ITEM ( )  RATIONAL_B_SPLINE_CURVE ( ( 1.000000000000000000, 0.8638816171694810864, 0.8638816171694810864, 1.000000000000000000 ) ) 
 REPRESENTATION_ITEM ( '' )  );
#7218=EDGE_CURVE ( 'NONE', #7888, #11196, #8720, .T. ) ;
#7221=CARTESIAN_POINT ( 'NONE',  ( 28.59999999999998721, 12.86707612778636012, 88.47553407664152303 ) ) ;
#7222=CARTESIAN_POINT ( 'NONE',  ( 42.47500000054623115, 13.07298590277314432, 88.54243821818161564 ) ) ;
#7224=CARTESIAN_POINT ( 'NONE',  ( 27.07500000054622902, 26.19570976099943849, 86.29171490190961435 ) ) ;
#7226=CARTESIAN_POINT ( 'NONE',  ( 10.00000000000000355, 20.00000000000000355, 83.29316153445363113 ) ) ;
#7227=PLANE ( 'NONE',  #5545 ) ;
#7229=CARTESIAN_POINT ( 'NONE',  ( -28.50000000000001066, 69.50000000000000000, 146.8533255156881978 ) ) ;
#7230=ORIENTED_EDGE ( 'NONE', *, *, #11727, .T. ) ;
#7237=CARTESIAN_POINT ( 'NONE',  ( 33.17500000054621978, 26.19570976099943849, 86.29171490190961435 ) ) ;
#7238=CARTESIAN_POINT ( 'NONE',  ( -28.50000000000001066, 84.49999999999998579, 146.8533255156881978 ) ) ;
#7239=CARTESIAN_POINT ( 'NONE',  ( 45.17500000054622689, 26.92701409722686634, 88.54243821818162985 ) ) ;
#7240=CARTESIAN_POINT ( 'NONE',  ( 31.07500000054622546, 24.28113015263587471, 84.90069139318163138 ) ) ;
#7241=CARTESIAN_POINT ( 'NONE',  ( 35.99999999999999289, 20.00000000000000355, 98.29316153445363113 ) ) ;
#7243=CARTESIAN_POINT ( 'NONE',  ( 43.57500000054623257, 24.28113015263587116, 96.68563167572563088 ) ) ;
#7244=VERTEX_POINT ( 'NONE', #7522 ) ;
#7245=CARTESIAN_POINT ( 'NONE',  ( 24.95000000109246585, 26.37988106264029398, 86.15790661882942914 ) ) ;
#7249=ORIENTED_EDGE ( 'NONE', *, *, #9929, .F. ) ;
#7252=CARTESIAN_POINT ( 'NONE',  ( 39.99999999999998579, 20.00000000000000355, 98.29316153445363113 ) ) ;
#7253=CARTESIAN_POINT ( 'NONE',  ( 25.19999999999998508, 24.40838939219355197, 84.72553407664153724 ) ) ;
#7254=CARTESIAN_POINT ( 'NONE',  ( 25.67500000054623044, 22.36655054427230027, 98.07665518445361386 ) ) ;
#7255=CARTESIAN_POINT ( 'NONE',  ( 26.47500000054622404, 13.07298590277314432, 88.54243821818161564 ) ) ;
#7259=VERTEX_POINT ( 'NONE', #7006 ) ;
#7260=CARTESIAN_POINT ( 'NONE',  ( 46.35000000109247509, 13.62011893735971135, 86.15790661882942914 ) ) ;
#7264=ORIENTED_EDGE ( 'NONE', *, *, #5433, .T. ) ;
#7268=VECTOR ( 'NONE', #675, 1000.000000000000000 ) ;
#7269=CARTESIAN_POINT ( 'NONE',  ( 20.67500000054622333, 17.63344945572770328, 83.50966788445364841 ) ) ;
#7273=CARTESIAN_POINT ( 'NONE',  ( 32.99999999999998579, 20.00000000000000355, 83.29316153445364534 ) ) ;
#7274=CARTESIAN_POINT ( 'NONE',  ( 42.59999999999998721, 12.86707612778636012, 88.47553407664152303 ) ) ;
#7275=CARTESIAN_POINT ( 'NONE',  ( -111.8465843842649292, 77.00000000000000000, 146.8533255156881978 ) ) ;
#7276=CARTESIAN_POINT ( 'NONE',  ( -6.999999999999999112, 55.00000000000000000, 124.8533255156881694 ) ) ;
#7280=VECTOR ( 'NONE', #9989, 1000.000000000000000 ) ;
#7283=ADVANCED_FACE ( 'NONE', ( #8909 ), #228, .F. ) ;
#7285=CARTESIAN_POINT ( 'NONE',  ( 43.97500000054622404, 17.63344945572769973, 98.07665518445361386 ) ) ;
#7286=CARTESIAN_POINT ( 'NONE',  ( 28.87500000054622262, 22.36655054427230382, 83.50966788445364841 ) ) ;
#7288=LINE ( 'NONE', #11158, #5628 ) ;
#7289=CARTESIAN_POINT ( 'NONE',  ( 33.29999999999999005, 26.37988106264029398, 86.15790661882942914 ) ) ;
#7290=FACE_OUTER_BOUND ( 'NONE', #7845, .T. ) ;
#7292=CARTESIAN_POINT ( 'NONE',  ( 23.45000000109246585, 24.40838939219354842, 96.86078899226572503 ) ) ;
#7295=CARTESIAN_POINT ( 'NONE',  ( 38.99999999999998579, 20.00000000000000355, 83.29316153445364534 ) ) ;
#7296=ORIENTED_EDGE ( 'NONE', *, *, #7312, .T. ) ;
#7297=CARTESIAN_POINT ( 'NONE',  ( 32.77500000054622831, 17.63344945572770328, 83.50966788445364841 ) ) ;
#7299=CARTESIAN_POINT ( 'NONE',  ( 43.77500000054622831, 20.00000000000000355, 98.07665518445361386 ) ) ;
#7300=CARTESIAN_POINT ( 'NONE',  ( 32.07500000054622546, 15.71886984736413417, 96.68563167572563088 ) ) ;
#7301=CARTESIAN_POINT ( 'NONE',  ( 34.69999999999998863, 13.62011893735971135, 86.15790661882942914 ) ) ;
#7304=CARTESIAN_POINT ( 'NONE',  ( 23.10660171779821681, 12.50000000000000711, 140.6066017177981848 ) ) ;
#7305=CARTESIAN_POINT ( 'NONE',  ( 47.37500000054622973, 26.92701409722686634, 93.04388485072563242 ) ) ;
#7307=CARTESIAN_POINT ( 'NONE',  ( 22.45000000109246585, 15.59161060780646046, 84.72553407664153724 ) ) ;
#7309=ORIENTED_EDGE ( 'NONE', *, *, #10691, .T. ) ;
#7312=EDGE_CURVE ( 'NONE', #10865, #136, #3008, .T. ) ;
#7314=VECTOR ( 'NONE', #4127, 1000.000000000000000 ) ;
#7315=CYLINDRICAL_SURFACE ( 'NONE', #8905, 7.500000000000000000 ) ;
#7316=DIRECTION ( 'NONE',  ( 0.000000000000000000, 0.000000000000000000, -1.000000000000000000 ) ) ;
#7318=CARTESIAN_POINT ( 'NONE',  ( 22.87500000054623328, 22.36655054427230382, 83.50966788445364841 ) ) ;
#7319=CARTESIAN_POINT ( 'NONE',  ( 23.17500000054622689, 26.19570976099943493, 86.29171490190961435 ) ) ;
#7323=CARTESIAN_POINT ( 'NONE',  ( 41.85000000109246798, 15.59161060780645691, 96.86078899226572503 ) ) ;
#7325=VERTEX_POINT ( 'NONE', #9868 ) ;
#7326=CARTESIAN_POINT ( 'NONE',  ( 4.999999999999999112, 0.000000000000000000, 121.2488769092545198 ) ) ;
#7330=CARTESIAN_POINT ( 'NONE',  ( 20.77500000054622831, 20.00000000000000355, 83.50966788445364841 ) ) ;
#7334=FACE_OUTER_BOUND ( 'NONE', #4805, .T. ) ;
#7335=( BOUNDED_CURVE ( )  B_SPLINE_CURVE ( 3, ( #241, #2203, #5061, #9165 ),
 .UNSPECIFIED., .F., .F. ) 
 B_SPLINE_CURVE_WITH_KNOTS ( ( 4, 4 ),
 ( 1.570796326794896558, 2.871659857756389211 ),
 .UNSPECIFIED. ) 
 CURVE ( )  GEOMETRIC_REPRESENTATION_ITEM ( )  RATIONAL_B_SPLINE_CURVE ( ( 1.000000000000000000, 0.8638816171694809753, 0.8638816171694809753, 1.000000000000000000 ) ) 
 REPRESENTATION_ITEM ( '' )  );
#7337=FACE_OUTER_BOUND ( 'NONE', #1982, .T. ) ;
#7339=CARTESIAN_POINT ( 'NONE',  ( 23.49999999999998579, 27.88596668178699645, 90.79316153445363113 ) ) ;
#7340=ORIENTED_EDGE ( 'NONE', *, *, #3179, .F. ) ;
#7343=CARTESIAN_POINT ( 'NONE',  ( 28.09999999999999076, 17.56310227825320425, 98.29316153445363113 ) ) ;
#7344=CARTESIAN_POINT ( 'NONE',  ( 40.47500000054622404, 13.07298590277314432, 88.54243821818161564 ) ) ;
#7345=CARTESIAN_POINT ( 'NONE',  ( 29.77500000054622831, 20.00000000000000355, 98.07665518445361386 ) ) ;
#7347=CARTESIAN_POINT ( 'NONE',  ( 6.909847264846026071, 12.77053099975849548, 92.80456193764219108 ) ) ;
#7350=CARTESIAN_POINT ( 'NONE',  ( 35.19999999999998863, 24.40838939219355197, 84.72553407664153724 ) ) ;
#7351=CARTESIAN_POINT ( 'NONE',  ( 31.29999999999998650, 26.37988106264029398, 86.15790661882942914 ) ) ;
#7355=ORIENTED_EDGE ( 'NONE', *, *, #10906, .F. ) ;
#7359=EDGE_CURVE ( 'NONE', #2741, #5525, #1240, .T. ) ;
#7360=CARTESIAN_POINT ( 'NONE',  ( 30.37500000054622618, 12.34168156654572357, 90.79316153445363113 ) ) ;
#7362=CARTESIAN_POINT ( 'NONE',  ( 43.07500000054622546, 26.19570976099943849, 86.29171490190961435 ) ) ;
#7363=CARTESIAN_POINT ( 'NONE',  ( 35.27500000054622120, 26.92701409722686634, 88.54243821818162985 ) ) ;
#7364=CARTESIAN_POINT ( 'NONE',  ( 32.99999999999998579, 20.00000000000000355, 83.29316153445364534 ) ) ;
#7365=CARTESIAN_POINT ( 'NONE',  ( 27.50000000000000355, 12.50000000000001066, 145.0000000000000000 ) ) ;
#7366=CARTESIAN_POINT ( 'NONE',  ( 40.97500000054622404, 24.28113015263587471, 84.90069139318163138 ) ) ;
#7367=EDGE_LOOP ( 'NONE', ( #4734, #2115, #5165, #8410, #6857 ) ) ;
#7369=CARTESIAN_POINT ( 'NONE',  ( 48.07500000054623257, 13.80429023900056507, 95.29460816699764791 ) ) ;
#7371=EDGE_LOOP ( 'NONE', ( #11887, #3794, #1132, #11904 ) ) ;
#7376=EDGE_CURVE ( 'NONE', #9352, #12263, #5996, .T. ) ;
#7377=CARTESIAN_POINT ( 'NONE',  ( -23.99529484836403981, 12.50000000000001243, 148.5047051516359602 ) ) ;
#7378=CARTESIAN_POINT ( 'NONE',  ( 32.15000000109246514, 12.11403331821300533, 90.79316153445363113 ) ) ;
#7379=CARTESIAN_POINT ( 'NONE',  ( 27.27500000054622475, 27.65831843345427998, 90.79316153445363113 ) ) ;
#7380=CARTESIAN_POINT ( 'NONE',  ( 21.97500000054622049, 17.63344945572769973, 98.07665518445361386 ) ) ;
#7382=DIRECTION ( 'NONE',  ( 0.000000000000000000, 0.000000000000000000, 1.000000000000000000 ) ) ;
#7383=EDGE_CURVE ( 'NONE', #10526, #10, #9741, .T. ) ;
#7384=CARTESIAN_POINT ( 'NONE',  ( 39.25000000109246656, 27.13292387221364876, 93.11078899226573924 ) ) ;
#7385=ORIENTED_EDGE ( 'NONE', *, *, #11576, .F. ) ;
#7386=CARTESIAN_POINT ( 'NONE',  ( 41.35000000109245377, 26.37988106264029398, 95.42841645007781892 ) ) ;
#7394=CARTESIAN_POINT ( 'NONE',  ( 29.39999999999998792, 27.13292387221364876, 88.47553407664153724 ) ) ;
#7400=DIRECTION ( 'NONE',  ( 0.000000000000000000, 0.000000000000000000, -1.000000000000000000 ) ) ;
#7401=CARTESIAN_POINT ( 'NONE',  ( 26.57500000054622902, 15.71886984736413773, 84.90069139318163138 ) ) ;
#7402=CARTESIAN_POINT ( 'NONE',  ( 26.99999999999998934, 20.00000000000000355, 83.29316153445364534 ) ) ;
#7404=ORIENTED_EDGE ( 'NONE', *, *, #2428, .F. ) ;
#7406=FACE_OUTER_BOUND ( 'NONE', #9610, .T. ) ;
#7407=VECTOR ( 'NONE', #2200, 1000.000000000000000 ) ;
#7408=SHAPE_REPRESENTATION ( 'Cast Iron Bearing Support Block', ( #9021 ), #309 ) ;
#7410=CARTESIAN_POINT ( 'NONE',  ( 36.37500000054622973, 13.07298590277314432, 88.54243821818161564 ) ) ;
#7411=CARTESIAN_POINT ( 'NONE',  ( 37.37500000054622262, 27.65831843345427998, 90.79316153445363113 ) ) ;
#7412=CARTESIAN_POINT ( 'NONE',  ( 28.97500000054622760, 24.28113015263587471, 84.90069139318163138 ) ) ;
#7413=CARTESIAN_POINT ( 'NONE',  ( 6.909788229321696562, 12.77047530449378776, 88.78197206557399568 ) ) ;
#7415=AXIS2_PLACEMENT_3D ( 'NONE', #4199, #11940, #10924 ) ;
#7416=CYLINDRICAL_SURFACE ( 'NONE', #3521, 7.499999999999992895 ) ;
#7418=VERTEX_POINT ( 'NONE', #7064 ) ;
#7420=ORIENTED_EDGE ( 'NONE', *, *, #456, .T. ) ;
#7422=EDGE_CURVE ( 'NONE', #11877, #110, #734, .T. ) ;
#7425=CARTESIAN_POINT ( 'NONE',  ( 32.17500000054622689, 13.80429023900056507, 95.29460816699764791 ) ) ;
#7427=CARTESIAN_POINT ( 'NONE',  ( 46.77500000054622831, 20.00000000000000355, 83.50966788445364841 ) ) ;
#7428=CARTESIAN_POINT ( 'NONE',  ( 35.97500000054620983, 17.63344945572769973, 98.07665518445361386 ) ) ;
#7429=CARTESIAN_POINT ( 'NONE',  ( 27.49999999999998934, 27.88596668178699645, 90.79316153445363113 ) ) ;
#7430=CARTESIAN_POINT ( 'NONE',  ( 20.00000000000001066, 15.60660171779821681, 137.4999999999999716 ) ) ;
#7431=CARTESIAN_POINT ( 'NONE',  ( 37.57500000054622546, 24.28113015263587116, 96.68563167572563088 ) ) ;
#7432=EDGE_LOOP ( 'NONE', ( #11936, #3825 ) ) ;
#7433=CARTESIAN_POINT ( 'NONE',  ( 21.65000000109246514, 20.00000000000000355, 98.29316153445363113 ) ) ;
#7442=CARTESIAN_POINT ( 'NONE',  ( -34.72841614740048044, 22.00000000000000000, 170.0000119999999697 ) ) ;
#7445=CARTESIAN_POINT ( 'NONE',  ( 22.47500000054623115, 13.80429023900056684, 86.29171490190961435 ) ) ;
#7446=CARTESIAN_POINT ( 'NONE',  ( 23.07500000054622546, 24.28113015263587471, 84.90069139318163138 ) ) ;
#7449=ORIENTED_EDGE ( 'NONE', *, *, #4123, .T. ) ;
#7450=CARTESIAN_POINT ( 'NONE',  ( 35.65000000109246514, 20.00000000000000355, 98.29316153445363113 ) ) ;
#7453=CARTESIAN_POINT ( 'NONE',  ( 29.95000000109246230, 13.62011893735970958, 95.42841645007781892 ) ) ;
#7454=EDGE_LOOP ( 'NONE', ( #1720, #1984, #8524, #11760 ) ) ;
#7455=CARTESIAN_POINT ( 'NONE',  ( 47.99999999999998579, 20.00000000000000355, 98.29316153445363113 ) ) ;
#7458=CARTESIAN_POINT ( 'NONE',  ( 29.59999999999998721, 27.13292387221364876, 93.11078899226573924 ) ) ;
#7459=AXIS2_PLACEMENT_3D ( 'NONE', #6819, #2057, #4027 ) ;
#7461=CARTESIAN_POINT ( 'NONE',  ( 27.99999999999998579, 20.00000000000000355, 98.29316153445363113 ) ) ;
#7463=EDGE_CURVE ( 'NONE', #10754, #8571, #7896, .T. ) ;
#7464=DIRECTION ( 'NONE',  ( 0.000000000000000000, 0.000000000000000000, -1.000000000000000000 ) ) ;
#7465=CARTESIAN_POINT ( 'NONE',  ( 47.77500000054622120, 22.36655054427230027, 98.07665518445361386 ) ) ;
#7466=LINE ( 'NONE', #1452, #12277 ) ;
#7469=VECTOR ( 'NONE', #2656, 1000.000000000000000 ) ;
#7470=EDGE_CURVE ( 'NONE', #5467, #5847, #10177, .T. ) ;
#7471=CARTESIAN_POINT ( 'NONE',  ( 4.999999999999999112, 18.00000000000000355, 169.9999999999999716 ) ) ;
#7473=CARTESIAN_POINT ( 'NONE',  ( 39.57500000054622546, 24.28113015263587116, 96.68563167572563088 ) ) ;
#7474=CARTESIAN_POINT ( 'NONE',  ( 35.37500000054622973, 27.65831843345427998, 90.79316153445363113 ) ) ;
#7476=VECTOR ( 'NONE', #8598, 1000.000000000000000 ) ;
#7477=DIRECTION ( 'NONE',  ( 1.000000000000000000, 0.000000000000000000, 0.000000000000000000 ) ) ;
#7479=FACE_OUTER_BOUND ( 'NONE', #9778, .T. ) ;
#7480=CARTESIAN_POINT ( 'NONE',  ( -21.00000000000001776, 81.39339828220178674, 154.3533255156881694 ) ) ;
#7483=ADVANCED_BREP_SHAPE_REPRESENTATION ( '', ( #6058, #9021 ), #309 ) ;
#7484=EDGE_CURVE ( 'NONE', #9352, #6763, #9820, .T. ) ;
#7487=CARTESIAN_POINT ( 'NONE',  ( 25.47500000054622404, 26.92701409722686634, 93.04388485072563242 ) ) ;
#7488=CARTESIAN_POINT ( 'NONE',  ( 34.72841614740048044, 22.00000000000000000, 170.0000119999999697 ) ) ;
#7489=CARTESIAN_POINT ( 'NONE',  ( 46.57500000054622546, 15.71886984736413773, 84.90069139318163138 ) ) ;
#7490=CARTESIAN_POINT ( 'NONE',  ( 29.37500000054622618, 27.65831843345427998, 90.79316153445363113 ) ) ;
#7491=CARTESIAN_POINT ( 'NONE',  ( 27.19999999999998863, 24.40838939219355197, 84.72553407664153724 ) ) ;
#7494=CARTESIAN_POINT ( 'NONE',  ( 41.27500000054622831, 27.65831843345427998, 90.79316153445363113 ) ) ;
#7497=CARTESIAN_POINT ( 'NONE',  ( 49.67500000054621978, 22.36655054427230027, 98.07665518445361386 ) ) ;
#7501=ORIENTED_EDGE ( 'NONE', *, *, #1120, .T. ) ;
#7506=CARTESIAN_POINT ( 'NONE',  ( 30.99999999999998934, 20.00000000000000355, 83.29316153445364534 ) ) ;
#7507=CARTESIAN_POINT ( 'NONE',  ( 26.87500000054622618, 22.36655054427230382, 83.50966788445364841 ) ) ;
#7508=CARTESIAN_POINT ( 'NONE',  ( 49.59999999999999432, 27.13292387221364876, 93.11078899226573924 ) ) ;
#7510=CARTESIAN_POINT ( 'NONE',  ( 40.99999999999998579, 20.00000000000000355, 83.29316153445364534 ) ) ;
#7513=CARTESIAN_POINT ( 'NONE',  ( 37.55000000109247082, 22.43689772174679575, 98.29316153445363113 ) ) ;
#7515=ORIENTED_EDGE ( 'NONE', *, *, #8294, .T. ) ;
#7522=CARTESIAN_POINT ( 'NONE',  ( -6.999999999999999112, 69.50000000000000000, 101.8533255156881978 ) ) ;
#7523=ADVANCED_FACE ( 'NONE', ( #11126 ), #2433, .F. ) ;
#7529=CARTESIAN_POINT ( 'NONE',  ( 20.27500000054623186, 12.34168156654572535, 90.79316153445363113 ) ) ;
#7530=CARTESIAN_POINT ( 'NONE',  ( 46.35000000109246798, 13.62011893735970958, 86.15790661882942914 ) ) ;
#7531=CARTESIAN_POINT ( 'NONE',  ( 47.45000000109246230, 24.40838939219354842, 96.86078899226572503 ) ) ;
#7537=CARTESIAN_POINT ( 'NONE',  ( 37.77500000054622120, 22.36655054427230027, 98.07665518445361386 ) ) ;
#7538=CARTESIAN_POINT ( 'NONE',  ( 20.57500000054622902, 15.71886984736413773, 84.90069139318163138 ) ) ;
#7543=DIRECTION ( 'NONE',  ( 1.000000000000000000, -0.000000000000000000, -0.000000000000000000 ) ) ;
#7549=( BOUNDED_CURVE ( )  B_SPLINE_CURVE ( 2, ( #8700, #6915, #11, #5972, #4896, #10719, #8757, #2032, #1160, #5024, #11165 ),
 .UNSPECIFIED., .F., .F. ) 
 B_SPLINE_CURVE_WITH_KNOTS ( ( 3, 2, 2, 2, 2, 3 ),
 ( 0.000000000000000000, 0.006666666666666673166, 0.01333333333333334633, 0.02000000000000001429, 0.02666666666666669266, 0.03333333333333336063 ),
 .UNSPECIFIED. ) 
 CURVE ( )  GEOMETRIC_REPRESENTATION_ITEM ( )  RATIONAL_B_SPLINE_CURVE ( ( 1.000000000000000000, 0.9510565162951535312, 1.000000000000000000, 0.9510565162951535312, 1.000000000000000000, 0.9510565162951535312, 1.000000000000000000, 0.9510565162951535312, 1.000000000000000000, 0.9510565162951533091, 1.000000000000000222 ) ) 
 REPRESENTATION_ITEM ( '' )  );
#7550=CARTESIAN_POINT ( 'NONE',  ( 26.57500000054622191, 13.80429023900056684, 86.29171490190961435 ) ) ;
#7551=CARTESIAN_POINT ( 'NONE',  ( 29.15000000109246159, 27.88596668178699645, 90.79316153445363113 ) ) ;
#7553=CARTESIAN_POINT ( 'NONE',  ( 39.67500000054623399, 22.36655054427230027, 98.07665518445361386 ) ) ;
#7554=CARTESIAN_POINT ( 'NONE',  ( 25.77500000054622831, 22.36655054427230027, 98.07665518445361386 ) ) ;
#7555=CARTESIAN_POINT ( 'NONE',  ( 31.99999999999998579, 20.00000000000000355, 98.29316153445363113 ) ) ;
#7557=CARTESIAN_POINT ( 'NONE',  ( 36.77500000054622831, 20.00000000000000355, 83.50966788445364841 ) ) ;
#7559=CARTESIAN_POINT ( 'NONE',  ( 46.97500000054623115, 24.28113015263587471, 84.90069139318163138 ) ) ;
#7560=CARTESIAN_POINT ( 'NONE',  ( 28.55000000109246372, 17.56310227825320425, 83.29316153445363113 ) ) ;
#7564=VERTEX_POINT ( 'NONE', #6183 ) ;
#7567=DIRECTION ( 'NONE',  ( 0.000000000000000000, 0.000000000000000000, -1.000000000000000000 ) ) ;
#7568=CARTESIAN_POINT ( 'NONE',  ( 44.27500000054622120, 13.07298590277314254, 93.04388485072563242 ) ) ;
#7570=CARTESIAN_POINT ( 'NONE',  ( 43.27500000054622120, 26.92701409722686634, 88.54243821818162985 ) ) ;
#7571=CARTESIAN_POINT ( 'NONE',  ( 49.09999999999999432, 22.43689772174679575, 83.29316153445363113 ) ) ;
#7573=CARTESIAN_POINT ( 'NONE',  ( 41.49999999999997158, 27.88596668178699645, 90.79316153445363113 ) ) ;
#7574=FACE_OUTER_BOUND ( 'NONE', #7432, .T. ) ;
#7577=CARTESIAN_POINT ( 'NONE',  ( 40.25000000109246656, 12.86707612778636012, 88.47553407664152303 ) ) ;
#7581=ORIENTED_EDGE ( 'NONE', *, *, #854, .F. ) ;
#7583=VECTOR ( 'NONE', #1849, 1000.000000000000000 ) ;
#7584=CARTESIAN_POINT ( 'NONE',  ( 30.75000000109246301, 22.43689772174679575, 83.29316153445363113 ) ) ;
#7589=CARTESIAN_POINT ( 'NONE',  ( 27.59999999999999076, 27.13292387221364876, 93.11078899226573924 ) ) ;
#7592=CARTESIAN_POINT ( 'NONE',  ( -50.00000000000001421, 55.00000000000000000, 124.8533255156881694 ) ) ;
#7593=CARTESIAN_POINT ( 'NONE',  ( 20.07500000054622546, 13.80429023900056507, 95.29460816699764791 ) ) ;
#7594=CARTESIAN_POINT ( 'NONE',  ( 46.55000000109247793, 17.56310227825318648, 83.29316153445365956 ) ) ;
#7595=CIRCLE ( 'NONE', #4354, 7.499999999999978684 ) ;
#7596=FACE_OUTER_BOUND ( 'NONE', #6559, .T. ) ;
#7602=EDGE_CURVE ( 'NONE', #5150, #1332, #5235, .T. ) ;
#7603=EDGE_CURVE ( 'NONE', #1411, #5847, #7704, .T. ) ;
#7607=DIRECTION ( 'NONE',  ( 1.000000000000000000, -0.000000000000000000, -0.000000000000000000 ) ) ;
#7610=CYLINDRICAL_SURFACE ( 'NONE', #6297, 7.499999999999992895 ) ;
#7614=ADVANCED_FACE ( 'NONE', ( #3689 ), #9599, .F. ) ;
#7615=LINE ( 'NONE', #1832, #8771 ) ;
#7616=CARTESIAN_POINT ( 'NONE',  ( 41.77500000054622831, 20.00000000000000355, 98.07665518445361386 ) ) ;
#7617=CARTESIAN_POINT ( 'NONE',  ( 28.37500000054622618, 12.34168156654572535, 90.79316153445363113 ) ) ;
#7618=CARTESIAN_POINT ( 'NONE',  ( 26.89999999999998792, 17.56310227825321135, 83.29316153445363113 ) ) ;
#7619=CARTESIAN_POINT ( 'NONE',  ( -50.00000000000001421, 20.00000000000000000, 137.5000000000000000 ) ) ;
#7620=CARTESIAN_POINT ( 'NONE',  ( 37.07500000054622546, 26.19570976099943493, 86.29171490190961435 ) ) ;
#7621=ORIENTED_EDGE ( 'NONE', *, *, #5224, .T. ) ;
#7623=CARTESIAN_POINT ( 'NONE',  ( 46.57500000054622546, 15.71886984736413773, 84.90069139318163138 ) ) ;
#7626=LINE ( 'NONE', #6724, #10156 ) ;
#7627=ORIENTED_EDGE ( 'NONE', *, *, #6675, .T. ) ;
#7629=( BOUNDED_CURVE ( )  B_SPLINE_CURVE ( 3, ( #9502, #7657, #1875, #11521 ),
 .UNSPECIFIED., .F., .F. ) 
 B_SPLINE_CURVE_WITH_KNOTS ( ( 4, 4 ),
 ( 4.712388980384689674, 6.013252511346182771 ),
 .UNSPECIFIED. ) 
 CURVE ( )  GEOMETRIC_REPRESENTATION_ITEM ( )  RATIONAL_B_SPLINE_CURVE ( ( 1.000000000000000000, 0.8638816171694809753, 0.8638816171694809753, 1.000000000000000000 ) ) 
 REPRESENTATION_ITEM ( '' )  );
#7630=CARTESIAN_POINT ( 'NONE',  ( 41.75000000109246656, 17.56310227825320425, 98.29316153445363113 ) ) ;
#7631=DIRECTION ( 'NONE',  ( 0.000000000000000000, 0.000000000000000000, -1.000000000000000000 ) ) ;
#7633=CARTESIAN_POINT ( 'NONE',  ( 41.77500000054621410, 22.36655054427230027, 98.07665518445361386 ) ) ;
#7634=PLANE ( 'NONE',  #11046 ) ;
#7635=CARTESIAN_POINT ( 'NONE',  ( 47.39999999999999147, 27.13292387221364876, 88.47553407664153724 ) ) ;
#7638=CARTESIAN_POINT ( 'NONE',  ( 38.65000000109246514, 20.00000000000000355, 83.29316153445364534 ) ) ;
#7640=CARTESIAN_POINT ( 'NONE',  ( 37.05000000109246372, 27.13292387221364876, 88.47553407664153724 ) ) ;
#7641=CARTESIAN_POINT ( 'NONE',  ( 24.39999999999998792, 12.86707612778636012, 93.11078899226572503 ) ) ;
#7645=DIRECTION ( 'NONE',  ( 0.000000000000000000, 0.000000000000000000, -1.000000000000000000 ) ) ;
#7652=CARTESIAN_POINT ( 'NONE',  ( 0.000000000000000000, 20.00000000000000355, 109.9999999999999858 ) ) ;
#7653=CARTESIAN_POINT ( 'NONE',  ( 20.47500000054622760, 13.80429023900056684, 86.29171490190961435 ) ) ;
#7657=CARTESIAN_POINT ( 'NONE',  ( -23.99529484836403270, 27.49999999999999645, 148.5047051516359318 ) ) ;
#7658=CYLINDRICAL_SURFACE ( 'NONE', #234, 7.500000000000000000 ) ;
#7659=ORIENTED_EDGE ( 'NONE', *, *, #8095, .F. ) ;
#7660=ORIENTED_EDGE ( 'NONE', *, *, #10849, .F. ) ;
#7664=CARTESIAN_POINT ( 'NONE',  ( 22.57500000054622902, 15.71886984736413773, 84.90069139318163138 ) ) ;
#7668=DIRECTION ( 'NONE',  ( -0.000000000000000000, -1.000000000000000000, -0.000000000000000000 ) ) ;
#7670=CARTESIAN_POINT ( 'NONE',  ( 19.99999999999999645, 20.00000000000000355, 170.0000119999999697 ) ) ;
#7671=ORIENTED_EDGE ( 'NONE', *, *, #189, .T. ) ;
#7676=CARTESIAN_POINT ( 'NONE',  ( 25.57500000054621836, 26.19570976099943849, 95.29460816699764791 ) ) ;
#7679=CARTESIAN_POINT ( 'NONE',  ( 40.57500000054623257, 15.71886984736413773, 84.90069139318163138 ) ) ;
#7681=CARTESIAN_POINT ( 'NONE',  ( 25.67500000054622333, 24.28113015263587116, 96.68563167572563088 ) ) ;
#7682=CARTESIAN_POINT ( 'NONE',  ( 29.69999999999998508, 26.37988106264029398, 95.42841645007781892 ) ) ;
#7683=( NAMED_UNIT ( * ) SI_UNIT ( $, .STERADIAN. ) SOLID_ANGLE_UNIT ( ) );
#7684=CARTESIAN_POINT ( 'NONE',  ( 31.77500000054622831, 20.00000000000000355, 98.07665518445361386 ) ) ;
#7686=FACE_OUTER_BOUND ( 'NONE', #1207, .T. ) ;
#7688=VECTOR ( 'NONE', #11353, 1000.000000000000000 ) ;
#7690=ORIENTED_EDGE ( 'NONE', *, *, #5232, .T. ) ;
#7691=AXIS2_PLACEMENT_3D ( 'NONE', #3320, #10939, #9866 ) ;
#7695=EDGE_CURVE ( 'NONE', #8919, #223, #2748, .T. ) ;
#7697=CARTESIAN_POINT ( 'NONE',  ( 19.87500000054622262, 20.00000000000000355, 98.07665518445361386 ) ) ;
#7699=CARTESIAN_POINT ( 'NONE',  ( 49.27500000054623541, 27.65831843345427998, 90.79316153445363113 ) ) ;
#7701=CARTESIAN_POINT ( 'NONE',  ( 33.05000000109247082, 27.13292387221364876, 88.47553407664153724 ) ) ;
#7702=CARTESIAN_POINT ( 'NONE',  ( 24.59999999999998721, 12.86707612778636012, 88.47553407664152303 ) ) ;
#7704=( BOUNDED_CURVE ( )  B_SPLINE_CURVE ( 2, ( #2494, #11248, #6370, #5422, #10236, #7378, #599, #4461, #8340, #12206, #3506 ),
 .UNSPECIFIED., .F., .F. ) 
 B_SPLINE_CURVE_WITH_KNOTS ( ( 3, 2, 2, 2, 2, 3 ),
 ( 0.5666666666666666519, 0.5733333333333333615, 0.5799999999999999600, 0.5866666666666666696, 0.5933333333333333792, 0.5999999999999999778 ),
 .UNSPECIFIED. ) 
 CURVE ( )  GEOMETRIC_REPRESENTATION_ITEM ( )  RATIONAL_B_SPLINE_CURVE ( ( 1.000000000000000000, 0.9510565162951535312, 1.000000000000000000, 0.9510565162951535312, 1.000000000000000000, 0.9510565162951535312, 1.000000000000000000, 0.9510565162951535312, 1.000000000000000000, 0.9510565162951535312, 1.000000000000000000 ) ) 
 REPRESENTATION_ITEM ( '' )  );
#7705=EDGE_CURVE ( 'NONE', #10754, #4846, #10287, .T. ) ;
#7706=VERTEX_POINT ( 'NONE', #10597 ) ;
#7711=CARTESIAN_POINT ( 'NONE',  ( 34.27500000054623541, 12.34168156654572535, 90.79316153445363113 ) ) ;
#7714=CARTESIAN_POINT ( 'NONE',  ( 27.50000000000000355, 27.49999999999999645, 145.0000000000000000 ) ) ;
#7716=AXIS2_PLACEMENT_3D ( 'NONE', #125, #11731, #11669 ) ;
#7718=CARTESIAN_POINT ( 'NONE',  ( -2.000000000000015543, 20.00000000000000355, 90.79316153445363113 ) ) ;
#7719=CARTESIAN_POINT ( 'NONE',  ( 19.77500000054622831, 20.00000000000000355, 98.07665518445361386 ) ) ;
#7721=CARTESIAN_POINT ( 'NONE',  ( 45.65000000109247225, 20.00000000000000355, 98.29316153445363113 ) ) ;
#7724=EDGE_LOOP ( 'NONE', ( #10553, #572, #1615, #4771, #3830, #1761 ) ) ;
#7733=CARTESIAN_POINT ( 'NONE',  ( -2.000000000000015543, 20.00000000000000355, 98.29316153445363113 ) ) ;
#7736=VERTEX_POINT ( 'NONE', #7506 ) ;
#7738=ADVANCED_FACE ( 'NONE', ( #841 ), #5794, .F. ) ;
#7739=CARTESIAN_POINT ( 'NONE',  ( 28.67500000054622689, 15.71886984736413773, 84.90069139318163138 ) ) ;
#7740=CARTESIAN_POINT ( 'NONE',  ( 48.17500000054622689, 13.80429023900056507, 95.29460816699764791 ) ) ;
#7741=CARTESIAN_POINT ( 'NONE',  ( 42.27500000054622120, 12.34168156654572357, 90.79316153445363113 ) ) ;
#7742=CARTESIAN_POINT ( 'NONE',  ( 26.27500000054622475, 13.07298590277314254, 93.04388485072563242 ) ) ;
#7743=CARTESIAN_POINT ( 'NONE',  ( 25.79999999999998650, 24.40838939219354842, 96.86078899226572503 ) ) ;
#7744=ADVANCED_FACE ( 'NONE', ( #11377 ), #8398, .F. ) ;
#7745=CARTESIAN_POINT ( 'NONE',  ( 35.57500000054622546, 24.28113015263587116, 96.68563167572563088 ) ) ;
#7750=VERTEX_POINT ( 'NONE', #11437 ) ;
#7751=CARTESIAN_POINT ( 'NONE',  ( 43.49999999999998579, 27.88596668178699645, 90.79316153445363113 ) ) ;
#7753=CARTESIAN_POINT ( 'NONE',  ( 43.27500000054622120, 26.92701409722686634, 88.54243821818162985 ) ) ;
#7754=CARTESIAN_POINT ( 'NONE',  ( 40.65000000109246514, 20.00000000000000355, 83.29316153445364534 ) ) ;
#7756=CARTESIAN_POINT ( 'NONE',  ( 46.17500000054622689, 13.80429023900056507, 95.29460816699764791 ) ) ;
#7757=CARTESIAN_POINT ( 'NONE',  ( 47.49999999999997868, 27.88596668178699645, 90.79316153445363113 ) ) ;
#7759=CARTESIAN_POINT ( 'NONE',  ( 40.99999999999998579, 20.00000000000000355, 83.29316153445364534 ) ) ;
#7762=CIRCLE ( 'NONE', #4308, 7.499999999999992895 ) ;
#7763=CARTESIAN_POINT ( 'NONE',  ( 33.85000000109246798, 15.59161060780645691, 96.86078899226572503 ) ) ;
#7766=EDGE_CURVE ( 'NONE', #11262, #8158, #8519, .T. ) ;
#7767=ORIENTED_EDGE ( 'NONE', *, *, #6076, .T. ) ;
#7773=CARTESIAN_POINT ( 'NONE',  ( 34.17500000054622689, 13.07298590277314254, 93.04388485072563242 ) ) ;
#7774=CARTESIAN_POINT ( 'NONE',  ( 40.57500000054621836, 13.80429023900056684, 86.29171490190961435 ) ) ;
#7776=CARTESIAN_POINT ( 'NONE',  ( 34.95000000109246940, 26.37988106264029398, 86.15790661882942914 ) ) ;
#7780=CARTESIAN_POINT ( 'NONE',  ( 48.95000000109246940, 26.37988106264029398, 86.15790661882942914 ) ) ;
#7781=ADVANCED_FACE ( 'NONE', ( #9852 ), #4136, .T. ) ;
#7782=ORIENTED_EDGE ( 'NONE', *, *, #4832, .F. ) ;
#7783=CARTESIAN_POINT ( 'NONE',  ( 35.99999999999999289, 20.00000000000000355, 98.29316153445363113 ) ) ;
#7791=CARTESIAN_POINT ( 'NONE',  ( 8.665638667393702477, 24.99499069331186973, 85.19347117998894703 ) ) ;
#7794=LINE ( 'NONE', #11666, #11819 ) ;
#7802=CARTESIAN_POINT ( 'NONE',  ( 24.07500000054622546, 15.71886984736413417, 96.68563167572563088 ) ) ;
#7803=CARTESIAN_POINT ( 'NONE',  ( 48.87500000054622262, 20.00000000000000355, 83.50966788445364841 ) ) ;
#7804=CARTESIAN_POINT ( 'NONE',  ( 38.07500000054622546, 13.80429023900056507, 95.29460816699764791 ) ) ;
#7805=CARTESIAN_POINT ( 'NONE',  ( 22.77500000054622475, 17.63344945572770328, 83.50966788445364841 ) ) ;
#7806=CARTESIAN_POINT ( 'NONE',  ( 22.79999999999998650, 15.59161060780646046, 84.72553407664153724 ) ) ;
#7807=CARTESIAN_POINT ( 'NONE',  ( 35.17500000054622689, 26.92701409722686634, 88.54243821818162985 ) ) ;
#7809=DIRECTION ( 'NONE',  ( -1.000000000000000000, 0.000000000000000000, -0.000000000000000000 ) ) ;
#7810=ORIENTED_EDGE ( 'NONE', *, *, #598, .T. ) ;
#7811=EDGE_CURVE ( 'NONE', #2249, #11209, #4960, .T. ) ;
#7815=CARTESIAN_POINT ( 'NONE',  ( 42.99999999999999289, 20.00000000000000355, 83.29316153445364534 ) ) ;
#7819=CARTESIAN_POINT ( 'NONE',  ( 38.97500000054622404, 22.36655054427230382, 83.50966788445364841 ) ) ;
#7820=CARTESIAN_POINT ( 'NONE',  ( 39.65000000109246514, 20.00000000000000355, 98.29316153445363113 ) ) ;
#7822=( BOUNDED_CURVE ( )  B_SPLINE_CURVE ( 2, ( #1047, #2874, #3063, #3822, #217, #8767, #4843, #11816, #1103, #4971, #5861 ),
 .UNSPECIFIED., .F., .F. ) 
 B_SPLINE_CURVE_WITH_KNOTS ( ( 3, 2, 2, 2, 2, 3 ),
 ( 0.3333333333333333703, 0.3400000000000000799, 0.3466666666666667340, 0.3533333333333333881, 0.3600000000000000422, 0.3666666666666666963 ),
 .UNSPECIFIED. ) 
 CURVE ( )  GEOMETRIC_REPRESENTATION_ITEM ( )  RATIONAL_B_SPLINE_CURVE ( ( 0.9999999999999995559, 0.9510565162951539753, 1.000000000000000000, 0.9510565162951535312, 1.000000000000000000, 0.9510565162951535312, 1.000000000000000000, 0.9510565162951535312, 1.000000000000000000, 0.9510565162951530871, 1.000000000000000444 ) ) 
 REPRESENTATION_ITEM ( '' )  );
#7823=CARTESIAN_POINT ( 'NONE',  ( 44.27500000054622120, 13.07298590277314254, 93.04388485072563242 ) ) ;
#7824=CARTESIAN_POINT ( 'NONE',  ( 45.09999999999999432, 22.43689772174679575, 83.29316153445363113 ) ) ;
#7827=ORIENTED_EDGE ( 'NONE', *, *, #11650, .T. ) ;
#7828=CARTESIAN_POINT ( 'NONE',  ( 32.25000000109245946, 12.86707612778636012, 88.47553407664152303 ) ) ;
#7830=ORIENTED_EDGE ( 'NONE', *, *, #5433, .F. ) ;
#7831=ORIENTED_EDGE ( 'NONE', *, *, #7705, .T. ) ;
#7832=DIRECTION ( 'NONE',  ( 1.000000000000000000, -0.000000000000000000, -0.000000000000000000 ) ) ;
#7833=ADVANCED_FACE ( 'NONE', ( #11689, #2995 ), #8827, .T. ) ;
#7835=CARTESIAN_POINT ( 'NONE',  ( 48.39999999999999147, 12.86707612778636012, 93.11078899226572503 ) ) ;
#7836=VECTOR ( 'NONE', #11154, 1000.000000000000114 ) ;
#7837=CARTESIAN_POINT ( 'NONE',  ( 38.07500000054623257, 13.80429023900056507, 95.29460816699764791 ) ) ;
#7838=CARTESIAN_POINT ( 'NONE',  ( 33.27500000054622831, 26.92701409722686634, 88.54243821818162985 ) ) ;
#7839=CARTESIAN_POINT ( 'NONE',  ( 35.35000000109246088, 26.37988106264029398, 95.42841645007781892 ) ) ;
#7841=DIRECTION ( 'NONE',  ( 1.000000000000000000, -0.000000000000000000, -0.000000000000000000 ) ) ;
#7845=EDGE_LOOP ( 'NONE', ( #9113, #8003, #8087 ) ) ;
#7849=EDGE_CURVE ( 'NONE', #6810, #4582, #5031, .T. ) ;
#7850=ORIENTED_EDGE ( 'NONE', *, *, #6451, .F. ) ;
#7852=ADVANCED_FACE ( 'NONE', ( #6862 ), #8895, .F. ) ;
#7854=CARTESIAN_POINT ( 'NONE',  ( 8.035266039410178252, 25.95549721022405976, 95.35796119567172013 ) ) ;
#7855=CARTESIAN_POINT ( 'NONE',  ( -50.00000000000001421, 84.49999999999998579, 101.8533255156881978 ) ) ;
#7858=CARTESIAN_POINT ( 'NONE',  ( -21.00000000000001776, 72.60660171779821326, 154.3533255156881694 ) ) ;
#7859=CARTESIAN_POINT ( 'NONE',  ( 45.17500000054622689, 26.92701409722686634, 88.54243821818162985 ) ) ;
#7865=CARTESIAN_POINT ( 'NONE',  ( 45.99999999999998579, 20.00000000000000355, 98.29316153445363113 ) ) ;
#7866=CARTESIAN_POINT ( 'NONE',  ( 48.37500000054621552, 12.34168156654572535, 90.79316153445363113 ) ) ;
#7867=CARTESIAN_POINT ( 'NONE',  ( 32.77500000054622831, 20.00000000000000355, 83.50966788445364841 ) ) ;
#7869=CARTESIAN_POINT ( 'NONE',  ( 22.27500000054622120, 13.07298590277314254, 93.04388485072563242 ) ) ;
#7870=CARTESIAN_POINT ( 'NONE',  ( 22.19999999999998863, 15.59161060780645691, 96.86078899226572503 ) ) ;
#7872=CARTESIAN_POINT ( 'NONE',  ( 30.97500000054622760, 24.28113015263587471, 84.90069139318163138 ) ) ;
#7878=DIRECTION ( 'NONE',  ( -0.000000000000000000, -0.000000000000000000, 1.000000000000000000 ) ) ;
#7880=CARTESIAN_POINT ( 'NONE',  ( 41.07500000054622546, 24.28113015263587471, 84.90069139318163138 ) ) ;
#7883=CARTESIAN_POINT ( 'NONE',  ( 20.25000000109246301, 12.86707612778636012, 88.47553407664152303 ) ) ;
#7884=CARTESIAN_POINT ( 'NONE',  ( 41.59999999999998721, 27.13292387221364876, 93.11078899226573924 ) ) ;
#7887=VECTOR ( 'NONE', #6975, 1000.000000000000000 ) ;
#7888=VERTEX_POINT ( 'NONE', #6921 ) ;
#7889=CARTESIAN_POINT ( 'NONE',  ( 30.25000000109246656, 12.86707612778636012, 88.47553407664152303 ) ) ;
#7894=CARTESIAN_POINT ( 'NONE',  ( -34.72841614740047333, 18.00000000000000355, 170.0000119999999697 ) ) ;
#7895=CARTESIAN_POINT ( 'NONE',  ( -5.000000000000000888, 18.00000000000000355, 218.7511230907454944 ) ) ;
#7896=LINE ( 'NONE', #11766, #1696 ) ;
#7897=CARTESIAN_POINT ( 'NONE',  ( 32.77500000054622831, 20.00000000000000355, 83.50966788445364841 ) ) ;
#7898=CARTESIAN_POINT ( 'NONE',  ( 29.47500000054622404, 26.92701409722686634, 93.04388485072563242 ) ) ;
#7904=CARTESIAN_POINT ( 'NONE',  ( 49.67500000054622689, 24.28113015263587116, 96.68563167572563088 ) ) ;
#7905=CARTESIAN_POINT ( 'NONE',  ( 48.75000000109246656, 22.43689772174679575, 83.29316153445363113 ) ) ;
#7906=EDGE_LOOP ( 'NONE', ( #10112, #10918, #12532, #5585 ) ) ;
#7910=PRODUCT_DEFINITION ( 'UNKNOWN', '', #9203, #2187 ) ;
#7913=ADVANCED_FACE ( 'NONE', ( #6797 ), #5918, .F. ) ;
#7916=FACE_OUTER_BOUND ( 'NONE', #3391, .T. ) ;
#7917=CARTESIAN_POINT ( 'NONE',  ( 9.950222915369092647, 21.02923226400954704, 98.22668337568666175 ) ) ;
#7918=CARTESIAN_POINT ( 'NONE',  ( 37.29999999999998295, 26.37988106264029398, 86.15790661882942914 ) ) ;
#7920=LINE ( 'NONE', #11786, #4319 ) ;
#7922=CARTESIAN_POINT ( 'NONE',  ( 40.47500000054622404, 13.80429023900056684, 86.29171490190961435 ) ) ;
#7923=FACE_OUTER_BOUND ( 'NONE', #3971, .T. ) ;
#7925=AXIS2_PLACEMENT_3D ( 'NONE', #5338, #454, #5401 ) ;
#7931=CARTESIAN_POINT ( 'NONE',  ( 35.47500000054623115, 26.19570976099943849, 95.29460816699764791 ) ) ;
#7932=ADVANCED_FACE ( 'NONE', ( #1043 ), #4903, .F. ) ;
#7934=CARTESIAN_POINT ( 'NONE',  ( 22.59999999999998721, 12.86707612778636012, 88.47553407664152303 ) ) ;
#7936=CARTESIAN_POINT ( 'NONE',  ( 26.07500000054622902, 13.80429023900056507, 95.29460816699764791 ) ) ;
#7942=EDGE_LOOP ( 'NONE', ( #6830, #8733, #10567, #7119 ) ) ;
#7943=( NAMED_UNIT ( * ) PLANE_ANGLE_UNIT ( ) SI_UNIT ( $, .RADIAN. ) );
#7944=FACE_OUTER_BOUND ( 'NONE', #1350, .T. ) ;
#7946=CARTESIAN_POINT ( 'NONE',  ( 35.57500000054622546, 26.19570976099943849, 95.29460816699764791 ) ) ;
#7947=DIRECTION ( 'NONE',  ( 1.000000000000000000, -0.000000000000000000, -0.000000000000000000 ) ) ;
#7949=CARTESIAN_POINT ( 'NONE',  ( 40.17500000054622689, 13.80429023900056507, 95.29460816699764791 ) ) ;
#7950=CARTESIAN_POINT ( 'NONE',  ( 43.59999999999998721, 27.13292387221364876, 93.11078899226573924 ) ) ;
#7951=CARTESIAN_POINT ( 'NONE',  ( 27.49999999999999645, 20.00000000000000355, 169.9999999999999716 ) ) ;
#7954=CARTESIAN_POINT ( 'NONE',  ( 33.25000000109245946, 27.13292387221364876, 93.11078899226573924 ) ) ;
#7958=CARTESIAN_POINT ( 'NONE',  ( 25.55000000109246372, 22.43689772174679575, 98.29316153445363113 ) ) ;
#7961=CARTESIAN_POINT ( 'NONE',  ( 33.07500000054623257, 26.19570976099943493, 86.29171490190961435 ) ) ;
#7962=CARTESIAN_POINT ( 'NONE',  ( 31.07500000054622546, 24.28113015263587471, 84.90069139318163138 ) ) ;
#7966=CARTESIAN_POINT ( 'NONE',  ( -28.50000000000001066, 77.00000000000000000, 104.8533255156881836 ) ) ;
#7967=ORIENTED_EDGE ( 'NONE', *, *, #1627, .F. ) ;
#7968=CARTESIAN_POINT ( 'NONE',  ( 49.07500000054622546, 24.28113015263587471, 84.90069139318163138 ) ) ;
#7970=DIRECTION ( 'NONE',  ( 0.000000000000000000, 0.000000000000000000, 1.000000000000000000 ) ) ;
#7972=ORIENTED_EDGE ( 'NONE', *, *, #2500, .F. ) ;
#7980=CARTESIAN_POINT ( 'NONE',  ( 6.910910677945284242, 27.22845955987902045, 92.80827258204288910 ) ) ;
#7984=CARTESIAN_POINT ( 'NONE',  ( -2.000000000000015543, 20.00000000000000355, 90.79316153445363113 ) ) ;
#7987=CARTESIAN_POINT ( 'NONE',  ( 42.27500000054622831, 12.34168156654572535, 90.79316153445363113 ) ) ;
#7990=EDGE_LOOP ( 'NONE', ( #7185, #5811, #7449, #1052 ) ) ;
#7992=EDGE_CURVE ( 'NONE', #10300, #6066, #11051, .T. ) ;
#7993=CARTESIAN_POINT ( 'NONE',  ( 22.07500000054622191, 15.71886984736413417, 96.68563167572563088 ) ) ;
#7994=CARTESIAN_POINT ( 'NONE',  ( 45.37500000054622973, 27.65831843345427998, 90.79316153445363113 ) ) ;
#7995=CARTESIAN_POINT ( 'NONE',  ( 36.37500000054622973, 13.07298590277314432, 88.54243821818161564 ) ) ;
#7996=CARTESIAN_POINT ( 'NONE',  ( 21.27500000054622475, 26.92701409722686634, 88.54243821818162985 ) ) ;
#7997=CARTESIAN_POINT ( 'NONE',  ( 25.89999999999999147, 22.43689772174679575, 98.29316153445363113 ) ) ;
#7999=CARTESIAN_POINT ( 'NONE',  ( 29.27500000054622831, 27.65831843345427998, 90.79316153445363113 ) ) ;
#8001=CARTESIAN_POINT ( 'NONE',  ( 33.45000000109246940, 24.40838939219354842, 96.86078899226572503 ) ) ;
#8002=VERTEX_POINT ( 'NONE', #7238 ) ;
#8003=ORIENTED_EDGE ( 'NONE', *, *, #8455, .T. ) ;
#8008=CARTESIAN_POINT ( 'NONE',  ( 40.37500000054620131, 12.34168156654572357, 90.79316153445363113 ) ) ;
#8011=CARTESIAN_POINT ( 'NONE',  ( 38.87500000054622262, 20.00000000000000355, 83.50966788445364841 ) ) ;
#8012=CARTESIAN_POINT ( 'NONE',  ( 44.19999999999998863, 15.59161060780645691, 96.86078899226572503 ) ) ;
#8013=VECTOR ( 'NONE', #5889, 1000.000000000000000 ) ;
#8015=CARTESIAN_POINT ( 'NONE',  ( 45.37500000054622973, 26.92701409722686634, 93.04388485072563242 ) ) ;
#8017=CARTESIAN_POINT ( 'NONE',  ( 25.35000000109246443, 26.37988106264029398, 95.42841645007781892 ) ) ;
#8019=ORIENTED_EDGE ( 'NONE', *, *, #7204, .F. ) ;
#8022=DIRECTION ( 'NONE',  ( 1.000000000000000000, -0.000000000000000000, -0.000000000000000000 ) ) ;
#8026=CARTESIAN_POINT ( 'NONE',  ( -50.00000000000001421, 18.00000000000000355, 188.4007504869563263 ) ) ;
#8028=CARTESIAN_POINT ( 'NONE',  ( 28.97500000054622760, 24.28113015263587471, 84.90069139318163138 ) ) ;
#8029=CARTESIAN_POINT ( 'NONE',  ( 28.57500000054622191, 13.80429023900056684, 86.29171490190961435 ) ) ;
#8032=CARTESIAN_POINT ( 'NONE',  ( 22.45000000109246585, 15.59161060780646046, 84.72553407664153724 ) ) ;
#8041=( BOUNDED_CURVE ( )  B_SPLINE_CURVE ( 3, ( #9604, #8900, #218, #4074 ),
 .UNSPECIFIED., .F., .F. ) 
 B_SPLINE_CURVE_WITH_KNOTS ( ( 4, 4 ),
 ( 4.712388980384689674, 6.283185307179585344 ),
 .UNSPECIFIED. ) 
 CURVE ( )  GEOMETRIC_REPRESENTATION_ITEM ( )  RATIONAL_B_SPLINE_CURVE ( ( 1.000000000000000000, 0.8047378541243649375, 0.8047378541243649375, 1.000000000000000000 ) ) 
 REPRESENTATION_ITEM ( '' )  );
#8043=EDGE_CURVE ( 'NONE', #10504, #7244, #8323, .T. ) ;
#8045=CARTESIAN_POINT ( 'NONE',  ( 6.843319662667745717, 27.29209522608180549, 92.56476529371846595 ) ) ;
#8053=CARTESIAN_POINT ( 'NONE',  ( 42.57500000054623257, 15.71886984736413773, 84.90069139318163138 ) ) ;
#8055=ORIENTED_EDGE ( 'NONE', *, *, #4865, .T. ) ;
#8058=CARTESIAN_POINT ( 'NONE',  ( 22.27500000054622120, 13.07298590277314254, 93.04388485072563242 ) ) ;
#8059=CARTESIAN_POINT ( 'NONE',  ( 47.47500000054622404, 26.92701409722686634, 93.04388485072563242 ) ) ;
#8060=CARTESIAN_POINT ( 'NONE',  ( 34.77500000054622831, 20.00000000000000355, 83.50966788445364841 ) ) ;
#8061=CARTESIAN_POINT ( 'NONE',  ( 22.67500000054622333, 15.71886984736413773, 84.90069139318163138 ) ) ;
#8064=CARTESIAN_POINT ( 'NONE',  ( 23.87500000054622973, 17.63344945572769973, 98.07665518445361386 ) ) ;
#8068=ORIENTED_EDGE ( 'NONE', *, *, #5111, .T. ) ;
#8069=AXIS2_PLACEMENT_3D ( 'NONE', #11810, #4900, #9663 ) ;
#8071=ORIENTED_EDGE ( 'NONE', *, *, #6421, .T. ) ;
#8075=CARTESIAN_POINT ( 'NONE',  ( 37.37500000054622262, 27.65831843345427998, 90.79316153445363113 ) ) ;
#8076=DIRECTION ( 'NONE',  ( -1.000000000000000000, -0.000000000000000000, -0.000000000000000000 ) ) ;
#8077=CARTESIAN_POINT ( 'NONE',  ( -27.49999999999999645, 12.50000000000001066, 145.0000000000000000 ) ) ;
#8078=CARTESIAN_POINT ( 'NONE',  ( 39.67500000054622689, 24.28113015263587116, 96.68563167572563088 ) ) ;
#8079=CARTESIAN_POINT ( 'NONE',  ( 40.49999999999999289, 12.11403331821300533, 90.79316153445363113 ) ) ;
#8080=CARTESIAN_POINT ( 'NONE',  ( 44.27500000054622120, 12.34168156654572535, 90.79316153445363113 ) ) ;
#8082=CARTESIAN_POINT ( 'NONE',  ( 22.75000000109246656, 22.43689772174679575, 83.29316153445363113 ) ) ;
#8087=ORIENTED_EDGE ( 'NONE', *, *, #9543, .T. ) ;
#8090=CARTESIAN_POINT ( 'NONE',  ( 41.05000000109246372, 27.13292387221364876, 88.47553407664153724 ) ) ;
#8092=CARTESIAN_POINT ( 'NONE',  ( 32.47500000054623825, 13.80429023900056684, 86.29171490190961435 ) ) ;
#8093=CARTESIAN_POINT ( 'NONE',  ( 34.27500000054622120, 13.07298590277314254, 93.04388485072563242 ) ) ;
#8094=CYLINDRICAL_SURFACE ( 'NONE', #10019, 7.499999999999978684 ) ;
#8095=EDGE_CURVE ( 'NONE', #8953, #3460, #5935, .T. ) ;
#8096=CLOSED_SHELL ( 'NONE', ( #3533, #6334, #7744, #615, #6832, #9561, #8922, #5518, #6293, #2886, #6947, #411, #7077, #11693, #6144, #10653, #212, #9316, #7738, #9259, #639, #372, #3953, #3556, #1649, #713, #3579, #4496, #3165, #1828, #7913, #9492, #6638, #5464, #6200, #12465, #2818, #11699, #1146, #6267, #11385, #6290, #7283, #10488, #7852, #7614, #857, #1547, #11261, #8770, #9950, #2638, #8582, #12022, #10557, #3432, #365, #1920, #8475, #7833, #12238, #756, #12419, #9960, #4963, #9185, #2607, #3472, #6765, #10253, #4108, #9454, #1252, #1898, #7523, #4649, #4245, #2255, #7781, #7932, #2738, #6531, #6739, #4441, #8537, #6903, #11882, #11343, #11291, #8377, #5117, #7032 ) ) ;
#8099=CARTESIAN_POINT ( 'NONE',  ( 40.95000000109246940, 26.37988106264029398, 86.15790661882942914 ) ) ;
#8100=ORIENTED_EDGE ( 'NONE', *, *, #561, .F. ) ;
#8108=CARTESIAN_POINT ( 'NONE',  ( 37.85000000109246798, 15.59161060780645691, 96.86078899226572503 ) ) ;
#8109=CIRCLE ( 'NONE', #6090, 7.500000000000000000 ) ;
#8111=LINE ( 'NONE', #5320, #3101 ) ;
#8115=( BOUNDED_CURVE ( )  B_SPLINE_CURVE ( 2, ( #3965, #2890, #8981, #10618, #4090, #10809, #4859, #3141, #1931, #7012, #5053 ),
 .UNSPECIFIED., .F., .F. ) 
 B_SPLINE_CURVE_WITH_KNOTS ( ( 3, 2, 2, 2, 2, 3 ),
 ( 0.5000000000000000000, 0.5066666666666667096, 0.5133333333333333082, 0.5200000000000000178, 0.5266666666666666163, 0.5333333333333333259 ),
 .UNSPECIFIED. ) 
 CURVE ( )  GEOMETRIC_REPRESENTATION_ITEM ( )  RATIONAL_B_SPLINE_CURVE ( ( 1.000000000000000000, 0.9510565162951535312, 1.000000000000000000, 0.9510565162951535312, 1.000000000000000000, 0.9510565162951535312, 1.000000000000000000, 0.9510565162951535312, 1.000000000000000000, 0.9510565162951535312, 1.000000000000000000 ) ) 
 REPRESENTATION_ITEM ( '' )  );
#8117=EDGE_CURVE ( 'NONE', #574, #1317, #10692, .T. ) ;
#8119=CARTESIAN_POINT ( 'NONE',  ( 44.17500000054622689, 13.80429023900056507, 95.29460816699764791 ) ) ;
#8120=CARTESIAN_POINT ( 'NONE',  ( 35.27500000054621410, 27.65831843345427998, 90.79316153445363113 ) ) ;
#8121=CARTESIAN_POINT ( 'NONE',  ( 8.669261784762754885, 15.00032884213714546, 96.40336117293375651 ) ) ;
#8122=CARTESIAN_POINT ( 'NONE',  ( 20.09999999999998366, 17.56310227825320425, 98.29316153445363113 ) ) ;
#8123=CARTESIAN_POINT ( 'NONE',  ( 49.89999999999998437, 22.43689772174679575, 98.29316153445363113 ) ) ;
#8124=CARTESIAN_POINT ( 'NONE',  ( 26.77500000054622831, 20.00000000000000355, 83.50966788445364841 ) ) ;
#8127=PRODUCT ( 'Cast Iron Bearing Support Block', 'Cast Iron Bearing Support Block', '', ( #3986 ) ) ;
#8131=CARTESIAN_POINT ( 'NONE',  ( 38.29999999999999005, 13.62011893735970958, 95.42841645007781892 ) ) ;
#8132=ORIENTED_EDGE ( 'NONE', *, *, #9835, .T. ) ;
#8133=EDGE_CURVE ( 'NONE', #6810, #1088, #3304, .T. ) ;
#8136=CARTESIAN_POINT ( 'NONE',  ( 34.77500000054621410, 17.63344945572770328, 83.50966788445364841 ) ) ;
#8138=EDGE_CURVE ( 'NONE', #10066, #5241, #11512, .T. ) ;
#8140=CARTESIAN_POINT ( 'NONE',  ( 37.57500000054623257, 26.19570976099943493, 95.29460816699764791 ) ) ;
#8141=CARTESIAN_POINT ( 'NONE',  ( 38.59999999999998721, 12.86707612778636012, 88.47553407664152303 ) ) ;
#8142=CARTESIAN_POINT ( 'NONE',  ( 43.37500000054622973, 26.92701409722686634, 93.04388485072563242 ) ) ;
#8144=CARTESIAN_POINT ( 'NONE',  ( 27.55000000109246017, 22.43689772174679575, 98.29316153445363113 ) ) ;
#8149=EDGE_LOOP ( 'NONE', ( #1737, #6, #712, #7045 ) ) ;
#8150=CYLINDRICAL_SURFACE ( 'NONE', #4855, 7.499999999999992895 ) ;
#8152=CARTESIAN_POINT ( 'NONE',  ( 25.79999999999998650, 24.40838939219354842, 96.86078899226572503 ) ) ;
#8153=EDGE_CURVE ( 'NONE', #10690, #1585, #7615, .T. ) ;
#8154=CARTESIAN_POINT ( 'NONE',  ( 29.67500000054623044, 22.36655054427230027, 98.07665518445361386 ) ) ;
#8155=CARTESIAN_POINT ( 'NONE',  ( 27.67500000054622333, 24.28113015263587116, 96.68563167572563088 ) ) ;
#8156=CARTESIAN_POINT ( 'NONE',  ( -111.8465843842649292, 84.49999999999998579, 101.8533255156881978 ) ) ;
#8158=VERTEX_POINT ( 'NONE', #9581 ) ;
#8159=EDGE_CURVE ( 'NONE', #10297, #10983, #3552, .T. ) ;
#8160=CARTESIAN_POINT ( 'NONE',  ( 46.75000000109246656, 22.43689772174679575, 83.29316153445363113 ) ) ;
#8163=CARTESIAN_POINT ( 'NONE',  ( 34.72841614740047333, 18.00000000000000355, 152.2284161474004520 ) ) ;
#8164=( BOUNDED_CURVE ( )  B_SPLINE_CURVE ( 2, ( #6969, #3292, #6396, #11033, #7221, #7155, #9136, #9073, #5327, #7343, #9197 ),
 .UNSPECIFIED., .F., .F. ) 
 B_SPLINE_CURVE_WITH_KNOTS ( ( 3, 2, 2, 2, 2, 3 ),
 ( 0.6999999999999999556, 0.7066666666666666652, 0.7133333333333333748, 0.7199999999999999734, 0.7266666666666666829, 0.7333333333333332815 ),
 .UNSPECIFIED. ) 
 CURVE ( )  GEOMETRIC_REPRESENTATION_ITEM ( )  RATIONAL_B_SPLINE_CURVE ( ( 1.000000000000000000, 0.9510565162951535312, 1.000000000000000000, 0.9510565162951535312, 1.000000000000000000, 0.9510565162951535312, 1.000000000000000000, 0.9510565162951535312, 1.000000000000000000, 0.9510565162951535312, 1.000000000000000000 ) ) 
 REPRESENTATION_ITEM ( '' )  );
#8171=DIRECTION ( 'NONE',  ( 1.000000000000000000, -0.000000000000000000, -0.000000000000000000 ) ) ;
#8178=ORIENTED_EDGE ( 'NONE', *, *, #2963, .F. ) ;
#8182=CARTESIAN_POINT ( 'NONE',  ( 45.77500000054622120, 22.36655054427230027, 98.07665518445361386 ) ) ;
#8183=VECTOR ( 'NONE', #414, 1000.000000000000000 ) ;
#8184=CARTESIAN_POINT ( 'NONE',  ( 29.07500000054623257, 26.19570976099943849, 86.29171490190961435 ) ) ;
#8186=CARTESIAN_POINT ( 'NONE',  ( 45.45000000109246230, 24.40838939219354842, 96.86078899226572503 ) ) ;
#8188=CARTESIAN_POINT ( 'NONE',  ( 32.99999999999998579, 20.00000000000000355, 83.29316153445364534 ) ) ;
#8189=CYLINDRICAL_SURFACE ( 'NONE', #10923, 7.499999999999992895 ) ;
#8190=CARTESIAN_POINT ( 'NONE',  ( 29.07500000054623257, 26.19570976099943493, 86.29171490190961435 ) ) ;
#8192=CARTESIAN_POINT ( 'NONE',  ( 33.15000000109246514, 27.88596668178699645, 90.79316153445363113 ) ) ;
#8196=CIRCLE ( 'NONE', #6968, 7.500000000000000000 ) ;
#8197=CARTESIAN_POINT ( 'NONE',  ( 29.07500000054622191, 24.28113015263587471, 84.90069139318163138 ) ) ;
#8199=CARTESIAN_POINT ( 'NONE',  ( 48.07500000054623257, 13.80429023900056507, 95.29460816699764791 ) ) ;
#8200=CARTESIAN_POINT ( 'NONE',  ( 33.57500000054622546, 26.19570976099943493, 95.29460816699764791 ) ) ;
#8201=CARTESIAN_POINT ( 'NONE',  ( 36.69999999999999574, 13.62011893735971135, 86.15790661882942914 ) ) ;
#8203=CARTESIAN_POINT ( 'NONE',  ( 46.07500000054623257, 13.80429023900056507, 95.29460816699764791 ) ) ;
#8206=CARTESIAN_POINT ( 'NONE',  ( 26.65000000109246514, 20.00000000000000355, 83.29316153445364534 ) ) ;
#8208=VERTEX_POINT ( 'NONE', #9397 ) ;
#8213=CARTESIAN_POINT ( 'NONE',  ( 36.55000000109246372, 17.56310227825317583, 83.29316153445365956 ) ) ;
#8216=CARTESIAN_POINT ( 'NONE',  ( 23.07500000054622902, 26.19570976099943493, 86.29171490190961435 ) ) ;
#8217=CARTESIAN_POINT ( 'NONE',  ( 26.67500000054622333, 15.71886984736413773, 84.90069139318163138 ) ) ;
#8218=APPLICATION_CONTEXT ( 'automotive_design' ) ;
#8221=ORIENTED_EDGE ( 'NONE', *, *, #6023, .T. ) ;
#8222=CARTESIAN_POINT ( 'NONE',  ( 43.05000000109246372, 27.13292387221364876, 88.47553407664153724 ) ) ;
#8223=ORIENTED_EDGE ( 'NONE', *, *, #2784, .T. ) ;
#8224=LINE ( 'NONE', #2565, #9250 ) ;
#8226=ORIENTED_EDGE ( 'NONE', *, *, #11408, .F. ) ;
#8234=CARTESIAN_POINT ( 'NONE',  ( 22.89999999999998792, 17.56310227825320425, 83.29316153445363113 ) ) ;
#8237=CARTESIAN_POINT ( 'NONE',  ( 24.99999999999998579, 20.00000000000000355, 83.29316153445364534 ) ) ;
#8238=LINE ( 'NONE', #7276, #10243 ) ;
#8239=EDGE_CURVE ( 'NONE', #12263, #7138, #336, .T. ) ;
#8241=ORIENTED_EDGE ( 'NONE', *, *, #2784, .F. ) ;
#8242=CARTESIAN_POINT ( 'NONE',  ( -50.00000000000001421, 0.000000000000000000, 169.9999999999999716 ) ) ;
#8244=DIRECTION ( 'NONE',  ( 0.000000000000000000, 1.000000000000000000, 0.000000000000000000 ) ) ;
#8245=CARTESIAN_POINT ( 'NONE',  ( 47.27500000054622831, 26.92701409722686634, 88.54243821818162985 ) ) ;
#8246=AXIS2_PLACEMENT_3D ( 'NONE', #10259, #625, #1634 ) ;
#8247=CARTESIAN_POINT ( 'NONE',  ( 25.77500000054622831, 20.00000000000000355, 98.07665518445361386 ) ) ;
#8249=CARTESIAN_POINT ( 'NONE',  ( -50.00000000000001421, 22.00000000000000000, 152.2284161474004520 ) ) ;
#8250=CARTESIAN_POINT ( 'NONE',  ( 40.09999999999998721, 17.56310227825322556, 98.29316153445364534 ) ) ;
#8251=CARTESIAN_POINT ( 'NONE',  ( -50.00000000000001421, 20.00000000000000000, 145.0000000000000000 ) ) ;
#8252=EDGE_CURVE ( 'NONE', #3301, #7750, #1623, .T. ) ;
#8253=ORIENTED_EDGE ( 'NONE', *, *, #7470, .T. ) ;
#8257=CARTESIAN_POINT ( 'NONE',  ( 29.37500000054622618, 27.65831843345427998, 90.79316153445363113 ) ) ;
#8259=CARTESIAN_POINT ( 'NONE',  ( 44.67500000054622689, 17.63344945572770328, 83.50966788445364841 ) ) ;
#8260=CARTESIAN_POINT ( 'NONE',  ( 34.27500000054622120, 13.07298590277314254, 93.04388485072563242 ) ) ;
#8261=CARTESIAN_POINT ( 'NONE',  ( 34.89999999999997726, 17.56310227825321135, 83.29316153445363113 ) ) ;
#8262=AXIS2_PLACEMENT_3D ( 'NONE', #10429, #1802, #6747 ) ;
#8263=LINE ( 'NONE', #4, #3621 ) ;
#8264=CARTESIAN_POINT ( 'NONE',  ( 43.27500000054623541, 27.65831843345427998, 90.79316153445363113 ) ) ;
#8265=ORIENTED_EDGE ( 'NONE', *, *, #6076, .F. ) ;
#8266=CARTESIAN_POINT ( 'NONE',  ( 24.45000000109246585, 15.59161060780646046, 84.72553407664153724 ) ) ;
#8268=ORIENTED_EDGE ( 'NONE', *, *, #4049, .F. ) ;
#8270=ORIENTED_EDGE ( 'NONE', *, *, #11892, .T. ) ;
#8272=CIRCLE ( 'NONE', #7459, 7.499999999999978684 ) ;
#8273=CARTESIAN_POINT ( 'NONE',  ( 21.55000000109246372, 22.43689772174679575, 98.29316153445363113 ) ) ;
#8277=CARTESIAN_POINT ( 'NONE',  ( 23.37500000054622973, 26.92701409722686634, 93.04388485072563242 ) ) ;
#8278=CARTESIAN_POINT ( 'NONE',  ( 22.67500000054622333, 15.71886984736413773, 84.90069139318163138 ) ) ;
#8283=CARTESIAN_POINT ( 'NONE',  ( 42.05000000109246372, 12.86707612778636012, 93.11078899226572503 ) ) ;
#8285=ORIENTED_EDGE ( 'NONE', *, *, #8470, .F. ) ;
#8286=CARTESIAN_POINT ( 'NONE',  ( 30.15000000109246159, 12.11403331821300533, 90.79316153445363113 ) ) ;
#8290=( GEOMETRIC_REPRESENTATION_CONTEXT ( 3 ) GLOBAL_UNCERTAINTY_ASSIGNED_CONTEXT ( ( #12538 ) ) GLOBAL_UNIT_ASSIGNED_CONTEXT ( ( #11679, #3738, #7683 ) ) REPRESENTATION_CONTEXT ( 'NONE', 'WORKASPACE' ) );
#8291=CARTESIAN_POINT ( 'NONE',  ( 29.99999999999998934, 20.00000000000000355, 98.29316153445363113 ) ) ;
#8292=VECTOR ( 'NONE', #2382, 1000.000000000000000 ) ;
#8294=EDGE_CURVE ( 'NONE', #7244, #3052, #7762, .T. ) ;
#8296=DIRECTION ( 'NONE',  ( 0.000000000000000000, 0.000000000000000000, -1.000000000000000000 ) ) ;
#8297=CARTESIAN_POINT ( 'NONE',  ( 42.19999999999998863, 15.59161060780645691, 96.86078899226572503 ) ) ;
#8302=CARTESIAN_POINT ( 'NONE',  ( 23.69999999999998508, 26.37988106264029398, 95.42841645007781892 ) ) ;
#8307=CARTESIAN_POINT ( 'NONE',  ( 39.17500000054621978, 26.19570976099943493, 86.29171490190961435 ) ) ;
#8308=CARTESIAN_POINT ( 'NONE',  ( 26.67500000054622689, 17.63344945572770328, 83.50966788445364841 ) ) ;
#8309=CARTESIAN_POINT ( 'NONE',  ( 6.843143145516298098, 12.70774044341717968, 89.02228661475956528 ) ) ;
#8310=DIRECTION ( 'NONE',  ( 1.000000000000000000, 0.000000000000000000, 0.000000000000000000 ) ) ;
#8313=ORIENTED_EDGE ( 'NONE', *, *, #6049, .T. ) ;
#8315=DIRECTION ( 'NONE',  ( 1.000000000000000000, -0.000000000000000000, -0.000000000000000000 ) ) ;
#8322=CARTESIAN_POINT ( 'NONE',  ( 33.97500000054621694, 17.63344945572769973, 98.07665518445361386 ) ) ;
#8323=LINE ( 'NONE', #6229, #272 ) ;
#8324=CARTESIAN_POINT ( 'NONE',  ( 43.97500000054623115, 15.71886984736413417, 96.68563167572563088 ) ) ;
#8325=CARTESIAN_POINT ( 'NONE',  ( 32.87500000054622262, 20.00000000000000355, 83.50966788445364841 ) ) ;
#8326=CARTESIAN_POINT ( 'NONE',  ( 33.89999999999998437, 22.43689772174679575, 98.29316153445363113 ) ) ;
#8329=CARTESIAN_POINT ( 'NONE',  ( 40.27500000054623541, 12.34168156654572535, 90.79316153445363113 ) ) ;
#8331=CARTESIAN_POINT ( 'NONE',  ( 45.87500000054622973, 17.63344945572769973, 98.07665518445361386 ) ) ;
#8332=CARTESIAN_POINT ( 'NONE',  ( 28.45000000109246585, 15.59161060780646046, 84.72553407664153724 ) ) ;
#8339=CARTESIAN_POINT ( 'NONE',  ( 35.95000000109246940, 13.62011893735970958, 95.42841645007781892 ) ) ;
#8340=CARTESIAN_POINT ( 'NONE',  ( 31.85000000109246443, 15.59161060780645691, 96.86078899226572503 ) ) ;
#8341=CARTESIAN_POINT ( 'NONE',  ( 21.37500000054622618, 26.92701409722686634, 93.04388485072563242 ) ) ;
#8342=CARTESIAN_POINT ( 'NONE',  ( 22.07500000054622191, 15.71886984736413417, 96.68563167572563088 ) ) ;
#8346=CARTESIAN_POINT ( 'NONE',  ( 45.85000000109246798, 15.59161060780645691, 96.86078899226572503 ) ) ;
#8347=CARTESIAN_POINT ( 'NONE',  ( -5.000000000000004441, 22.00000000000000000, 152.2284161474004520 ) ) ;
#8349=CARTESIAN_POINT ( 'NONE',  ( 47.59999999999998721, 27.13292387221364876, 93.11078899226573924 ) ) ;
#8350=ORIENTED_EDGE ( 'NONE', *, *, #7992, .T. ) ;
#8351=DIRECTION ( 'NONE',  ( -0.000000000000000000, -0.000000000000000000, 1.000000000000000000 ) ) ;
#8363=CARTESIAN_POINT ( 'NONE',  ( 27.49999999999999645, 20.00000000000000355, 99.99999999999997158 ) ) ;
#8365=CARTESIAN_POINT ( 'NONE',  ( 35.47500000054623115, 26.19570976099943493, 95.29460816699764791 ) ) ;
#8366=CARTESIAN_POINT ( 'NONE',  ( 35.97500000054620983, 17.63344945572769973, 98.07665518445361386 ) ) ;
#8367=CARTESIAN_POINT ( 'NONE',  ( 24.87500000054622618, 22.36655054427230382, 83.50966788445364841 ) ) ;
#8368=CARTESIAN_POINT ( 'NONE',  ( 49.99999999999998579, 40.00000000000000000, 82.99999999999995737 ) ) ;
#8372=DIRECTION ( 'NONE',  ( 1.000000000000000000, -0.000000000000000000, -0.000000000000000000 ) ) ;
#8373=ORIENTED_EDGE ( 'NONE', *, *, #2722, .T. ) ;
#8375=ORIENTED_EDGE ( 'NONE', *, *, #9707, .T. ) ;
#8376=FACE_OUTER_BOUND ( 'NONE', #2962, .T. ) ;
#8377=ADVANCED_FACE ( 'NONE', ( #9899 ), #11107, .F. ) ;
#8378=VECTOR ( 'NONE', #10140, 1000.000000000000000 ) ;
#8379=CARTESIAN_POINT ( 'NONE',  ( 33.57500000054622546, 26.19570976099943849, 95.29460816699764791 ) ) ;
#8380=CARTESIAN_POINT ( 'NONE',  ( 27.15000000109246159, 27.88596668178699645, 90.79316153445363113 ) ) ;
#8382=CARTESIAN_POINT ( 'NONE',  ( 46.67500000054623399, 17.63344945572770328, 83.50966788445364841 ) ) ;
#8383=CARTESIAN_POINT ( 'NONE',  ( 33.47500000054622404, 26.92701409722686634, 93.04388485072563242 ) ) ;
#8384=CARTESIAN_POINT ( 'NONE',  ( 30.69999999999998863, 13.62011893735971135, 86.15790661882942914 ) ) ;
#8386=CARTESIAN_POINT ( 'NONE',  ( 41.67500000054622689, 22.36655054427230027, 98.07665518445361386 ) ) ;
#8389=CARTESIAN_POINT ( 'NONE',  ( 47.57500000054622546, 24.28113015263587116, 96.68563167572563088 ) ) ;
#8391=ORIENTED_EDGE ( 'NONE', *, *, #10849, .T. ) ;
#8392=EDGE_CURVE ( 'NONE', #1420, #113, #6808, .T. ) ;
#8394=ORIENTED_EDGE ( 'NONE', *, *, #11608, .F. ) ;
#8396=DIRECTION ( 'NONE',  ( 1.000000000000000000, -0.000000000000000000, -0.000000000000000000 ) ) ;
#8397=CARTESIAN_POINT ( 'NONE',  ( 49.99999999999998579, 20.00000000000000000, 145.0000000000000000 ) ) ;
#8398=CYLINDRICAL_SURFACE ( 'NONE', #9211, 7.500000000000000000 ) ;
#8400=CARTESIAN_POINT ( 'NONE',  ( 22.77500000054622831, 20.00000000000000355, 83.50966788445364841 ) ) ;
#8401=CARTESIAN_POINT ( 'NONE',  ( 23.87500000054622262, 20.00000000000000355, 98.07665518445361386 ) ) ;
#8403=CARTESIAN_POINT ( 'NONE',  ( 41.89999999999999147, 22.43689772174679575, 98.29316153445363113 ) ) ;
#8406=CARTESIAN_POINT ( 'NONE',  ( 37.45000000109246230, 24.40838939219354842, 96.86078899226572503 ) ) ;
#8409=CARTESIAN_POINT ( 'NONE',  ( -2.000000000000015543, 20.00000000000000355, 98.29316153445363113 ) ) ;
#8410=ORIENTED_EDGE ( 'NONE', *, *, #8511, .T. ) ;
#8411=CARTESIAN_POINT ( 'NONE',  ( 44.65000000109246514, 20.00000000000000355, 83.29316153445364534 ) ) ;
#8412=CARTESIAN_POINT ( 'NONE',  ( -5.000000000000000888, 18.00000000000000355, 169.9999999999999716 ) ) ;
#8416=CARTESIAN_POINT ( 'NONE',  ( -34.72841614740048044, 18.00000000000000355, 169.9999999999999716 ) ) ;
#8420=CARTESIAN_POINT ( 'NONE',  ( 22.67500000054622333, 17.63344945572770328, 83.50966788445364841 ) ) ;
#8427=CARTESIAN_POINT ( 'NONE',  ( 35.77500000054622831, 20.00000000000000355, 98.07665518445361386 ) ) ;
#8428=CARTESIAN_POINT ( 'NONE',  ( 35.87500000054622973, 20.00000000000000355, 98.07665518445361386 ) ) ;
#8430=CARTESIAN_POINT ( 'NONE',  ( 9.844533866065003025, 18.22526997752235189, 98.08466769849140121 ) ) ;
#8431=FACE_OUTER_BOUND ( 'NONE', #6249, .T. ) ;
#8432=CARTESIAN_POINT ( 'NONE',  ( 33.39999999999998437, 27.13292387221364876, 88.47553407664153724 ) ) ;
#8434=CARTESIAN_POINT ( 'NONE',  ( -2.000000000000015543, 20.00000000000000355, 83.29316153445364534 ) ) ;
#8439=( BOUNDED_CURVE ( )  B_SPLINE_CURVE ( 3, ( #1906, #10412, #1783, #5789 ),
 .UNSPECIFIED., .F., .F. ) 
 B_SPLINE_CURVE_WITH_KNOTS ( ( 4, 4 ),
 ( 1.570796326794896558, 3.141592653589793560 ),
 .UNSPECIFIED. ) 
 CURVE ( )  GEOMETRIC_REPRESENTATION_ITEM ( )  RATIONAL_B_SPLINE_CURVE ( ( 1.000000000000000000, 0.8047378541243649375, 0.8047378541243649375, 1.000000000000000000 ) ) 
 REPRESENTATION_ITEM ( '' )  );
#8440=CARTESIAN_POINT ( 'NONE',  ( 25.97500000054622049, 17.63344945572769973, 98.07665518445361386 ) ) ;
#8442=CARTESIAN_POINT ( 'NONE',  ( 48.27500000054622120, 12.34168156654572357, 90.79316153445363113 ) ) ;
#8443=CARTESIAN_POINT ( 'NONE',  ( 31.37500000054622618, 27.65831843345427998, 90.79316153445363113 ) ) ;
#8444=CARTESIAN_POINT ( 'NONE',  ( 27.69999999999998508, 26.37988106264029398, 95.42841645007781892 ) ) ;
#8445=EDGE_CURVE ( 'NONE', #9490, #5989, #446, .T. ) ;
#8447=CARTESIAN_POINT ( 'NONE',  ( 36.57500000054622546, 15.71886984736413773, 84.90069139318163138 ) ) ;
#8449=CARTESIAN_POINT ( 'NONE',  ( 49.37500000054622973, 26.92701409722686634, 93.04388485072563242 ) ) ;
#8455=EDGE_CURVE ( 'NONE', #11877, #9504, #1403, .T. ) ;
#8456=ORIENTED_EDGE ( 'NONE', *, *, #4672, .T. ) ;
#8457=LINE ( 'NONE', #4584, #11537 ) ;
#8459=CARTESIAN_POINT ( 'NONE',  ( 49.82500000054622546, 20.00000000000000355, 98.29316153445363113 ) ) ;
#8461=CARTESIAN_POINT ( 'NONE',  ( 25.27500000054622475, 27.65831843345427998, 90.79316153445363113 ) ) ;
#8462=CARTESIAN_POINT ( 'NONE',  ( 20.87500000054622262, 20.00000000000000355, 83.50966788445364841 ) ) ;
#8465=ORIENTED_EDGE ( 'NONE', *, *, #1424, .F. ) ;
#8466=CARTESIAN_POINT ( 'NONE',  ( 37.85000000109246798, 15.59161060780645691, 96.86078899226572503 ) ) ;
#8469=DIRECTION ( 'NONE',  ( 0.000000000000000000, 0.000000000000000000, -1.000000000000000000 ) ) ;
#8470=EDGE_CURVE ( 'NONE', #5557, #9392, #10152, .T. ) ;
#8475=ADVANCED_FACE ( 'NONE', ( #3357 ), #7227, .T. ) ;
#8476=VECTOR ( 'NONE', #9048, 1000.000000000000000 ) ;
#8478=CARTESIAN_POINT ( 'NONE',  ( 41.99999999999998579, 20.00000000000000355, 98.29316153445363113 ) ) ;
#8479=CARTESIAN_POINT ( 'NONE',  ( -50.00000000000001421, 20.00000000000000000, 145.0000000000000000 ) ) ;
#8481=CARTESIAN_POINT ( 'NONE',  ( 23.37500000054622973, 26.92701409722686634, 93.04388485072563242 ) ) ;
#8482=CYLINDRICAL_SURFACE ( 'NONE', #725, 7.499999999999992895 ) ;
#8484=VERTEX_POINT ( 'NONE', #8249 ) ;
#8487=CARTESIAN_POINT ( 'NONE',  ( 21.19999999999998508, 24.40838939219355197, 84.72553407664153724 ) ) ;
#8489=CARTESIAN_POINT ( 'NONE',  ( 40.87500000054622262, 20.00000000000000355, 83.50966788445364841 ) ) ;
#8490=CARTESIAN_POINT ( 'NONE',  ( 21.87500000054622973, 17.63344945572769973, 98.07665518445361386 ) ) ;
#8494=DIRECTION ( 'NONE',  ( 0.000000000000000000, -0.7071067811865440200, 0.7071067811865511255 ) ) ;
#8500=CARTESIAN_POINT ( 'NONE',  ( 25.07500000054622191, 24.28113015263587471, 84.90069139318163138 ) ) ;
#8501=DIRECTION ( 'NONE',  ( 1.000000000000000000, 0.000000000000000000, 0.000000000000000000 ) ) ;
#8502=CARTESIAN_POINT ( 'NONE',  ( 36.97500000054623115, 24.28113015263587471, 84.90069139318163138 ) ) ;
#8503=CARTESIAN_POINT ( 'NONE',  ( 27.47500000054622404, 26.92701409722686634, 93.04388485072563242 ) ) ;
#8504=CARTESIAN_POINT ( 'NONE',  ( 28.69999999999998863, 13.62011893735971135, 86.15790661882942914 ) ) ;
#8505=DIRECTION ( 'NONE',  ( -0.4999999999999892308, -0.000000000000000000, -0.8660254037844448138 ) ) ;
#8506=CARTESIAN_POINT ( 'NONE',  ( 39.07500000054621836, 26.19570976099943493, 86.29171490190961435 ) ) ;
#8507=ORIENTED_EDGE ( 'NONE', *, *, #8455, .F. ) ;
#8508=CARTESIAN_POINT ( 'NONE',  ( 49.07500000054622546, 26.19570976099943493, 86.29171490190961435 ) ) ;
#8511=EDGE_CURVE ( 'NONE', #8002, #9150, #4187, .T. ) ;
#8513=ORIENTED_EDGE ( 'NONE', *, *, #10927, .T. ) ;
#8514=( BOUNDED_CURVE ( )  B_SPLINE_CURVE ( 2, ( #1771, #8123, #2089, #11932, #9841, #2025, #11870, #8881, #8951, #10845, #5908 ),
 .UNSPECIFIED., .F., .F. ) 
 B_SPLINE_CURVE_WITH_KNOTS ( ( 3, 2, 2, 2, 2, 3 ),
 ( 0.000000000000000000, 0.006666666666666673166, 0.01333333333333334633, 0.02000000000000001429, 0.02666666666666669266, 0.03333333333333336063 ),
 .UNSPECIFIED. ) 
 CURVE ( )  GEOMETRIC_REPRESENTATION_ITEM ( )  RATIONAL_B_SPLINE_CURVE ( ( 1.000000000000000000, 0.9510565162951535312, 1.000000000000000000, 0.9510565162951535312, 1.000000000000000000, 0.9510565162951535312, 1.000000000000000000, 0.9510565162951535312, 1.000000000000000000, 0.9510565162951533091, 1.000000000000000222 ) ) 
 REPRESENTATION_ITEM ( '' )  );
#8515=CARTESIAN_POINT ( 'NONE',  ( -2.000000000000015543, 20.00000000000000355, 90.79316153445363113 ) ) ;
#8518=CARTESIAN_POINT ( 'NONE',  ( 46.27500000054622831, 13.07298590277314254, 93.04388485072563242 ) ) ;
#8519=LINE ( 'NONE', #8459, #2105 ) ;
#8520=CARTESIAN_POINT ( 'NONE',  ( 43.47500000054622404, 26.92701409722686634, 93.04388485072563242 ) ) ;
#8521=CARTESIAN_POINT ( 'NONE',  ( 45.89999999999999147, 22.43689772174679575, 98.29316153445363113 ) ) ;
#8523=CARTESIAN_POINT ( 'NONE',  ( 38.95000000109246230, 26.37988106264029398, 86.15790661882942914 ) ) ;
#8524=ORIENTED_EDGE ( 'NONE', *, *, #6839, .F. ) ;
#8525=CARTESIAN_POINT ( 'NONE',  ( 36.75000000109245946, 22.43689772174679575, 83.29316153445363113 ) ) ;
#8528=CYLINDRICAL_SURFACE ( 'NONE', #390, 7.499999999999992895 ) ;
#8533=EDGE_CURVE ( 'NONE', #12151, #7564, #7288, .T. ) ;
#8536=AXIS2_PLACEMENT_3D ( 'NONE', #696, #9458, #5712 ) ;
#8537=ADVANCED_FACE ( 'NONE', ( #2463 ), #10207, .F. ) ;
#8538=B_SPLINE_CURVE_WITH_KNOTS ( 'NONE', 3,
 ( #6518, #9571, #10896, #7917, #180, #9823, #4039, #3976, #11723, #8932, #2209, #11783, #10758, #10696, #307, #7854, #2069, #11663, #4102, #3088, #11849, #7980, #8045, #118, #3156, #8994, #51, #4171, #7022, #9760, #11914, #3221, #1069, #2969, #10964, #6955, #6081, #9951, #4932, #1257, #7791, #1200, #5067, #6835, #8800, #246, #5129, #7083, #2272, #2009, #6013, #6139, #10011, #4873 ),
 .UNSPECIFIED., .F., .F.,
 ( 4, 2, 2, 2, 2, 2, 2, 2, 2, 2, 2, 2, 2, 2, 2, 2, 2, 2, 2, 2, 2, 2, 2, 2, 2, 2, 4 ),
 ( 0.02456447672714493283, 0.02533051008357335709, 0.02609654344000177789, 0.02686257679643020216, 0.02762861015285862296, 0.02916067686571544720, 0.03069274357857226798, 0.03145877693500069572, 0.03222481029142912345, 0.03375687700428597893, 0.03452291036071443442, 0.03528894371714287603, 0.03605497707357133153, 0.03682101042999977314, 0.03758704378642822863, 0.03835307714285667025, 0.03988514385571360898, 0.04065117721214206448, 0.04141721056857051997, 0.04294927728142744483, 0.04371531063785590726, 0.04448134399428436969, 0.04601341070714128068, 0.04677944406356973617, 0.04754547741999817778, 0.04831151077642663327, 0.04907754413285508877 ),
 .UNSPECIFIED. ) ;
#8541=CARTESIAN_POINT ( 'NONE',  ( -50.00000000000001421, 20.00000000000000000, 137.5000000000000000 ) ) ;
#8542=EDGE_LOOP ( 'NONE', ( #727, #10687, #8619, #11198 ) ) ;
#8545=CARTESIAN_POINT ( 'NONE',  ( 19.97500000054623115, 15.71886984736413417, 96.68563167572563088 ) ) ;
#8548=VERTEX_POINT ( 'NONE', #6400 ) ;
#8550=ORIENTED_EDGE ( 'NONE', *, *, #879, .T. ) ;
#8551=CARTESIAN_POINT ( 'NONE',  ( 42.65000000109246514, 20.00000000000000355, 83.29316153445364534 ) ) ;
#8555=CARTESIAN_POINT ( 'NONE',  ( 49.82500000054622546, 20.00000000000000355, 98.07665518445361386 ) ) ;
#8558=CARTESIAN_POINT ( 'NONE',  ( -50.00000000000001421, 0.000000000000000000, 69.99999999999998579 ) ) ;
#8559=LINE ( 'NONE', #8434, #6891 ) ;
#8560=ORIENTED_EDGE ( 'NONE', *, *, #179, .F. ) ;
#8562=CARTESIAN_POINT ( 'NONE',  ( -50.00000000000001421, 40.00000000000000000, 169.9999999999999716 ) ) ;
#8564=CARTESIAN_POINT ( 'NONE',  ( 29.25000000109246301, 27.13292387221364876, 93.11078899226573924 ) ) ;
#8566=CARTESIAN_POINT ( 'NONE',  ( 36.57500000054622546, 15.71886984736413773, 84.90069139318163138 ) ) ;
#8567=CARTESIAN_POINT ( 'NONE',  ( 29.17500000054622333, 26.19570976099943493, 86.29171490190961435 ) ) ;
#8568=CARTESIAN_POINT ( 'NONE',  ( 26.99999999999998934, 20.00000000000000355, 83.29316153445364534 ) ) ;
#8569=CARTESIAN_POINT ( 'NONE',  ( 30.19999999999998863, 15.59161060780645691, 96.86078899226572503 ) ) ;
#8570=CARTESIAN_POINT ( 'NONE',  ( 40.77500000054622831, 20.00000000000000355, 83.50966788445364841 ) ) ;
#8571=VERTEX_POINT ( 'NONE', #10265 ) ;
#8572=CARTESIAN_POINT ( 'NONE',  ( 19.65000000109246514, 20.00000000000000355, 98.29316153445363113 ) ) ;
#8580=CARTESIAN_POINT ( 'NONE',  ( 41.87500000054622262, 20.00000000000000355, 98.07665518445361386 ) ) ;
#8582=ADVANCED_FACE ( 'NONE', ( #8431 ), #11407, .F. ) ;
#8583=CARTESIAN_POINT ( 'NONE',  ( 46.89999999999999147, 17.56310227825321135, 83.29316153445363113 ) ) ;
#8586=VERTEX_POINT ( 'NONE', #4618 ) ;
#8588=CARTESIAN_POINT ( 'NONE',  ( 39.35000000109246088, 26.37988106264029398, 95.42841645007781892 ) ) ;
#8591=DIRECTION ( 'NONE',  ( 1.000000000000000000, -0.000000000000000000, -0.000000000000000000 ) ) ;
#8595=AXIS2_PLACEMENT_3D ( 'NONE', #4402, #5178, #2436 ) ;
#8596=LINE ( 'NONE', #4603, #6359 ) ;
#8598=DIRECTION ( 'NONE',  ( 0.000000000000000000, -1.000000000000000000, 0.000000000000000000 ) ) ;
#8601=CARTESIAN_POINT ( 'NONE',  ( 27.65000000109246514, 20.00000000000000355, 98.29316153445363113 ) ) ;
#8603=CARTESIAN_POINT ( 'NONE',  ( 21.67500000054622689, 22.36655054427230027, 98.07665518445361386 ) ) ;
#8604=ORIENTED_EDGE ( 'NONE', *, *, #5218, .T. ) ;
#8606=VECTOR ( 'NONE', #5625, 1000.000000000000000 ) ;
#8607=CARTESIAN_POINT ( 'NONE',  ( 23.29999999999998650, 26.37988106264029398, 86.15790661882942914 ) ) ;
#8608=EDGE_LOOP ( 'NONE', ( #3271, #10623, #11670, #867, #9241, #8834 ) ) ;
#8609=ORIENTED_EDGE ( 'NONE', *, *, #12193, .F. ) ;
#8613=CARTESIAN_POINT ( 'NONE',  ( 22.27500000054622475, 12.34168156654572357, 90.79316153445363113 ) ) ;
#8619=ORIENTED_EDGE ( 'NONE', *, *, #5503, .T. ) ;
#8620=LINE ( 'NONE', #8562, #439 ) ;
#8623=CARTESIAN_POINT ( 'NONE',  ( 26.47500000054622404, 13.07298590277314432, 88.54243821818161564 ) ) ;
#8624=CARTESIAN_POINT ( 'NONE',  ( 36.49999999999998579, 12.11403331821300533, 90.79316153445363113 ) ) ;
#8625=CARTESIAN_POINT ( 'NONE',  ( 41.17500000054623399, 26.92701409722686634, 88.54243821818162985 ) ) ;
#8627=CARTESIAN_POINT ( 'NONE',  ( 26.67500000054622333, 15.71886984736413773, 84.90069139318163138 ) ) ;
#8628=CARTESIAN_POINT ( 'NONE',  ( 28.39999999999998792, 12.86707612778636012, 93.11078899226572503 ) ) ;
#8630=CARTESIAN_POINT ( 'NONE',  ( 35.77500000054622831, 20.00000000000000355, 98.07665518445361386 ) ) ;
#8631=ORIENTED_EDGE ( 'NONE', *, *, #5505, .F. ) ;
#8632=CARTESIAN_POINT ( 'NONE',  ( 45.27500000054622831, 27.65831843345427998, 90.79316153445363113 ) ) ;
#8638=DIRECTION ( 'NONE',  ( 1.000000000000000000, -0.000000000000000000, -0.000000000000000000 ) ) ;
#8639=CARTESIAN_POINT ( 'NONE',  ( 32.49999999999997868, 12.11403331821300533, 90.79316153445363113 ) ) ;
#8641=CARTESIAN_POINT ( 'NONE',  ( 45.07500000054622546, 24.28113015263587471, 84.90069139318163138 ) ) ;
#8644=CARTESIAN_POINT ( 'NONE',  ( 46.67500000054622689, 15.71886984736413773, 84.90069139318163138 ) ) ;
#8645=CARTESIAN_POINT ( 'NONE',  ( 47.89999999999999147, 22.43689772174679575, 98.29316153445363113 ) ) ;
#8647=CARTESIAN_POINT ( 'NONE',  ( 49.47500000054621694, 26.19570976099943493, 95.29460816699764791 ) ) ;
#8649=CARTESIAN_POINT ( 'NONE',  ( 37.25000000109246656, 27.13292387221364876, 93.11078899226573924 ) ) ;
#8659=CARTESIAN_POINT ( 'NONE',  ( 37.07500000054622546, 26.19570976099943493, 86.29171490190961435 ) ) ;
#8661=CARTESIAN_POINT ( 'NONE',  ( 27.29999999999998295, 26.37988106264029398, 86.15790661882942914 ) ) ;
#8662=VERTEX_POINT ( 'NONE', #12098 ) ;
#8663=DIRECTION ( 'NONE',  ( 1.000000000000000000, 0.000000000000000000, 0.000000000000000000 ) ) ;
#8665=CARTESIAN_POINT ( 'NONE',  ( 48.47500000054622404, 13.07298590277314432, 88.54243821818161564 ) ) ;
#8669=DIRECTION ( 'NONE',  ( 1.000000000000000000, -0.000000000000000000, -0.000000000000000000 ) ) ;
#8670=ORIENTED_EDGE ( 'NONE', *, *, #3894, .F. ) ;
#8675=CARTESIAN_POINT ( 'NONE',  ( 43.65000000109246514, 20.00000000000000355, 98.29316153445363113 ) ) ;
#8678=CARTESIAN_POINT ( 'NONE',  ( 19.97500000054623115, 15.71886984736413417, 96.68563167572563088 ) ) ;
#8680=DIRECTION ( 'NONE',  ( 1.000000000000000000, 0.000000000000000000, 0.000000000000000000 ) ) ;
#8689=CARTESIAN_POINT ( 'NONE',  ( 27.57500000054622191, 26.19570976099943849, 95.29460816699764791 ) ) ;
#8690=CARTESIAN_POINT ( 'NONE',  ( 24.05000000109246372, 12.86707612778636012, 93.11078899226572503 ) ) ;
#8691=CARTESIAN_POINT ( 'NONE',  ( 39.77500000054622831, 20.00000000000000355, 98.07665518445361386 ) ) ;
#8692=CARTESIAN_POINT ( 'NONE',  ( 27.67500000054622333, 24.28113015263587116, 96.68563167572563088 ) ) ;
#8693=CARTESIAN_POINT ( 'NONE',  ( 24.79999999999999005, 15.59161060780646046, 84.72553407664153724 ) ) ;
#8695=LINE ( 'NONE', #7619, #5662 ) ;
#8696=CARTESIAN_POINT ( 'NONE',  ( 34.77500000054622831, 20.00000000000000355, 83.50966788445364841 ) ) ;
#8697=ORIENTED_EDGE ( 'NONE', *, *, #7111, .F. ) ;
#8698=PLANE ( 'NONE',  #1022 ) ;
#8700=CARTESIAN_POINT ( 'NONE',  ( 49.65000000109246514, 20.00000000000000355, 98.29316153445363113 ) ) ;
#8704=VECTOR ( 'NONE', #8022, 1000.000000000000000 ) ;
#8705=CARTESIAN_POINT ( 'NONE',  ( 43.39999999999998437, 27.13292387221364876, 88.47553407664153724 ) ) ;
#8709=CARTESIAN_POINT ( 'NONE',  ( 49.69999999999998863, 26.37988106264029398, 95.42841645007781892 ) ) ;
#8711=CARTESIAN_POINT ( 'NONE',  ( 44.69999999999998153, 13.62011893735970958, 86.15790661882942914 ) ) ;
#8713=CARTESIAN_POINT ( 'NONE',  ( 31.55000000109246727, 22.43689772174679575, 98.29316153445363113 ) ) ;
#8716=VERTEX_POINT ( 'NONE', #4724 ) ;
#8720=LINE ( 'NONE', #33, #10204 ) ;
#8721=CARTESIAN_POINT ( 'NONE',  ( 35.17500000054622689, 26.92701409722686634, 88.54243821818162985 ) ) ;
#8722=CARTESIAN_POINT ( 'NONE',  ( 34.97500000054622404, 22.36655054427230382, 83.50966788445364841 ) ) ;
#8725=EDGE_LOOP ( 'NONE', ( #10568, #10037, #7621, #8631, #664, #1617, #9906, #10515, #7830 ) ) ;
#8733=ORIENTED_EDGE ( 'NONE', *, *, #3417, .T. ) ;
#8735=CARTESIAN_POINT ( 'NONE',  ( 43.35000000109246088, 26.37988106264029398, 95.42841645007781892 ) ) ;
#8737=CARTESIAN_POINT ( 'NONE',  ( -50.00000000000001421, 40.00000000000000000, 169.9999999999999716 ) ) ;
#8739=CARTESIAN_POINT ( 'NONE',  ( 37.89999999999999147, 22.43689772174674246, 98.29316153445367377 ) ) ;
#8746=CARTESIAN_POINT ( 'NONE',  ( 46.49999999999998579, 12.11403331821300533, 90.79316153445363113 ) ) ;
#8747=CARTESIAN_POINT ( 'NONE',  ( 48.97500000054622404, 22.36655054427230382, 83.50966788445364841 ) ) ;
#8748=CARTESIAN_POINT ( 'NONE',  ( 37.27500000054622831, 27.65831843345427998, 90.79316153445363113 ) ) ;
#8749=CARTESIAN_POINT ( 'NONE',  ( 22.87500000054622618, 20.00000000000000355, 83.50966788445364841 ) ) ;
#8750=CARTESIAN_POINT ( 'NONE',  ( 21.99999999999998934, 20.00000000000000355, 98.29316153445363113 ) ) ;
#8751=CARTESIAN_POINT ( 'NONE',  ( 34.29999999999996874, 13.62011893735970958, 95.42841645007781892 ) ) ;
#8752=CARTESIAN_POINT ( 'NONE',  ( 31.57500000054622902, 24.28113015263587116, 96.68563167572563088 ) ) ;
#8754=EDGE_CURVE ( 'NONE', #5847, #58, #9413, .T. ) ;
#8756=VERTEX_POINT ( 'NONE', #8412 ) ;
#8757=CARTESIAN_POINT ( 'NONE',  ( 49.05000000109246372, 27.13292387221364876, 88.47553407664153724 ) ) ;
#8760=LINE ( 'NONE', #1039, #940 ) ;
#8762=CARTESIAN_POINT ( 'NONE',  ( 45.67500000054621978, 24.28113015263587116, 96.68563167572563088 ) ) ;
#8763=CARTESIAN_POINT ( 'NONE',  ( -111.8465843842649292, 69.50000000000000000, 146.8533255156881978 ) ) ;
#8765=CARTESIAN_POINT ( 'NONE',  ( 44.97500000054621694, 22.36655054427230382, 83.50966788445364841 ) ) ;
#8766=CARTESIAN_POINT ( 'NONE',  ( 41.89999999999999858, 22.43689772174679575, 98.29316153445363113 ) ) ;
#8767=CARTESIAN_POINT ( 'NONE',  ( 39.49999999999997868, 27.88596668178699645, 90.79316153445363113 ) ) ;
#8770=ADVANCED_FACE ( 'NONE', ( #6563 ), #10491, .F. ) ;
#8771=VECTOR ( 'NONE', #6472, 1000.000000000000000 ) ;
#8772=CARTESIAN_POINT ( 'NONE',  ( 33.55000000109246372, 22.43689772174679575, 98.29316153445363113 ) ) ;
#8781=CARTESIAN_POINT ( 'NONE',  ( 39.17500000054623399, 26.92701409722686634, 88.54243821818162985 ) ) ;
#8782=CARTESIAN_POINT ( 'NONE',  ( 32.27500000054622831, 13.07298590277314254, 93.04388485072563242 ) ) ;
#8784=CARTESIAN_POINT ( 'NONE',  ( 35.65000000109246514, 20.00000000000000355, 98.29316153445363113 ) ) ;
#8790=LINE ( 'NONE', #6005, #12261 ) ;
#8791=ORIENTED_EDGE ( 'NONE', *, *, #7111, .T. ) ;
#8794=EDGE_LOOP ( 'NONE', ( #8955, #6393 ) ) ;
#8795=AXIS2_PLACEMENT_3D ( 'NONE', #3511, #2686, #7382 ) ;
#8800=CARTESIAN_POINT ( 'NONE',  ( 9.405136654060040513, 23.43083853196268507, 84.10547354511845697 ) ) ;
#8801=CARTESIAN_POINT ( 'NONE',  ( 37.49999999999999289, 27.88596668178699645, 90.79316153445363113 ) ) ;
#8802=CIRCLE ( 'NONE', #9615, 7.499999999999978684 ) ;
#8809=AXIS2_PLACEMENT_3D ( 'NONE', #1355, #2241, #5221 ) ;
#8810=CARTESIAN_POINT ( 'NONE',  ( 46.29999999999999005, 13.62011893735970958, 95.42841645007781892 ) ) ;
#8811=CARTESIAN_POINT ( 'NONE',  ( 23.75000000109246301, 17.56310227825320425, 98.29316153445363113 ) ) ;
#8812=CARTESIAN_POINT ( 'NONE',  ( 30.57500000054622902, 15.71886984736413773, 84.90069139318163138 ) ) ;
#8814=CARTESIAN_POINT ( 'NONE',  ( 22.09999999999998010, 17.56310227825320425, 98.29316153445363113 ) ) ;
#8816=CARTESIAN_POINT ( 'NONE',  ( 34.27500000054623541, 12.34168156654572535, 90.79316153445363113 ) ) ;
#8817=EDGE_LOOP ( 'NONE', ( #11288, #6209, #5309, #5039 ) ) ;
#8821=CARTESIAN_POINT ( 'NONE',  ( 19.82500000054622546, 20.00000000000000355, 98.29316153445363113 ) ) ;
#8826=CARTESIAN_POINT ( 'NONE',  ( 35.97500000054620983, 17.63344945572769973, 98.07665518445361386 ) ) ;
#8827=PLANE ( 'NONE',  #11401 ) ;
#8829=CARTESIAN_POINT ( 'NONE',  ( 10.00000000000000355, 20.00000000000000355, 98.29316153445363113 ) ) ;
#8830=CARTESIAN_POINT ( 'NONE',  ( 37.07500000054622546, 24.28113015263587471, 84.90069139318163138 ) ) ;
#8831=CARTESIAN_POINT ( 'NONE',  ( 42.19999999999998863, 15.59161060780645691, 96.86078899226572503 ) ) ;
#8832=CARTESIAN_POINT ( 'NONE',  ( 45.79999999999999005, 24.40838939219354842, 96.86078899226572503 ) ) ;
#8833=CARTESIAN_POINT ( 'NONE',  ( 44.49999999999999289, 12.11403331821300533, 90.79316153445363113 ) ) ;
#8834=ORIENTED_EDGE ( 'NONE', *, *, #764, .T. ) ;
#8836=CARTESIAN_POINT ( 'NONE',  ( 29.65000000109246514, 20.00000000000000355, 98.29316153445363113 ) ) ;
#8840=CYLINDRICAL_SURFACE ( 'NONE', #6834, 7.499999999999978684 ) ;
#8843=( BOUNDED_CURVE ( )  B_SPLINE_CURVE ( 2, ( #9018, #12122, #7292, #11935, #1220, #3180, #3300, #5151, #10035, #10916, #6100 ),
 .UNSPECIFIED., .F., .F. ) 
 B_SPLINE_CURVE_WITH_KNOTS ( ( 3, 2, 2, 2, 2, 3 ),
 ( 0.8666666666666666963, 0.8733333333333332948, 0.8800000000000000044, 0.8866666666666667140, 0.8933333333333333126, 0.9000000000000000222 ),
 .UNSPECIFIED. ) 
 CURVE ( )  GEOMETRIC_REPRESENTATION_ITEM ( )  RATIONAL_B_SPLINE_CURVE ( ( 1.000000000000000000, 0.9510565162951535312, 1.000000000000000000, 0.9510565162951535312, 1.000000000000000000, 0.9510565162951535312, 1.000000000000000000, 0.9510565162951535312, 1.000000000000000000, 0.9510565162951535312, 1.000000000000000000 ) ) 
 REPRESENTATION_ITEM ( '' )  );
#8844=CARTESIAN_POINT ( 'NONE',  ( 33.77500000054622831, 20.00000000000000355, 98.07665518445361386 ) ) ;
#8845=CARTESIAN_POINT ( 'NONE',  ( 31.47500000054622404, 26.92701409722686634, 93.04388485072563242 ) ) ;
#8847=LINE ( 'NONE', #5427, #2394 ) ;
#8849=CARTESIAN_POINT ( 'NONE',  ( 48.47500000054622404, 13.07298590277314432, 88.54243821818161564 ) ) ;
#8851=CARTESIAN_POINT ( 'NONE',  ( 47.75000000109245946, 17.56310227825320425, 98.29316153445363113 ) ) ;
#8853=ORIENTED_EDGE ( 'NONE', *, *, #8445, .F. ) ;
#8855=ORIENTED_EDGE ( 'NONE', *, *, #4672, .F. ) ;
#8858=CARTESIAN_POINT ( 'NONE',  ( -5.000000000000000888, 0.000000000000000000, 121.2488769092545198 ) ) ;
#8862=CARTESIAN_POINT ( 'NONE',  ( 34.99999999999999289, 20.00000000000000355, 83.29316153445364534 ) ) ;
#8864=VECTOR ( 'NONE', #1549, 1000.000000000000000 ) ;
#8865=CARTESIAN_POINT ( 'NONE',  ( 21.20617189303578698, 25.37779564132840804, 151.2938281069642130 ) ) ;
#8866=CARTESIAN_POINT ( 'NONE',  ( 37.09999999999998010, 22.43689772174681707, 83.29316153445364534 ) ) ;
#8868=CYLINDRICAL_SURFACE ( 'NONE', #6952, 7.499999999999992895 ) ;
#8870=CARTESIAN_POINT ( 'NONE',  ( 40.87500000054623683, 22.36655054427230382, 83.50966788445364841 ) ) ;
#8872=ORIENTED_EDGE ( 'NONE', *, *, #6277, .F. ) ;
#8875=CARTESIAN_POINT ( 'NONE',  ( 21.67500000054622333, 24.28113015263587116, 96.68563167572563088 ) ) ;
#8876=CARTESIAN_POINT ( 'NONE',  ( 24.55000000109246017, 17.56310227825320425, 83.29316153445363113 ) ) ;
#8877=CARTESIAN_POINT ( 'NONE',  ( 30.07500000054622546, 13.80429023900056507, 95.29460816699764791 ) ) ;
#8879=CARTESIAN_POINT ( 'NONE',  ( 22.07500000054622191, 15.71886984736413417, 96.68563167572563088 ) ) ;
#8880=CARTESIAN_POINT ( 'NONE',  ( 26.19999999999998863, 15.59161060780645691, 96.86078899226572503 ) ) ;
#8881=CARTESIAN_POINT ( 'NONE',  ( 49.29999999999998295, 26.37988106264029398, 86.15790661882942914 ) ) ;
#8882=CARTESIAN_POINT ( 'NONE',  ( 35.97500000054623115, 15.71886984736413417, 96.68563167572563088 ) ) ;
#8888=CARTESIAN_POINT ( 'NONE',  ( 38.99999999999998579, 20.00000000000000355, 83.29316153445364534 ) ) ;
#8889=EDGE_LOOP ( 'NONE', ( #2502, #10097, #1860, #11243 ) ) ;
#8890=VECTOR ( 'NONE', #7477, 1000.000000000000000 ) ;
#8894=CARTESIAN_POINT ( 'NONE',  ( 40.77500000054622120, 17.63344945572770328, 83.50966788445364841 ) ) ;
#8895=CYLINDRICAL_SURFACE ( 'NONE', #11809, 7.499999999999978684 ) ;
#8896=CARTESIAN_POINT ( 'NONE',  ( 49.27500000054622831, 27.65831843345427998, 90.79316153445363113 ) ) ;
#8897=CARTESIAN_POINT ( 'NONE',  ( 45.39999999999999147, 27.13292387221364876, 88.47553407664153724 ) ) ;
#8899=EDGE_CURVE ( 'NONE', #3460, #8756, #6934, .T. ) ;
#8900=CARTESIAN_POINT ( 'NONE',  ( -23.10660171779821326, 12.50000000000000888, 140.6066017177982133 ) ) ;
#8902=CARTESIAN_POINT ( 'NONE',  ( 30.65000000109246514, 20.00000000000000355, 83.29316153445364534 ) ) ;
#8904=VERTEX_POINT ( 'NONE', #7063 ) ;
#8905=AXIS2_PLACEMENT_3D ( 'NONE', #2490, #1546, #596 ) ;
#8906=VERTEX_POINT ( 'NONE', #1925 ) ;
#8907=CARTESIAN_POINT ( 'NONE',  ( 0.000000000000000000, 0.000000000000000000, 169.9999999999999716 ) ) ;
#8909=FACE_OUTER_BOUND ( 'NONE', #6964, .T. ) ;
#8910=CARTESIAN_POINT ( 'NONE',  ( 29.17500000054623044, 26.92701409722686634, 88.54243821818162985 ) ) ;
#8911=CARTESIAN_POINT ( 'NONE',  ( 29.07500000054622191, 24.28113015263587471, 84.90069139318163138 ) ) ;
#8914=CARTESIAN_POINT ( 'NONE',  ( -111.8465843842649292, 69.50000000000000000, 146.8533255156881978 ) ) ;
#8916=CARTESIAN_POINT ( 'NONE',  ( 48.97500000054621694, 22.36655054427230382, 83.50966788445364841 ) ) ;
#8918=CARTESIAN_POINT ( 'NONE',  ( -2.000000000000015543, 20.00000000000000355, 83.29316153445364534 ) ) ;
#8919=VERTEX_POINT ( 'NONE', #227 ) ;
#8921=VECTOR ( 'NONE', #10051, 1000.000000000000000 ) ;
#8922=ADVANCED_FACE ( 'NONE', ( #3134 ), #8840, .F. ) ;
#8926=( BOUNDED_CURVE ( )  B_SPLINE_CURVE ( 2, ( #8291, #4539, #1567, #5250, #7458, #492, #7394, #9121, #3466, #6442, #5439 ),
 .UNSPECIFIED., .F., .F. ) 
 B_SPLINE_CURVE_WITH_KNOTS ( ( 3, 2, 2, 2, 2, 3 ),
 ( 0.6666666666666666297, 0.6733333333333333393, 0.6800000000000000488, 0.6866666666666666474, 0.6933333333333333570, 0.6999999999999999556 ),
 .UNSPECIFIED. ) 
 CURVE ( )  GEOMETRIC_REPRESENTATION_ITEM ( )  RATIONAL_B_SPLINE_CURVE ( ( 1.000000000000000000, 0.9510565162951535312, 1.000000000000000000, 0.9510565162951535312, 1.000000000000000000, 0.9510565162951535312, 1.000000000000000000, 0.9510565162951535312, 1.000000000000000000, 0.9510565162951535312, 1.000000000000000000 ) ) 
 REPRESENTATION_ITEM ( '' )  );
#8927=CARTESIAN_POINT ( 'NONE',  ( -5.000000000000004441, 40.00000000000000000, 69.99999999999998579 ) ) ;
#8930=DIRECTION ( 'NONE',  ( -1.000000000000000000, 0.000000000000000000, 0.000000000000000000 ) ) ;
#8932=CARTESIAN_POINT ( 'NONE',  ( 9.408430673389327481, 23.42179483032959197, 97.48547108980501719 ) ) ;
#8938=CARTESIAN_POINT ( 'NONE',  ( 43.67500000054621978, 22.36655054427230027, 98.07665518445361386 ) ) ;
#8940=EDGE_LOOP ( 'NONE', ( #2047, #11369, #10752, #5418 ) ) ;
#8945=CARTESIAN_POINT ( 'NONE',  ( 23.67500000054622333, 24.28113015263587116, 96.68563167572563088 ) ) ;
#8946=CARTESIAN_POINT ( 'NONE',  ( 24.45000000109246585, 15.59161060780646046, 84.72553407664153724 ) ) ;
#8948=CARTESIAN_POINT ( 'NONE',  ( 30.77500000054622831, 20.00000000000000355, 83.50966788445364841 ) ) ;
#8949=CARTESIAN_POINT ( 'NONE',  ( 23.27500000054622475, 26.92701409722686634, 88.54243821818162985 ) ) ;
#8950=CARTESIAN_POINT ( 'NONE',  ( 21.69999999999998508, 26.37988106264029398, 95.42841645007781892 ) ) ;
#8951=CARTESIAN_POINT ( 'NONE',  ( 49.19999999999998863, 24.40838939219355197, 84.72553407664153724 ) ) ;
#8952=CARTESIAN_POINT ( 'NONE',  ( 24.27500000054622475, 12.34168156654572535, 90.79316153445363113 ) ) ;
#8953=VERTEX_POINT ( 'NONE', #2431 ) ;
#8955=ORIENTED_EDGE ( 'NONE', *, *, #2881, .F. ) ;
#8959=CARTESIAN_POINT ( 'NONE',  ( 41.27500000054622120, 26.92701409722686634, 88.54243821818162985 ) ) ;
#8960=CARTESIAN_POINT ( 'NONE',  ( -10.00000000000000355, 20.00000000000000355, 109.9999999999999858 ) ) ;
#8962=CARTESIAN_POINT ( 'NONE',  ( 38.97500000054623115, 22.36655054427230382, 83.50966788445364841 ) ) ;
#8963=CARTESIAN_POINT ( 'NONE',  ( 39.39999999999999147, 27.13292387221364876, 88.47553407664153724 ) ) ;
#8964=CARTESIAN_POINT ( 'NONE',  ( 46.37500000054622973, 13.07298590277314432, 88.54243821818161564 ) ) ;
#8965=EDGE_LOOP ( 'NONE', ( #10463, #10063, #12170, #559 ) ) ;
#8966=CARTESIAN_POINT ( 'NONE',  ( 33.35000000109246798, 26.37988106264029398, 95.42841645007781892 ) ) ;
#8972=DIRECTION ( 'NONE',  ( 0.000000000000000000, 0.000000000000000000, -1.000000000000000000 ) ) ;
#8976=CARTESIAN_POINT ( 'NONE',  ( 29.07500000054623257, 26.19570976099943493, 86.29171490190961435 ) ) ;
#8977=CARTESIAN_POINT ( 'NONE',  ( 30.47500000054622404, 13.07298590277314432, 88.54243821818161564 ) ) ;
#8979=CARTESIAN_POINT ( 'NONE',  ( 39.65000000109246514, 20.00000000000000355, 98.29316153445363113 ) ) ;
#8981=CARTESIAN_POINT ( 'NONE',  ( 34.45000000109246940, 15.59161060780646046, 84.72553407664153724 ) ) ;
#8982=ORIENTED_EDGE ( 'NONE', *, *, #8159, .T. ) ;
#8983=CARTESIAN_POINT ( 'NONE',  ( 49.57500000054621836, 26.19570976099943849, 95.29460816699764791 ) ) ;
#8984=CARTESIAN_POINT ( 'NONE',  ( 48.05000000109247082, 12.86707612778636012, 93.11078899226572503 ) ) ;
#8986=LINE ( 'NONE', #3215, #1345 ) ;
#8990=CARTESIAN_POINT ( 'NONE',  ( 49.87500000054622262, 20.00000000000000355, 98.07665518445361386 ) ) ;
#8992=CARTESIAN_POINT ( 'NONE',  ( -34.99999999999999289, 15.60660171779821681, 137.4999999999999716 ) ) ;
#8993=EDGE_CURVE ( 'NONE', #5802, #10066, #10119, .T. ) ;
#8994=CARTESIAN_POINT ( 'NONE',  ( 6.629859784148791846, 27.48642350972822612, 91.31199581522203346 ) ) ;
#8995=CARTESIAN_POINT ( 'NONE',  ( -2.000000000000015543, 20.00000000000000355, 90.79316153445363113 ) ) ;
#9001=CARTESIAN_POINT ( 'NONE',  ( 44.47500000054622404, 13.80429023900056684, 86.29171490190961435 ) ) ;
#9005=VERTEX_POINT ( 'NONE', #7252 ) ;
#9006=( BOUNDED_CURVE ( )  B_SPLINE_CURVE ( 2, ( #4927, #7594, #9690, #7530, #6571, #9564, #1937, #10565, #3711, #4735, #7721 ),
 .UNSPECIFIED., .F., .F. ) 
 B_SPLINE_CURVE_WITH_KNOTS ( ( 3, 2, 2, 2, 2, 3 ),
 ( 0.1000000000000000888, 0.1066666666666667151, 0.1133333333333333276, 0.1199999999999999678, 0.1266666666666665941, 0.1333333333333332205 ),
 .UNSPECIFIED. ) 
 CURVE ( )  GEOMETRIC_REPRESENTATION_ITEM ( )  RATIONAL_B_SPLINE_CURVE ( ( 0.9999999999999994449, 0.9510565162951540863, 1.000000000000000000, 0.9510565162951535312, 1.000000000000000000, 0.9510565162951535312, 1.000000000000000000, 0.9510565162951535312, 1.000000000000000000, 0.9510565162951543083, 0.9999999999999992228 ) ) 
 REPRESENTATION_ITEM ( '' )  );
#9009=CARTESIAN_POINT ( 'NONE',  ( 46.59999999999998721, 12.86707612778636012, 88.47553407664152303 ) ) ;
#9010=CARTESIAN_POINT ( 'NONE',  ( 44.07500000054622546, 15.71886984736413417, 96.68563167572563088 ) ) ;
#9011=CARTESIAN_POINT ( 'NONE',  ( 32.97500000054622404, 24.28113015263587471, 84.90069139318163138 ) ) ;
#9012=CARTESIAN_POINT ( 'NONE',  ( 23.07500000054622546, 24.28113015263587471, 84.90069139318163138 ) ) ;
#9013=DIRECTION ( 'NONE',  ( -0.000000000000000000, 1.000000000000000000, 0.000000000000000000 ) ) ;
#9015=CARTESIAN_POINT ( 'NONE',  ( 27.57500000054622902, 24.28113015263587116, 96.68563167572563088 ) ) ;
#9017=EDGE_CURVE ( 'NONE', #3374, #5229, #260, .T. ) ;
#9018=CARTESIAN_POINT ( 'NONE',  ( 23.65000000109246514, 20.00000000000000355, 98.29316153445363113 ) ) ;
#9020=ORIENTED_EDGE ( 'NONE', *, *, #7484, .T. ) ;
#9021=AXIS2_PLACEMENT_3D ( 'NONE', #11433, #2744, #207 ) ;
#9026=CARTESIAN_POINT ( 'NONE',  ( 37.67500000054621978, 24.28113015263587116, 96.68563167572563088 ) ) ;
#9028=CARTESIAN_POINT ( 'NONE',  ( 26.99999999999998934, 20.00000000000000355, 83.29316153445364534 ) ) ;
#9029=CARTESIAN_POINT ( 'NONE',  ( 39.47500000054622404, 26.92701409722686634, 93.04388485072563242 ) ) ;
#9030=CARTESIAN_POINT ( 'NONE',  ( 43.39999999999998437, 27.13292387221364876, 88.47553407664153724 ) ) ;
#9032=CARTESIAN_POINT ( 'NONE',  ( 45.67500000054621978, 22.36655054427230027, 98.07665518445361386 ) ) ;
#9033=EDGE_LOOP ( 'NONE', ( #1814, #12356, #452, #10750, #11063 ) ) ;
#9034=CARTESIAN_POINT ( 'NONE',  ( 24.35000000109246798, 13.62011893735971135, 86.15790661882942914 ) ) ;
#9038=VECTOR ( 'NONE', #5133, 1000.000000000000000 ) ;
#9040=CARTESIAN_POINT ( 'NONE',  ( 24.65000000109246514, 20.00000000000000355, 83.29316153445364534 ) ) ;
#9043=CARTESIAN_POINT ( 'NONE',  ( 48.49999999999998579, 12.11403331821300533, 90.79316153445363113 ) ) ;
#9045=CARTESIAN_POINT ( 'NONE',  ( 32.67500000054622689, 17.63344945572770328, 83.50966788445364841 ) ) ;
#9046=CARTESIAN_POINT ( 'NONE',  ( 30.37500000054622618, 12.34168156654572535, 90.79316153445363113 ) ) ;
#9048=DIRECTION ( 'NONE',  ( 1.000000000000000000, -0.000000000000000000, -0.000000000000000000 ) ) ;
#9050=CARTESIAN_POINT ( 'NONE',  ( 42.35000000109246798, 13.62011893735971135, 86.15790661882942914 ) ) ;
#9053=EDGE_CURVE ( 'NONE', #9486, #1716, #11125, .T. ) ;
#9054=DIRECTION ( 'NONE',  ( 0.7071067811865489050, -0.000000000000000000, 0.7071067811865460184 ) ) ;
#9055=ORIENTED_EDGE ( 'NONE', *, *, #7383, .F. ) ;
#9057=AXIS2_PLACEMENT_3D ( 'NONE', #11153, #6395, #1512 ) ;
#9061=CARTESIAN_POINT ( 'NONE',  ( 37.95000000109246940, 13.62011893735970958, 95.42841645007781892 ) ) ;
#9062=CARTESIAN_POINT ( 'NONE',  ( 22.59999999999998721, 12.86707612778636012, 88.47553407664152303 ) ) ;
#9063=PLANE ( 'NONE',  #9221 ) ;
#9069=ORIENTED_EDGE ( 'NONE', *, *, #854, .T. ) ;
#9073=CARTESIAN_POINT ( 'NONE',  ( 28.29999999999998650, 13.62011893735970958, 95.42841645007781892 ) ) ;
#9074=CARTESIAN_POINT ( 'NONE',  ( 45.57500000054621836, 26.19570976099943493, 95.29460816699764791 ) ) ;
#9075=CARTESIAN_POINT ( 'NONE',  ( 30.47500000054622404, 13.80429023900056684, 86.29171490190961435 ) ) ;
#9076=CARTESIAN_POINT ( 'NONE',  ( 7.061376757456052644, 12.91846277011745592, 93.27565706701507509 ) ) ;
#9078=CARTESIAN_POINT ( 'NONE',  ( 20.27158385259951956, 18.00000000000000355, 170.0000119999999697 ) ) ;
#9079=CARTESIAN_POINT ( 'NONE',  ( 25.77500000054622831, 20.00000000000000355, 98.07665518445361386 ) ) ;
#9081=CARTESIAN_POINT ( 'NONE',  ( -6.999999999999999112, 92.00000000000000000, 166.8533255156881694 ) ) ;
#9084=CARTESIAN_POINT ( 'NONE',  ( 38.49999999999999289, 12.11403331821300533, 90.79316153445363113 ) ) ;
#9086=EDGE_CURVE ( 'NONE', #7706, #2249, #4621, .T. ) ;
#9088=VECTOR ( 'NONE', #5239, 1000.000000000000000 ) ;
#9089=CARTESIAN_POINT ( 'NONE',  ( 40.57500000054621836, 13.80429023900056684, 86.29171490190961435 ) ) ;
#9093=CARTESIAN_POINT ( 'NONE',  ( 39.07500000054622546, 24.28113015263587471, 84.90069139318163138 ) ) ;
#9094=CARTESIAN_POINT ( 'NONE',  ( 37.49999999999999289, 27.88596668178699645, 90.79316153445363113 ) ) ;
#9095=CARTESIAN_POINT ( 'NONE',  ( 43.67500000054621978, 22.36655054427230027, 98.07665518445361386 ) ) ;
#9097=CARTESIAN_POINT ( 'NONE',  ( 26.55000000109246017, 17.56310227825321135, 83.29316153445363113 ) ) ;
#9100=EDGE_CURVE ( 'NONE', #1088, #10690, #5730, .T. ) ;
#9102=CYLINDRICAL_SURFACE ( 'NONE', #11572, 7.499999999999992895 ) ;
#9106=CARTESIAN_POINT ( 'NONE',  ( -50.00000000000001421, 0.000000000000000000, 169.9999999999999716 ) ) ;
#9108=CARTESIAN_POINT ( 'NONE',  ( 28.67500000054623044, 17.63344945572770328, 83.50966788445364841 ) ) ;
#9109=CARTESIAN_POINT ( 'NONE',  ( 25.67500000054622333, 24.28113015263587116, 96.68563167572563088 ) ) ;
#9113=ORIENTED_EDGE ( 'NONE', *, *, #6078, .T. ) ;
#9114=CARTESIAN_POINT ( 'NONE',  ( 45.45000000109246230, 24.40838939219354842, 96.86078899226572503 ) ) ;
#9117=DIRECTION ( 'NONE',  ( 0.000000000000000000, 0.000000000000000000, -1.000000000000000000 ) ) ;
#9121=CARTESIAN_POINT ( 'NONE',  ( 29.29999999999998650, 26.37988106264029398, 86.15790661882942914 ) ) ;
#9122=CARTESIAN_POINT ( 'NONE',  ( 37.65000000109246514, 20.00000000000000355, 98.29316153445363113 ) ) ;
#9124=( BOUNDED_CURVE ( )  B_SPLINE_CURVE ( 2, ( #9253, #5508, #5444, #4543, #7274, #434, #554, #10196, #8297, #10309, #6389 ),
 .UNSPECIFIED., .F., .F. ) 
 B_SPLINE_CURVE_WITH_KNOTS ( ( 3, 2, 2, 2, 2, 3 ),
 ( 0.2333333333333333093, 0.2399999999999999634, 0.2466666666666666452, 0.2533333333333333548, 0.2600000000000000089, 0.2666666666666666630 ),
 .UNSPECIFIED. ) 
 CURVE ( )  GEOMETRIC_REPRESENTATION_ITEM ( )  RATIONAL_B_SPLINE_CURVE ( ( 1.000000000000000222, 0.9510565162951533091, 1.000000000000000000, 0.9510565162951535312, 1.000000000000000000, 0.9510565162951535312, 1.000000000000000000, 0.9510565162951535312, 1.000000000000000000, 0.9510565162951535312, 1.000000000000000000 ) ) 
 REPRESENTATION_ITEM ( '' )  );
#9125=AXIS2_PLACEMENT_3D ( 'NONE', #3807, #11553, #137 ) ;
#9136=CARTESIAN_POINT ( 'NONE',  ( 28.39999999999998792, 12.86707612778636012, 93.11078899226572503 ) ) ;
#9137=CARTESIAN_POINT ( 'NONE',  ( 42.77500000054622831, 17.63344945572770328, 83.50966788445364841 ) ) ;
#9138=CARTESIAN_POINT ( 'NONE',  ( 24.67500000054622689, 17.63344945572770328, 83.50966788445364841 ) ) ;
#9141=CARTESIAN_POINT ( 'NONE',  ( 35.49999999999998579, 27.88596668178699645, 90.79316153445363113 ) ) ;
#9143=CARTESIAN_POINT ( 'NONE',  ( 27.17500000054622689, 26.92701409722686634, 88.54243821818162985 ) ) ;
#9147=CARTESIAN_POINT ( 'NONE',  ( 33.35000000109246088, 26.37988106264029398, 95.42841645007781892 ) ) ;
#9148=VERTEX_POINT ( 'NONE', #10290 ) ;
#9150=VERTEX_POINT ( 'NONE', #11375 ) ;
#9152=CARTESIAN_POINT ( 'NONE',  ( 33.47500000054622404, 26.92701409722686634, 93.04388485072563242 ) ) ;
#9154=CARTESIAN_POINT ( 'NONE',  ( 42.87500000054622262, 22.36655054427230382, 83.50966788445364841 ) ) ;
#9155=CARTESIAN_POINT ( 'NONE',  ( 31.57500000054622191, 26.19570976099943493, 95.29460816699764791 ) ) ;
#9156=CARTESIAN_POINT ( 'NONE',  ( 38.69999999999998863, 13.62011893735971135, 86.15790661882942914 ) ) ;
#9158=CARTESIAN_POINT ( 'NONE',  ( 47.17500000054623399, 26.92701409722686634, 88.54243821818162985 ) ) ;
#9160=CARTESIAN_POINT ( 'NONE',  ( 24.25000000109246301, 12.86707612778636012, 88.47553407664152303 ) ) ;
#9165=CARTESIAN_POINT ( 'NONE',  ( -34.72841614740047333, 18.00000000000000355, 152.2284161474004520 ) ) ;
#9166=CARTESIAN_POINT ( 'NONE',  ( 23.99529484836403626, 12.50000000000001066, 148.5047051516359318 ) ) ;
#9169=CARTESIAN_POINT ( 'NONE',  ( 23.17500000054622689, 26.92701409722686634, 88.54243821818162985 ) ) ;
#9170=CARTESIAN_POINT ( 'NONE',  ( 25.17500000054622689, 26.19570976099943493, 86.29171490190961435 ) ) ;
#9174=ORIENTED_EDGE ( 'NONE', *, *, #737, .T. ) ;
#9175=CARTESIAN_POINT ( 'NONE',  ( 42.45000000109246940, 15.59161060780646046, 84.72553407664153724 ) ) ;
#9183=CARTESIAN_POINT ( 'NONE',  ( -2.000000000000015543, 20.00000000000000355, 90.79316153445363113 ) ) ;
#9184=AXIS2_PLACEMENT_3D ( 'NONE', #11813, #1973, #2169 ) ;
#9185=ADVANCED_FACE ( 'NONE', ( #5605 ), #12326, .F. ) ;
#9187=CARTESIAN_POINT ( 'NONE',  ( 0.000000000000000000, 18.00000000000000355, 169.9999999999999716 ) ) ;
#9190=DIRECTION ( 'NONE',  ( 1.000000000000000000, -0.000000000000000000, -0.000000000000000000 ) ) ;
#9196=CARTESIAN_POINT ( 'NONE',  ( 34.72841614740047333, 18.00000000000000355, 169.9999999999999716 ) ) ;
#9197=CARTESIAN_POINT ( 'NONE',  ( 27.99999999999998579, 20.00000000000000355, 98.29316153445363113 ) ) ;
#9198=CARTESIAN_POINT ( 'NONE',  ( 44.27500000054622120, 13.07298590277314254, 93.04388485072563242 ) ) ;
#9200=CARTESIAN_POINT ( 'NONE',  ( 23.87500000054622618, 17.63344945572769973, 98.07665518445361386 ) ) ;
#9203=PRODUCT_DEFINITION_FORMATION_WITH_SPECIFIED_SOURCE ( 'ANY', '', #8127, .NOT_KNOWN. ) ;
#9204=CARTESIAN_POINT ( 'NONE',  ( 31.79999999999998650, 24.40838939219354842, 96.86078899226572503 ) ) ;
#9207=EDGE_LOOP ( 'NONE', ( #5803, #10158, #1423, #6048, #6161 ) ) ;
#9208=EDGE_CURVE ( 'NONE', #4057, #10641, #7216, .T. ) ;
#9211=AXIS2_PLACEMENT_3D ( 'NONE', #1729, #1667, #2621 ) ;
#9213=CARTESIAN_POINT ( 'NONE',  ( 31.77500000054622831, 22.36655054427230027, 98.07665518445361386 ) ) ;
#9215=CARTESIAN_POINT ( 'NONE',  ( 45.67500000054621978, 22.36655054427230027, 98.07665518445361386 ) ) ;
#9216=CARTESIAN_POINT ( 'NONE',  ( 35.87500000054622973, 20.00000000000000355, 98.07665518445361386 ) ) ;
#9217=CARTESIAN_POINT ( 'NONE',  ( 39.09999999999999432, 22.43689772174679575, 83.29316153445363113 ) ) ;
#9219=CARTESIAN_POINT ( 'NONE',  ( 42.87500000054622973, 22.36655054427230382, 83.50966788445364841 ) ) ;
#9221=AXIS2_PLACEMENT_3D ( 'NONE', #11785, #10898, #7024 ) ;
#9222=CARTESIAN_POINT ( 'NONE',  ( 24.75000000109246656, 22.43689772174679575, 83.29316153445363113 ) ) ;
#9224=VERTEX_POINT ( 'NONE', #6545 ) ;
#9229=EDGE_CURVE ( 'NONE', #5525, #4126, #10895, .T. ) ;
#9231=CIRCLE ( 'NONE', #5784, 7.499999999999992895 ) ;
#9233=CARTESIAN_POINT ( 'NONE',  ( 22.17500000054622689, 13.07298590277314254, 93.04388485072563242 ) ) ;
#9234=CARTESIAN_POINT ( 'NONE',  ( 23.47500000054622404, 26.92701409722686634, 93.04388485072563242 ) ) ;
#9236=FACE_OUTER_BOUND ( 'NONE', #7990, .T. ) ;
#9239=CARTESIAN_POINT ( 'NONE',  ( 41.45000000109246940, 24.40838939219354842, 96.86078899226572503 ) ) ;
#9241=ORIENTED_EDGE ( 'NONE', *, *, #5764, .T. ) ;
#9242=CARTESIAN_POINT ( 'NONE',  ( 47.19999999999998863, 24.40838939219355197, 84.72553407664153724 ) ) ;
#9243=ORIENTED_EDGE ( 'NONE', *, *, #939, .T. ) ;
#9247=CARTESIAN_POINT ( 'NONE',  ( -6.999999999999999112, 77.00000000000000000, 101.8533255156881978 ) ) ;
#9250=VECTOR ( 'NONE', #2442, 1000.000000000000000 ) ;
#9253=CARTESIAN_POINT ( 'NONE',  ( 42.99999999999999289, 20.00000000000000355, 83.29316153445364534 ) ) ;
#9255=CARTESIAN_POINT ( 'NONE',  ( -50.00000000000001421, 40.00000000000000000, 132.8533255156884820 ) ) ;
#9257=CARTESIAN_POINT ( 'NONE',  ( 46.95000000109246230, 26.37988106264029398, 86.15790661882942914 ) ) ;
#9259=ADVANCED_FACE ( 'NONE', ( #10660 ), #3056, .F. ) ;
#9261=CARTESIAN_POINT ( 'NONE',  ( 49.99999999999998579, 20.00000000000000355, 83.29316153445363113 ) ) ;
#9263=CARTESIAN_POINT ( 'NONE',  ( 41.27500000054622120, 26.92701409722686634, 88.54243821818162985 ) ) ;
#9265=CARTESIAN_POINT ( 'NONE',  ( 27.17500000054622689, 26.92701409722686634, 88.54243821818162985 ) ) ;
#9266=CARTESIAN_POINT ( 'NONE',  ( 9.237585187503595918, 16.16340832531784244, 84.34413360981309893 ) ) ;
#9267=CARTESIAN_POINT ( 'NONE',  ( 44.65000000109246514, 20.00000000000000355, 83.29316153445364534 ) ) ;
#9270=VERTEX_POINT ( 'NONE', #1971 ) ;
#9275=CARTESIAN_POINT ( 'NONE',  ( 33.77500000054622831, 22.36655054427230027, 98.07665518445361386 ) ) ;
#9277=CARTESIAN_POINT ( 'NONE',  ( 44.47500000054622404, 13.80429023900056684, 86.29171490190961435 ) ) ;
#9278=CARTESIAN_POINT ( 'NONE',  ( 33.07500000054622546, 24.28113015263587471, 84.90069139318163138 ) ) ;
#9279=CARTESIAN_POINT ( 'NONE',  ( 33.29999999999999005, 26.37988106264029398, 86.15790661882942914 ) ) ;
#9282=CARTESIAN_POINT ( 'NONE',  ( 39.67500000054623399, 22.36655054427230027, 98.07665518445361386 ) ) ;
#9283=ORIENTED_EDGE ( 'NONE', *, *, #5764, .F. ) ;
#9284=CARTESIAN_POINT ( 'NONE',  ( 23.95000000109246585, 13.62011893735971135, 95.42841645007781892 ) ) ;
#9286=EDGE_LOOP ( 'NONE', ( #6483, #2439, #5484, #4452 ) ) ;
#9288=EDGE_LOOP ( 'NONE', ( #5103, #7340 ) ) ;
#9289=DIRECTION ( 'NONE',  ( 0.000000000000000000, 0.000000000000000000, -1.000000000000000000 ) ) ;
#9294=EDGE_CURVE ( 'NONE', #2160, #8662, #10595, .T. ) ;
#9295=CARTESIAN_POINT ( 'NONE',  ( 21.87500000054622973, 17.63344945572769973, 98.07665518445361386 ) ) ;
#9296=CARTESIAN_POINT ( 'NONE',  ( 22.97500000054622049, 22.36655054427230382, 83.50966788445364841 ) ) ;
#9297=DIRECTION ( 'NONE',  ( 1.000000000000000000, -0.000000000000000000, -0.000000000000000000 ) ) ;
#9301=CARTESIAN_POINT ( 'NONE',  ( 46.15000000109246514, 12.11403331821300533, 90.79316153445363113 ) ) ;
#9304=FACE_OUTER_BOUND ( 'NONE', #532, .T. ) ;
#9311=VECTOR ( 'NONE', #6498, 1000.000000000000000 ) ;
#9313=CARTESIAN_POINT ( 'NONE',  ( 38.15000000109245804, 12.11403331821300533, 90.79316153445363113 ) ) ;
#9316=ADVANCED_FACE ( 'NONE', ( #11559 ), #4002, .F. ) ;
#9317=DIRECTION ( 'NONE',  ( -1.000000000000000000, 0.000000000000000000, 0.000000000000000000 ) ) ;
#9319=AXIS2_PLACEMENT_3D ( 'NONE', #12485, #7543, #1703 ) ;
#9325=CARTESIAN_POINT ( 'NONE',  ( 38.17500000054622689, 13.80429023900056507, 95.29460816699764791 ) ) ;
#9326=CARTESIAN_POINT ( 'NONE',  ( 26.07500000054622546, 13.80429023900056507, 95.29460816699764791 ) ) ;
#9327=CARTESIAN_POINT ( 'NONE',  ( 8.250161558006810836, 14.33538267060655436, 85.85517769022618495 ) ) ;
#9330=DIRECTION ( 'NONE',  ( 0.000000000000000000, 0.000000000000000000, -1.000000000000000000 ) ) ;
#9332=ORIENTED_EDGE ( 'NONE', *, *, #12502, .T. ) ;
#9335=DIRECTION ( 'NONE',  ( -0.4999999999999892308, -0.000000000000000000, 0.8660254037844448138 ) ) ;
#9337=( BOUNDED_CURVE ( )  B_SPLINE_CURVE ( 2, ( #1930, #9936, #11708, #3075, #2122, #6818, #167, #2955, #1243, #10682, #3013 ),
 .UNSPECIFIED., .F., .F. ) 
 B_SPLINE_CURVE_WITH_KNOTS ( ( 3, 2, 2, 2, 2, 3 ),
 ( 0.1666666666666665741, 0.1733333333333332560, 0.1799999999999999101, 0.1866666666666665919, 0.1933333333333332460, 0.1999999999999999278 ),
 .UNSPECIFIED. ) 
 CURVE ( )  GEOMETRIC_REPRESENTATION_ITEM ( )  RATIONAL_B_SPLINE_CURVE ( ( 1.000000000000000666, 0.9510565162951529761, 1.000000000000000000, 0.9510565162951535312, 1.000000000000000000, 0.9510565162951535312, 1.000000000000000000, 0.9510565162951535312, 1.000000000000000000, 0.9510565162951540863, 0.9999999999999994449 ) ) 
 REPRESENTATION_ITEM ( '' )  );
#9338=CARTESIAN_POINT ( 'NONE',  ( 32.87500000054622262, 20.00000000000000355, 83.50966788445364841 ) ) ;
#9339=CARTESIAN_POINT ( 'NONE',  ( 28.95000000109246585, 26.37988106264029398, 86.15790661882942914 ) ) ;
#9340=CARTESIAN_POINT ( 'NONE',  ( 48.97500000054622404, 24.28113015263587471, 84.90069139318163138 ) ) ;
#9341=CARTESIAN_POINT ( 'NONE',  ( 33.67500000054622689, 24.28113015263587116, 96.68563167572563088 ) ) ;
#9342=CARTESIAN_POINT ( 'NONE',  ( 35.39999999999998437, 27.13292387221364876, 88.47553407664153724 ) ) ;
#9343=CIRCLE ( 'NONE', #3860, 7.500000000000000000 ) ;
#9345=CARTESIAN_POINT ( 'NONE',  ( 39.97500000054622404, 15.71886984736413417, 96.68563167572563088 ) ) ;
#9346=EDGE_LOOP ( 'NONE', ( #10281, #1476, #1869, #1663, #10813, #6753, #4879, #6807, #1315, #3229, #11554 ) ) ;
#9347=CARTESIAN_POINT ( 'NONE',  ( 20.95000000109246230, 26.37988106264029398, 86.15790661882942914 ) ) ;
#9348=CARTESIAN_POINT ( 'NONE',  ( 28.25000000109246301, 12.86707612778636012, 88.47553407664152303 ) ) ;
#9352=VERTEX_POINT ( 'NONE', #1396 ) ;
#9359=CARTESIAN_POINT ( 'NONE',  ( 24.87500000054622618, 22.36655054427230382, 83.50966788445364841 ) ) ;
#9360=CARTESIAN_POINT ( 'NONE',  ( 27.97500000054622404, 17.63344945572769973, 98.07665518445361386 ) ) ;
#9362=DIRECTION ( 'NONE',  ( 1.000000000000000000, 0.000000000000000000, -0.000000000000000000 ) ) ;
#9364=CARTESIAN_POINT ( 'NONE',  ( 39.95000000109245519, 13.62011893735971135, 95.42841645007781892 ) ) ;
#9367=LINE ( 'NONE', #8409, #3829 ) ;
#9374=CARTESIAN_POINT ( 'NONE',  ( 27.99999999999998579, 20.00000000000000355, 98.29316153445363113 ) ) ;
#9376=CARTESIAN_POINT ( 'NONE',  ( 47.65000000109246514, 20.00000000000000355, 98.29316153445363113 ) ) ;
#9377=CARTESIAN_POINT ( 'NONE',  ( 29.47500000054622404, 26.19570976099943493, 95.29460816699764791 ) ) ;
#9380=ORIENTED_EDGE ( 'NONE', *, *, #7218, .T. ) ;
#9384=CARTESIAN_POINT ( 'NONE',  ( 36.07500000054622546, 13.80429023900056507, 95.29460816699764791 ) ) ;
#9385=CARTESIAN_POINT ( 'NONE',  ( 36.87500000054622262, 20.00000000000000355, 83.50966788445364841 ) ) ;
#9386=CARTESIAN_POINT ( 'NONE',  ( 26.97500000054622760, 24.28113015263587471, 84.90069139318163138 ) ) ;
#9392=VERTEX_POINT ( 'NONE', #7471 ) ;
#9396=CARTESIAN_POINT ( 'NONE',  ( 31.57500000054622191, 26.19570976099943849, 95.29460816699764791 ) ) ;
#9397=CARTESIAN_POINT ( 'NONE',  ( 42.99999999999999289, 20.00000000000000355, 83.29316153445364534 ) ) ;
#9399=CARTESIAN_POINT ( 'NONE',  ( 48.67500000054623399, 17.63344945572770328, 83.50966788445364841 ) ) ;
#9400=CARTESIAN_POINT ( 'NONE',  ( 35.47500000054622404, 26.92701409722686634, 93.04388485072563242 ) ) ;
#9401=CARTESIAN_POINT ( 'NONE',  ( 29.39999999999998792, 27.13292387221364876, 88.47553407664153724 ) ) ;
#9404=CARTESIAN_POINT ( 'NONE',  ( 38.07500000054623257, 13.80429023900056507, 95.29460816699764791 ) ) ;
#9405=EDGE_LOOP ( 'NONE', ( #2627, #6885, #40, #1619 ) ) ;
#9406=AXIS2_PLACEMENT_3D ( 'NONE', #8026, #4085, #3136 ) ;
#9407=CARTESIAN_POINT ( 'NONE',  ( 19.75000000109246301, 17.56310227825320425, 98.29316153445363113 ) ) ;
#9409=ORIENTED_EDGE ( 'NONE', *, *, #2844, .F. ) ;
#9413=( BOUNDED_CURVE ( )  B_SPLINE_CURVE ( 2, ( #3582, #4790, #3767, #3703, #3833, #11329, #9493, #5621, #12404, #7584, #4663 ),
 .UNSPECIFIED., .F., .F. ) 
 B_SPLINE_CURVE_WITH_KNOTS ( ( 3, 2, 2, 2, 2, 3 ),
 ( 0.5999999999999999778, 0.6066666666666666874, 0.6133333333333332860, 0.6199999999999999956, 0.6266666666666667052, 0.6333333333333333037 ),
 .UNSPECIFIED. ) 
 CURVE ( )  GEOMETRIC_REPRESENTATION_ITEM ( )  RATIONAL_B_SPLINE_CURVE ( ( 1.000000000000000000, 0.9510565162951535312, 1.000000000000000000, 0.9510565162951535312, 1.000000000000000000, 0.9510565162951535312, 1.000000000000000000, 0.9510565162951535312, 1.000000000000000000, 0.9510565162951535312, 1.000000000000000000 ) ) 
 REPRESENTATION_ITEM ( '' )  );
#9414=EDGE_CURVE ( 'NONE', #11966, #4281, #9661, .T. ) ;
#9416=LINE ( 'NONE', #12265, #3836 ) ;
#9419=CARTESIAN_POINT ( 'NONE',  ( 25.37500000054622973, 26.92701409722686634, 93.04388485072563242 ) ) ;
#9420=CARTESIAN_POINT ( 'NONE',  ( 21.27500000054622475, 26.92701409722686634, 88.54243821818162985 ) ) ;
#9423=CARTESIAN_POINT ( 'NONE',  ( -50.00000000000001421, 40.00000000000000000, 121.2488769092545198 ) ) ;
#9425=CARTESIAN_POINT ( 'NONE',  ( 35.15000000109247225, 27.88596668178699645, 90.79316153445363113 ) ) ;
#9426=CARTESIAN_POINT ( 'NONE',  ( 24.29999999999999005, 13.62011893735970958, 95.42841645007781892 ) ) ;
#9432=VECTOR ( 'NONE', #11838, 1000.000000000000000 ) ;
#9438=CARTESIAN_POINT ( 'NONE',  ( 49.67500000054622689, 24.28113015263587116, 96.68563167572563088 ) ) ;
#9440=CARTESIAN_POINT ( 'NONE',  ( 46.75000000109247367, 22.43689772174677088, 83.29316153445361692 ) ) ;
#9442=VERTEX_POINT ( 'NONE', #1576 ) ;
#9443=VECTOR ( 'NONE', #6697, 1000.000000000000000 ) ;
#9447=CARTESIAN_POINT ( 'NONE',  ( 38.47500000054622404, 13.07298590277314432, 88.54243821818161564 ) ) ;
#9448=CARTESIAN_POINT ( 'NONE',  ( 23.57500000054622902, 24.28113015263587116, 96.68563167572563088 ) ) ;
#9454=ADVANCED_FACE ( 'NONE', ( #12172 ), #5388, .T. ) ;
#9457=( BOUNDED_CURVE ( )  B_SPLINE_CURVE ( 2, ( #8784, #37, #9745, #7839, #10681, #10616, #3898, #7776, #2954, #1992, #103 ),
 .UNSPECIFIED., .F., .F. ) 
 B_SPLINE_CURVE_WITH_KNOTS ( ( 3, 2, 2, 2, 2, 3 ),
 ( 0.4666666666666666186, 0.4733333333333332726, 0.4799999999999999267, 0.4866666666666666918, 0.4933333333333333459, 0.5000000000000000000 ),
 .UNSPECIFIED. ) 
 CURVE ( )  GEOMETRIC_REPRESENTATION_ITEM ( )  RATIONAL_B_SPLINE_CURVE ( ( 1.000000000000000444, 0.9510565162951531981, 1.000000000000000000, 0.9510565162951535312, 1.000000000000000000, 0.9510565162951535312, 1.000000000000000000, 0.9510565162951535312, 1.000000000000000000, 0.9510565162951535312, 1.000000000000000000 ) ) 
 REPRESENTATION_ITEM ( '' )  );
#9458=DIRECTION ( 'NONE',  ( 0.000000000000000000, 0.000000000000000000, -1.000000000000000000 ) ) ;
#9461=CARTESIAN_POINT ( 'NONE',  ( 26.27500000054622475, 13.07298590277314254, 93.04388485072563242 ) ) ;
#9463=CARTESIAN_POINT ( 'NONE',  ( 39.97500000054622404, 15.71886984736413417, 96.68563167572563088 ) ) ;
#9464=CARTESIAN_POINT ( 'NONE',  ( 29.07500000054622191, 24.28113015263587471, 84.90069139318163138 ) ) ;
#9465=CARTESIAN_POINT ( 'NONE',  ( 32.89999999999998437, 17.56310227825321135, 83.29316153445363113 ) ) ;
#9466=CARTESIAN_POINT ( 'NONE',  ( 30.39999999999998792, 12.86707612778636012, 93.11078899226572503 ) ) ;
#9467=CARTESIAN_POINT ( 'NONE',  ( 40.57500000054623257, 15.71886984736413773, 84.90069139318163138 ) ) ;
#9468=ORIENTED_EDGE ( 'NONE', *, *, #1189, .F. ) ;
#9470=CARTESIAN_POINT ( 'NONE',  ( 47.17500000054623399, 26.92701409722686634, 88.54243821818162985 ) ) ;
#9473=DIRECTION ( 'NONE',  ( 1.000000000000000000, -0.000000000000000000, -0.000000000000000000 ) ) ;
#9476=CARTESIAN_POINT ( 'NONE',  ( 43.09999999999998721, 22.43689772174680641, 83.29316153445363113 ) ) ;
#9479=CARTESIAN_POINT ( 'NONE',  ( 42.67500000054622689, 15.71886984736413773, 84.90069139318163138 ) ) ;
#9482=CARTESIAN_POINT ( 'NONE',  ( 47.59999999999998721, 27.13292387221364876, 93.11078899226573924 ) ) ;
#9486=VERTEX_POINT ( 'NONE', #9196 ) ;
#9487=CARTESIAN_POINT ( 'NONE',  ( 38.85000000109246798, 24.40838939219355197, 84.72553407664153724 ) ) ;
#9490=VERTEX_POINT ( 'NONE', #8242 ) ;
#9492=ADVANCED_FACE ( 'NONE', ( #7406 ), #3414, .F. ) ;
#9493=CARTESIAN_POINT ( 'NONE',  ( 31.05000000109246372, 27.13292387221364876, 88.47553407664153724 ) ) ;
#9499=CARTESIAN_POINT ( 'NONE',  ( 42.65000000109246514, 20.00000000000000355, 83.29316153445364534 ) ) ;
#9500=CARTESIAN_POINT ( 'NONE',  ( 48.55000000109247082, 17.56310227825320069, 83.29316153445363113 ) ) ;
#9501=CARTESIAN_POINT ( 'NONE',  ( 48.67500000054622689, 15.71886984736413773, 84.90069139318163138 ) ) ;
#9502=CARTESIAN_POINT ( 'NONE',  ( -27.49999999999999645, 27.49999999999999645, 145.0000000000000000 ) ) ;
#9503=CARTESIAN_POINT ( 'NONE',  ( 27.50000000000000355, 12.50000000000001066, 145.0000000000000000 ) ) ;
#9504=VERTEX_POINT ( 'NONE', #9261 ) ;
#9506=ORIENTED_EDGE ( 'NONE', *, *, #482, .T. ) ;
#9508=CARTESIAN_POINT ( 'NONE',  ( -50.00000000000001421, 20.00000000000000000, 145.0000000000000000 ) ) ;
#9510=CARTESIAN_POINT ( 'NONE',  ( 39.67500000054622689, 24.28113015263587116, 96.68563167572563088 ) ) ;
#9511=CARTESIAN_POINT ( 'NONE',  ( 21.67500000054622689, 22.36655054427230027, 98.07665518445361386 ) ) ;
#9523=CARTESIAN_POINT ( 'NONE',  ( 24.37500000054621907, 12.34168156654572357, 90.79316153445363113 ) ) ;
#9524=CARTESIAN_POINT ( 'NONE',  ( 36.59999999999998721, 12.86707612778636012, 88.47553407664152303 ) ) ;
#9525=CARTESIAN_POINT ( 'NONE',  ( 39.47500000054622404, 26.19570976099943849, 95.29460816699764791 ) ) ;
#9526=CARTESIAN_POINT ( 'NONE',  ( 29.47500000054622404, 26.92701409722686634, 93.04388485072563242 ) ) ;
#9527=CARTESIAN_POINT ( 'NONE',  ( 27.79999999999998650, 24.40838939219354842, 96.86078899226572503 ) ) ;
#9529=CARTESIAN_POINT ( 'NONE',  ( 41.07500000054622546, 26.19570976099943493, 86.29171490190961435 ) ) ;
#9532=CARTESIAN_POINT ( 'NONE',  ( 48.47500000054623115, 13.80429023900056684, 86.29171490190961435 ) ) ;
#9534=ORIENTED_EDGE ( 'NONE', *, *, #1944, .F. ) ;
#9541=CARTESIAN_POINT ( 'NONE',  ( 42.17500000054622689, 13.80429023900056507, 95.29460816699764791 ) ) ;
#9543=EDGE_CURVE ( 'NONE', #9504, #11262, #6814, .T. ) ;
#9545=CARTESIAN_POINT ( 'NONE',  ( 47.27500000054622831, 26.92701409722686634, 88.54243821818162985 ) ) ;
#9546=CARTESIAN_POINT ( 'NONE',  ( 21.77500000054622831, 22.36655054427230027, 98.07665518445361386 ) ) ;
#9548=CARTESIAN_POINT ( 'NONE',  ( 39.15000000109246514, 27.88596668178699645, 90.79316153445363113 ) ) ;
#9550=CARTESIAN_POINT ( 'NONE',  ( 38.95000000109246940, 26.37988106264029398, 86.15790661882942914 ) ) ;
#9554=CARTESIAN_POINT ( 'NONE',  ( 19.82500000054622546, 20.00000000000000355, 98.07665518445361386 ) ) ;
#9557=CARTESIAN_POINT ( 'NONE',  ( -36.00000000000001421, 77.00000000000000000, 104.8533255156881836 ) ) ;
#9561=ADVANCED_FACE ( 'NONE', ( #10630 ), #12418, .F. ) ;
#9563=CARTESIAN_POINT ( 'NONE',  ( 22.37500000054622973, 13.07298590277314432, 88.54243821818161564 ) ) ;
#9564=CARTESIAN_POINT ( 'NONE',  ( 46.15000000109246514, 12.11403331821300533, 90.79316153445363113 ) ) ;
#9568=EDGE_CURVE ( 'NONE', #5882, #12216, #12406, .T. ) ;
#9571=CARTESIAN_POINT ( 'NONE',  ( 10.00000000000001421, 20.25634836214397794, 98.29316153445363113 ) ) ;
#9574=CARTESIAN_POINT ( 'NONE',  ( -111.8465843842649292, 84.49999999999998579, 146.8533255156881978 ) ) ;
#9580=CARTESIAN_POINT ( 'NONE',  ( 26.97500000054622049, 22.36655054427230382, 83.50966788445364841 ) ) ;
#9581=CARTESIAN_POINT ( 'NONE',  ( 49.65000000109246514, 20.00000000000000355, 98.29316153445363113 ) ) ;
#9583=CARTESIAN_POINT ( 'NONE',  ( 38.87500000054622973, 22.36655054427230382, 83.50966788445364841 ) ) ;
#9584=CARTESIAN_POINT ( 'NONE',  ( 24.87500000054622262, 20.00000000000000355, 83.50966788445364841 ) ) ;
#9585=CARTESIAN_POINT ( 'NONE',  ( 31.89999999999998437, 22.43689772174679575, 98.29316153445363113 ) ) ;
#9587=CARTESIAN_POINT ( 'NONE',  ( 34.87500000054623683, 22.36655054427230382, 83.50966788445364841 ) ) ;
#9589=CARTESIAN_POINT ( 'NONE',  ( 43.97500000054623115, 15.71886984736413417, 96.68563167572563088 ) ) ;
#9590=CARTESIAN_POINT ( 'NONE',  ( 27.65000000109246514, 20.00000000000000355, 98.29316153445363113 ) ) ;
#9596=CARTESIAN_POINT ( 'NONE',  ( 32.99999999999998579, 20.00000000000000355, 83.29316153445364534 ) ) ;
#9598=CARTESIAN_POINT ( 'NONE',  ( 46.57500000054622546, 13.80429023900056684, 86.29171490190961435 ) ) ;
#9599=CYLINDRICAL_SURFACE ( 'NONE', #12433, 7.499999999999978684 ) ;
#9601=CARTESIAN_POINT ( 'NONE',  ( 47.99999999999998579, 20.00000000000000355, 98.29316153445363113 ) ) ;
#9603=CYLINDRICAL_SURFACE ( 'NONE', #1308, 7.499999999999992895 ) ;
#9604=CARTESIAN_POINT ( 'NONE',  ( -27.49999999999999645, 12.50000000000001066, 145.0000000000000000 ) ) ;
#9606=CIRCLE ( 'NONE', #10408, 7.500000000000000000 ) ;
#9608=CARTESIAN_POINT ( 'NONE',  ( 38.75000000109245946, 22.43689772174679575, 83.29316153445363113 ) ) ;
#9610=EDGE_LOOP ( 'NONE', ( #2027, #7230, #2267, #11775 ) ) ;
#9615=AXIS2_PLACEMENT_3D ( 'NONE', #1571, #4362, #7147 ) ;
#9618=EDGE_CURVE ( 'NONE', #1942, #10754, #2437, .T. ) ;
#9619=CARTESIAN_POINT ( 'NONE',  ( 36.67500000054623399, 17.63344945572770328, 83.50966788445364841 ) ) ;
#9623=FACE_OUTER_BOUND ( 'NONE', #9346, .T. ) ;
#9625=CARTESIAN_POINT ( 'NONE',  ( 22.57500000054622902, 15.71886984736413773, 84.90069139318163138 ) ) ;
#9627=CARTESIAN_POINT ( 'NONE',  ( -27.49999999999999645, 27.49999999999999645, 145.0000000000000000 ) ) ;
#9629=ORIENTED_EDGE ( 'NONE', *, *, #7190, .T. ) ;
#9635=DIRECTION ( 'NONE',  ( -1.000000000000000000, -0.000000000000000000, -0.000000000000000000 ) ) ;
#9636=CARTESIAN_POINT ( 'NONE',  ( 48.99999999999998579, 20.00000000000000355, 83.29316153445364534 ) ) ;
#9637=CARTESIAN_POINT ( 'NONE',  ( -28.50000000000001066, 84.49999999999998579, 146.8533255156881978 ) ) ;
#9647=CARTESIAN_POINT ( 'NONE',  ( 25.67500000054622333, 24.28113015263587116, 96.68563167572563088 ) ) ;
#9648=CARTESIAN_POINT ( 'NONE',  ( 47.77500000054622120, 22.36655054427230027, 98.07665518445361386 ) ) ;
#9649=AXIS2_PLACEMENT_3D ( 'NONE', #3815, #2802, #6793 ) ;
#9650=CARTESIAN_POINT ( 'NONE',  ( 38.47500000054621694, 13.80429023900056684, 86.29171490190961435 ) ) ;
#9651=CARTESIAN_POINT ( 'NONE',  ( 27.07500000054622546, 24.28113015263587471, 84.90069139318163138 ) ) ;
#9652=CARTESIAN_POINT ( 'NONE',  ( 28.49999999999998934, 12.11403331821300533, 90.79316153445363113 ) ) ;
#9654=CARTESIAN_POINT ( 'NONE',  ( 34.59999999999999432, 12.86707612778636012, 88.47553407664152303 ) ) ;
#9655=CARTESIAN_POINT ( 'NONE',  ( 35.37500000054622973, 26.92701409722686634, 93.04388485072563242 ) ) ;
#9661=CIRCLE ( 'NONE', #2771, 7.500000000000000000 ) ;
#9663=DIRECTION ( 'NONE',  ( 0.000000000000000000, 0.000000000000000000, -1.000000000000000000 ) ) ;
#9664=CARTESIAN_POINT ( 'NONE',  ( 44.07500000054622546, 15.71886984736413417, 96.68563167572563088 ) ) ;
#9665=CARTESIAN_POINT ( 'NONE',  ( -50.00000000000001421, 0.000000000000000000, 69.99999999999998579 ) ) ;
#9666=CARTESIAN_POINT ( 'NONE',  ( 44.37500000054622262, 12.34168156654572535, 90.79316153445363113 ) ) ;
#9667=CARTESIAN_POINT ( 'NONE',  ( 48.59999999999998721, 12.86707612778636012, 88.47553407664152303 ) ) ;
#9668=VECTOR ( 'NONE', #10695, 1000.000000000000000 ) ;
#9672=CARTESIAN_POINT ( 'NONE',  ( 29.75000000109245946, 17.56310227825320425, 98.29316153445363113 ) ) ;
#9681=CARTESIAN_POINT ( 'NONE',  ( 39.27500000054622120, 27.65831843345427998, 90.79316153445363113 ) ) ;
#9684=FACE_OUTER_BOUND ( 'NONE', #11652, .T. ) ;
#9688=CARTESIAN_POINT ( 'NONE',  ( 47.87500000054622262, 20.00000000000000355, 98.07665518445361386 ) ) ;
#9689=ORIENTED_EDGE ( 'NONE', *, *, #6277, .T. ) ;
#9690=CARTESIAN_POINT ( 'NONE',  ( 46.45000000109246230, 15.59161060780646046, 84.72553407664153724 ) ) ;
#9691=CARTESIAN_POINT ( 'NONE',  ( -5.000000000000000888, -3.000000000000002665, 121.2488769092545198 ) ) ;
#9694=AXIS2_PLACEMENT_3D ( 'NONE', #2597, #4625, #10331 ) ;
#9695=CARTESIAN_POINT ( 'NONE',  ( 21.99999999999998934, 20.00000000000000355, 98.29316153445363113 ) ) ;
#9696=EDGE_CURVE ( 'NONE', #7152, #5818, #4931, .T. ) ;
#9697=CARTESIAN_POINT ( 'NONE',  ( 21.47500000054622760, 26.19570976099943849, 95.29460816699764791 ) ) ;
#9699=CARTESIAN_POINT ( 'NONE',  ( 0.000000000000000000, 31.99999999999960565, 124.8533255156881694 ) ) ;
#9704=EDGE_LOOP ( 'NONE', ( #915, #2291, #9988, #3619 ) ) ;
#9707=EDGE_CURVE ( 'NONE', #707, #9442, #11719, .T. ) ;
#9708=CARTESIAN_POINT ( 'NONE',  ( 20.87500000054622262, 20.00000000000000355, 83.50966788445364841 ) ) ;
#9710=CARTESIAN_POINT ( 'NONE',  ( 40.07500000054623257, 13.80429023900056507, 95.29460816699764791 ) ) ;
#9712=CARTESIAN_POINT ( 'NONE',  ( 27.87500000054622262, 20.00000000000000355, 98.07665518445361386 ) ) ;
#9713=CARTESIAN_POINT ( 'NONE',  ( 22.69999999999998153, 13.62011893735971135, 86.15790661882942914 ) ) ;
#9715=CARTESIAN_POINT ( 'NONE',  ( 33.77500000054622831, 20.00000000000000355, 98.07665518445361386 ) ) ;
#9721=ORIENTED_EDGE ( 'NONE', *, *, #9835, .F. ) ;
#9722=CARTESIAN_POINT ( 'NONE',  ( 43.59999999999998721, 27.13292387221364876, 93.11078899226573924 ) ) ;
#9725=CARTESIAN_POINT ( 'NONE',  ( 46.67500000054622689, 15.71886984736413773, 84.90069139318163138 ) ) ;
#9728=CARTESIAN_POINT ( 'NONE',  ( 43.87500000054622973, 20.00000000000000355, 98.07665518445361386 ) ) ;
#9729=CARTESIAN_POINT ( 'NONE',  ( 43.49999999999998579, 27.88596668178699645, 90.79316153445363113 ) ) ;
#9731=CARTESIAN_POINT ( 'NONE',  ( 45.49999999999997868, 27.88596668178699645, 90.79316153445363113 ) ) ;
#9732=CARTESIAN_POINT ( 'NONE',  ( 4.999999999999997335, 40.00000000000000000, 69.99999999999998579 ) ) ;
#9733=ORIENTED_EDGE ( 'NONE', *, *, #525, .F. ) ;
#9734=CARTESIAN_POINT ( 'NONE',  ( 32.55000000109247082, 17.56310227825321135, 83.29316153445363113 ) ) ;
#9736=VERTEX_POINT ( 'NONE', #8862 ) ;
#9738=VECTOR ( 'NONE', #2988, 1000.000000000000000 ) ;
#9741=LINE ( 'NONE', #2119, #3925 ) ;
#9742=( BOUNDED_CURVE ( )  B_SPLINE_CURVE ( 2, ( #9374, #4542, #12469, #12287, #7589, #1625, #1807, #8661, #5750, #4796, #3587 ),
 .UNSPECIFIED., .F., .F. ) 
 B_SPLINE_CURVE_WITH_KNOTS ( ( 3, 2, 2, 2, 2, 3 ),
 ( 0.7333333333333332815, 0.7399999999999999911, 0.7466666666666667007, 0.7533333333333331883, 0.7599999999999998979, 0.7666666666666666075 ),
 .UNSPECIFIED. ) 
 CURVE ( )  GEOMETRIC_REPRESENTATION_ITEM ( )  RATIONAL_B_SPLINE_CURVE ( ( 1.000000000000000000, 0.9510565162951535312, 1.000000000000000000, 0.9510565162951535312, 1.000000000000000000, 0.9510565162951535312, 1.000000000000000000, 0.9510565162951535312, 1.000000000000000000, 0.9510565162951543083, 0.9999999999999992228 ) ) 
 REPRESENTATION_ITEM ( '' )  );
#9743=CARTESIAN_POINT ( 'NONE',  ( 40.07500000054623257, 13.80429023900056507, 95.29460816699764791 ) ) ;
#9744=CARTESIAN_POINT ( 'NONE',  ( 37.27500000054622831, 26.92701409722686634, 88.54243821818162985 ) ) ;
#9745=CARTESIAN_POINT ( 'NONE',  ( 35.45000000109246940, 24.40838939219354842, 96.86078899226572503 ) ) ;
#9747=CARTESIAN_POINT ( 'NONE',  ( 35.00000000000000000, 24.39339828220178674, 137.5000000000000000 ) ) ;
#9748=ORIENTED_EDGE ( 'NONE', *, *, #4314, .T. ) ;
#9750=CARTESIAN_POINT ( 'NONE',  ( 47.85000000109246088, 15.59161060780645691, 96.86078899226572503 ) ) ;
#9753=CARTESIAN_POINT ( 'NONE',  ( -27.49999999999999645, 20.00000000000000355, 170.0000119999999697 ) ) ;
#9755=ORIENTED_EDGE ( 'NONE', *, *, #720, .F. ) ;
#9760=CARTESIAN_POINT ( 'NONE',  ( 6.688242141207060953, 27.43430974961319535, 89.77032832267597939 ) ) ;
#9761=CARTESIAN_POINT ( 'NONE',  ( 37.69999999999998153, 26.37988106264029398, 95.42841645007781892 ) ) ;
#9764=CARTESIAN_POINT ( 'NONE',  ( -28.50000000000001066, 69.50000000000000000, 146.8533255156881978 ) ) ;
#9765=CARTESIAN_POINT ( 'NONE',  ( -111.8465843842649292, 69.50000000000000000, 146.8533255156881978 ) ) ;
#9770=CARTESIAN_POINT ( 'NONE',  ( 22.97500000054622049, 22.36655054427230382, 83.50966788445364841 ) ) ;
#9771=CARTESIAN_POINT ( 'NONE',  ( 48.57500000054622546, 13.80429023900056684, 86.29171490190961435 ) ) ;
#9773=CARTESIAN_POINT ( 'NONE',  ( 32.37500000054622973, 13.07298590277314432, 88.54243821818161564 ) ) ;
#9775=CARTESIAN_POINT ( 'NONE',  ( 21.59999999999998721, 27.13292387221364876, 93.11078899226573924 ) ) ;
#9776=DIRECTION ( 'NONE',  ( 0.000000000000000000, 0.000000000000000000, -1.000000000000000000 ) ) ;
#9777=CARTESIAN_POINT ( 'NONE',  ( 33.87500000054621552, 17.63344945572769973, 98.07665518445361386 ) ) ;
#9778=EDGE_LOOP ( 'NONE', ( #3984, #12026, #9380, #3623 ) ) ;
#9780=ORIENTED_EDGE ( 'NONE', *, *, #4697, .F. ) ;
#9782=EDGE_LOOP ( 'NONE', ( #4765, #6378, #2237, #9409 ) ) ;
#9784=CARTESIAN_POINT ( 'NONE',  ( -21.00000000000001066, 77.00000000000000000, 104.8533255156881836 ) ) ;
#9786=CARTESIAN_POINT ( 'NONE',  ( 36.77500000054622831, 17.63344945572770328, 83.50966788445364841 ) ) ;
#9790=CARTESIAN_POINT ( 'NONE',  ( 37.27500000054622831, 26.92701409722686634, 88.54243821818162985 ) ) ;
#9791=CARTESIAN_POINT ( 'NONE',  ( 39.59999999999998721, 27.13292387221364876, 93.11078899226573924 ) ) ;
#9792=CARTESIAN_POINT ( 'NONE',  ( -5.000000000000000888, -3.000000000000002665, 121.2488769092545198 ) ) ;
#9794=ORIENTED_EDGE ( 'NONE', *, *, #10084, .F. ) ;
#9796=VECTOR ( 'NONE', #10899, 1000.000000000000000 ) ;
#9797=CARTESIAN_POINT ( 'NONE',  ( 28.25000000109246301, 12.86707612778636012, 88.47553407664152303 ) ) ;
#9799=VERTEX_POINT ( 'NONE', #2207 ) ;
#9806=CARTESIAN_POINT ( 'NONE',  ( 35.67500000054623399, 22.36655054427230027, 98.07665518445361386 ) ) ;
#9807=CARTESIAN_POINT ( 'NONE',  ( 30.77500000054621765, 17.63344945572770328, 83.50966788445364841 ) ) ;
#9811=CARTESIAN_POINT ( 'NONE',  ( -10.00000000000000355, 20.00000000000000355, 69.99999999999998579 ) ) ;
#9812=VERTEX_POINT ( 'NONE', #3219 ) ;
#9817=ORIENTED_EDGE ( 'NONE', *, *, #11552, .T. ) ;
#9818=AXIS2_PLACEMENT_3D ( 'NONE', #10266, #10324, #9330 ) ;
#9820=( BOUNDED_CURVE ( )  B_SPLINE_CURVE ( 2, ( #2554, #10291, #8152, #1550, #12019, #4219, #5359, #11957, #7253, #11002, #1431 ),
 .UNSPECIFIED., .F., .F. ) 
 B_SPLINE_CURVE_WITH_KNOTS ( ( 3, 2, 2, 2, 2, 3 ),
 ( 0.8000000000000000444, 0.8066666666666666430, 0.8133333333333333526, 0.8199999999999999512, 0.8266666666666666607, 0.8333333333333333703 ),
 .UNSPECIFIED. ) 
 CURVE ( )  GEOMETRIC_REPRESENTATION_ITEM ( )  RATIONAL_B_SPLINE_CURVE ( ( 1.000000000000000000, 0.9510565162951535312, 1.000000000000000000, 0.9510565162951535312, 1.000000000000000000, 0.9510565162951535312, 1.000000000000000000, 0.9510565162951535312, 1.000000000000000000, 0.9510565162951535312, 1.000000000000000000 ) ) 
 REPRESENTATION_ITEM ( '' )  );
#9822=CARTESIAN_POINT ( 'NONE',  ( -5.000000000000000888, 0.000000000000000000, 169.9999999999999716 ) ) ;
#9823=CARTESIAN_POINT ( 'NONE',  ( 9.843890364154358252, 21.77789078299004188, 98.08379766955695800 ) ) ;
#9824=CARTESIAN_POINT ( 'NONE',  ( 36.99999999999999289, 20.00000000000000355, 83.29316153445364534 ) ) ;
#9829=CARTESIAN_POINT ( 'NONE',  ( 43.57500000054623257, 24.28113015263587116, 96.68563167572563088 ) ) ;
#9835=EDGE_CURVE ( 'NONE', #1690, #2848, #5945, .T. ) ;
#9838=CARTESIAN_POINT ( 'NONE',  ( 35.77500000054622831, 20.00000000000000355, 98.07665518445361386 ) ) ;
#9839=CARTESIAN_POINT ( 'NONE',  ( 23.37500000054621907, 27.65831843345427998, 90.79316153445363113 ) ) ;
#9840=CARTESIAN_POINT ( 'NONE',  ( 24.49999999999998934, 12.11403331821300533, 90.79316153445363113 ) ) ;
#9841=CARTESIAN_POINT ( 'NONE',  ( 49.59999999999999432, 27.13292387221364876, 93.11078899226573924 ) ) ;
#9842=CARTESIAN_POINT ( 'NONE',  ( 33.67500000054623399, 22.36655054427230027, 98.07665518445361386 ) ) ;
#9846=ORIENTED_EDGE ( 'NONE', *, *, #5834, .F. ) ;
#9851=CARTESIAN_POINT ( 'NONE',  ( 36.97500000054622404, 22.36655054427230382, 83.50966788445364841 ) ) ;
#9852=FACE_OUTER_BOUND ( 'NONE', #8149, .T. ) ;
#9853=CARTESIAN_POINT ( 'NONE',  ( 49.47500000054621694, 26.19570976099943849, 95.29460816699764791 ) ) ;
#9854=CARTESIAN_POINT ( 'NONE',  ( 41.57500000054622546, 26.19570976099943493, 95.29460816699764791 ) ) ;
#9855=CARTESIAN_POINT ( 'NONE',  ( 42.39999999999998437, 12.86707612778636012, 93.11078899226572503 ) ) ;
#9858=DIRECTION ( 'NONE',  ( -0.000000000000000000, -0.000000000000000000, 1.000000000000000000 ) ) ;
#9859=LINE ( 'NONE', #5862, #5249 ) ;
#9860=ORIENTED_EDGE ( 'NONE', *, *, #10791, .T. ) ;
#9861=CARTESIAN_POINT ( 'NONE',  ( 31.05000000109246372, 27.13292387221364876, 88.47553407664153724 ) ) ;
#9864=EDGE_CURVE ( 'NONE', #652, #12355, #3725, .T. ) ;
#9866=DIRECTION ( 'NONE',  ( 0.000000000000000000, 0.000000000000000000, -1.000000000000000000 ) ) ;
#9868=CARTESIAN_POINT ( 'NONE',  ( -36.00000000000001421, 77.00000000000000000, 154.3533255156881978 ) ) ;
#9869=EDGE_CURVE ( 'NONE', #2004, #2031, #5040, .T. ) ;
#9870=CARTESIAN_POINT ( 'NONE',  ( 31.87500000054622973, 17.63344945572769973, 98.07665518445361386 ) ) ;
#9871=CARTESIAN_POINT ( 'NONE',  ( 32.07500000054622546, 15.71886984736413417, 96.68563167572563088 ) ) ;
#9874=FACE_OUTER_BOUND ( 'NONE', #10530, .T. ) ;
#9877=ORIENTED_EDGE ( 'NONE', *, *, #6134, .T. ) ;
#9878=DIRECTION ( 'NONE',  ( 0.000000000000000000, 1.000000000000000000, 0.000000000000000000 ) ) ;
#9884=UNCERTAINTY_MEASURE_WITH_UNIT (LENGTH_MEASURE( 1.000000000000000082E-05 ), #2929, 'distance_accuracy_value', 'NONE');
#9887=CARTESIAN_POINT ( 'NONE',  ( 27.50000000000000355, 27.49999999999999645, 145.0000000000000000 ) ) ;
#9888=CARTESIAN_POINT ( 'NONE',  ( 49.99999999999998579, 0.000000000000000000, 169.9999999999999716 ) ) ;
#9892=CARTESIAN_POINT ( 'NONE',  ( 40.77500000054622831, 20.00000000000000355, 83.50966788445364841 ) ) ;
#9895=VECTOR ( 'NONE', #1671, 1000.000000000000000 ) ;
#9898=CARTESIAN_POINT ( 'NONE',  ( 23.37500000054621907, 27.65831843345427998, 90.79316153445363113 ) ) ;
#9899=FACE_OUTER_BOUND ( 'NONE', #3873, .T. ) ;
#9900=CARTESIAN_POINT ( 'NONE',  ( 31.97500000054623470, 15.71886984736413417, 96.68563167572563088 ) ) ;
#9903=CARTESIAN_POINT ( 'NONE',  ( 23.29999999999999005, 26.37988106264029398, 86.15790661882942914 ) ) ;
#9905=CARTESIAN_POINT ( 'NONE',  ( 26.27500000054622475, 12.34168156654572535, 90.79316153445363113 ) ) ;
#9906=ORIENTED_EDGE ( 'NONE', *, *, #2513, .F. ) ;
#9907=CARTESIAN_POINT ( 'NONE',  ( 0.000000000000000000, 18.00000000000000355, 169.9999999999999716 ) ) ;
#9914=FACE_BOUND ( 'NONE', #10346, .T. ) ;
#9915=CARTESIAN_POINT ( 'NONE',  ( 36.37500000054622973, 12.34168156654572357, 90.79316153445363113 ) ) ;
#9917=CYLINDRICAL_SURFACE ( 'NONE', #8809, 7.499999999999992895 ) ;
#9918=CARTESIAN_POINT ( 'NONE',  ( 41.37500000054622973, 27.65831843345427998, 90.79316153445363113 ) ) ;
#9919=CARTESIAN_POINT ( 'NONE',  ( 39.49999999999997158, 27.88596668178699645, 90.79316153445363113 ) ) ;
#9920=CARTESIAN_POINT ( 'NONE',  ( 47.57500000054622546, 24.28113015263587116, 96.68563167572563088 ) ) ;
#9921=VECTOR ( 'NONE', #3724, 1000.000000000000000 ) ;
#9922=ORIENTED_EDGE ( 'NONE', *, *, #10633, .F. ) ;
#9923=CARTESIAN_POINT ( 'NONE',  ( 30.35000000109246088, 13.62011893735971135, 86.15790661882942914 ) ) ;
#9928=CARTESIAN_POINT ( 'NONE',  ( -2.000000000000015543, 20.00000000000000355, 90.79316153445363113 ) ) ;
#9929=EDGE_CURVE ( 'NONE', #1996, #5802, #8164, .T. ) ;
#9931=CARTESIAN_POINT ( 'NONE',  ( -2.000000000000015543, 20.00000000000000355, 98.29316153445363113 ) ) ;
#9933=CARTESIAN_POINT ( 'NONE',  ( 29.37500000054622973, 26.92701409722686634, 93.04388485072563242 ) ) ;
#9934=CARTESIAN_POINT ( 'NONE',  ( 29.57500000054621836, 26.19570976099943493, 95.29460816699764791 ) ) ;
#9936=CARTESIAN_POINT ( 'NONE',  ( 44.55000000109245661, 17.56310227825322912, 83.29316153445361692 ) ) ;
#9939=CARTESIAN_POINT ( 'NONE',  ( 47.77500000054622120, 22.36655054427230027, 98.07665518445361386 ) ) ;
#9940=CARTESIAN_POINT ( 'NONE',  ( 49.15000000109245804, 27.88596668178699645, 90.79316153445363113 ) ) ;
#9942=CARTESIAN_POINT ( 'NONE',  ( 30.55000000109246372, 17.56310227825320425, 83.29316153445363113 ) ) ;
#9943=VECTOR ( 'NONE', #5541, 1000.000000000000000 ) ;
#9944=VERTEX_POINT ( 'NONE', #10260 ) ;
#9950=ADVANCED_FACE ( 'NONE', ( #11278 ), #5203, .F. ) ;
#9951=CARTESIAN_POINT ( 'NONE',  ( 8.035510277249453992, 25.96172493762885480, 86.21852126538452410 ) ) ;
#9952=CARTESIAN_POINT ( 'NONE',  ( 49.99999999999998579, 0.000000000000000000, 169.9999999999999716 ) ) ;
#9954=DIRECTION ( 'NONE',  ( 0.000000000000000000, 0.000000000000000000, -1.000000000000000000 ) ) ;
#9956=B_SPLINE_CURVE_WITH_KNOTS ( 'NONE', 3,
 ( #7226, #11037, #4307, #2347, #4431, #5267, #3356, #1517, #5394, #9266, #445, #3541, #566, #9327, #10151, #6215, #3480, #1462, #629, #7413, #8309, #10322, #1580, #12177, #10088, #10264, #4249, #5459, #2528, #11096, #7347, #9076, #11217, #5207, #4494, #2589, #385, #8121, #2403, #11991, #3295, #7159, #6639, #1698, #8430, #1885, #11406, #11533 ),
 .UNSPECIFIED., .F., .F.,
 ( 4, 2, 2, 2, 2, 2, 2, 2, 2, 2, 2, 2, 2, 2, 2, 2, 2, 2, 2, 2, 2, 2, 2, 4 ),
 ( 3.469446951953614189E-18, 0.001535279795446541822, 0.002302919693169815877, 0.003070559590893089715, 0.003838199488616363120, 0.004605839386339637825, 0.006141119181786200247, 0.007676398977232760067, 0.009211678772679319019, 0.009979318670402598929, 0.01074695856812587884, 0.01151459846584915875, 0.01228223836357244039, 0.01304987826129572030, 0.01381751815901900195, 0.01458515805674228012, 0.01535279795446556003, 0.01688807774991211985, 0.01842335754535867967, 0.01995863734080524296, 0.02149391713625179931, 0.02226155703397508789, 0.02302919693169837301, 0.02456447672714493283 ),
 .UNSPECIFIED. ) ;
#9957=CARTESIAN_POINT ( 'NONE',  ( 43.17500000054622689, 26.92701409722686634, 88.54243821818162985 ) ) ;
#9960=ADVANCED_FACE ( 'NONE', ( #10085 ), #1397, .F. ) ;
#9961=VECTOR ( 'NONE', #12123, 1000.000000000000114 ) ;
#9963=CARTESIAN_POINT ( 'NONE',  ( 22.17500000054622333, 13.80429023900056507, 95.29460816699764791 ) ) ;
#9964=CARTESIAN_POINT ( 'NONE',  ( 44.47500000054622404, 13.07298590277314432, 88.54243821818161564 ) ) ;
#9965=CARTESIAN_POINT ( 'NONE',  ( 33.37500000054622973, 26.92701409722686634, 93.04388485072563242 ) ) ;
#9966=CARTESIAN_POINT ( 'NONE',  ( 21.47500000054622404, 26.92701409722686634, 93.04388485072563242 ) ) ;
#9967=CARTESIAN_POINT ( 'NONE',  ( 21.29999999999999005, 26.37988106264029398, 86.15790661882942914 ) ) ;
#9968=CARTESIAN_POINT ( 'NONE',  ( 28.57500000054622902, 15.71886984736413773, 84.90069139318163138 ) ) ;
#9970=CARTESIAN_POINT ( 'NONE',  ( 4.999999999999999112, 0.000000000000000000, 169.9999999999999716 ) ) ;
#9975=CARTESIAN_POINT ( 'NONE',  ( 0.000000000000000000, 22.00000000000000000, 169.9999999999999716 ) ) ;
#9976=CARTESIAN_POINT ( 'NONE',  ( 38.47500000054622404, 13.07298590277314432, 88.54243821818161564 ) ) ;
#9979=CARTESIAN_POINT ( 'NONE',  ( 19.95000000109246230, 13.62011893735970958, 95.42841645007781892 ) ) ;
#9980=CARTESIAN_POINT ( 'NONE',  ( 41.77500000054621410, 22.36655054427230027, 98.07665518445361386 ) ) ;
#9981=CARTESIAN_POINT ( 'NONE',  ( 44.49999999999999289, 12.11403331821300533, 90.79316153445363113 ) ) ;
#9982=CARTESIAN_POINT ( 'NONE',  ( 46.57500000054622546, 15.71886984736413773, 84.90069139318163138 ) ) ;
#9984=CARTESIAN_POINT ( 'NONE',  ( 27.65000000109246514, 20.00000000000000355, 98.29316153445363113 ) ) ;
#9986=ORIENTED_EDGE ( 'NONE', *, *, #9086, .T. ) ;
#9988=ORIENTED_EDGE ( 'NONE', *, *, #391, .T. ) ;
#9989=DIRECTION ( 'NONE',  ( -0.000000000000000000, -0.000000000000000000, 1.000000000000000000 ) ) ;
#9990=CARTESIAN_POINT ( 'NONE',  ( 41.55000000109246372, 22.43689772174679575, 98.29316153445363113 ) ) ;
#9991=CARTESIAN_POINT ( 'NONE',  ( 48.79999999999999005, 15.59161060780646046, 84.72553407664153724 ) ) ;
#9992=EDGE_CURVE ( 'NONE', #513, #11209, #563, .T. ) ;
#9993=CARTESIAN_POINT ( 'NONE',  ( 33.67500000054623399, 22.36655054427230027, 98.07665518445361386 ) ) ;
#9994=CARTESIAN_POINT ( 'NONE',  ( 32.97500000054621694, 22.36655054427230382, 83.50966788445364841 ) ) ;
#9996=VECTOR ( 'NONE', #1274, 1000.000000000000000 ) ;
#9997=CARTESIAN_POINT ( 'NONE',  ( 49.99999999999998579, 20.00000000000000355, 98.29316153445363113 ) ) ;
#9999=DIRECTION ( 'NONE',  ( -1.000000000000000000, 0.000000000000000000, 0.000000000000000000 ) ) ;
#10002=CARTESIAN_POINT ( 'NONE',  ( 41.05000000109246372, 27.13292387221364876, 88.47553407664153724 ) ) ;
#10005=CARTESIAN_POINT ( 'NONE',  ( 45.65000000109247225, 20.00000000000000355, 98.29316153445363113 ) ) ;
#10011=CARTESIAN_POINT ( 'NONE',  ( 10.00000000000000355, 20.25957311745080958, 83.29316153445364534 ) ) ;
#10015=EDGE_CURVE ( 'NONE', #8158, #9799, #3353, .T. ) ;
#10019=AXIS2_PLACEMENT_3D ( 'NONE', #1309, #9297, #11070 ) ;
#10020=CARTESIAN_POINT ( 'NONE',  ( 44.97500000054623115, 24.28113015263587471, 84.90069139318163138 ) ) ;
#10027=CARTESIAN_POINT ( 'NONE',  ( 46.77500000054622831, 17.63344945572770328, 83.50966788445364841 ) ) ;
#10028=CARTESIAN_POINT ( 'NONE',  ( 31.57500000054622902, 24.28113015263587116, 96.68563167572563088 ) ) ;
#10030=CARTESIAN_POINT ( 'NONE',  ( 23.17500000054622689, 26.19570976099943493, 86.29171490190961435 ) ) ;
#10033=CARTESIAN_POINT ( 'NONE',  ( 26.17500000054623044, 13.07298590277314254, 93.04388485072563242 ) ) ;
#10035=CARTESIAN_POINT ( 'NONE',  ( 22.85000000109246443, 24.40838939219355197, 84.72553407664153724 ) ) ;
#10037=ORIENTED_EDGE ( 'NONE', *, *, #4697, .T. ) ;
#10038=CARTESIAN_POINT ( 'NONE',  ( 38.19999999999998863, 15.59161060780645691, 96.86078899226572503 ) ) ;
#10041=AXIS2_PLACEMENT_3D ( 'NONE', #1798, #11507, #2817 ) ;
#10042=CARTESIAN_POINT ( 'NONE',  ( 37.87500000054622262, 20.00000000000000355, 98.07665518445361386 ) ) ;
#10043=CARTESIAN_POINT ( 'NONE',  ( 36.99999999999999289, 20.00000000000000355, 83.29316153445364534 ) ) ;
#10044=CARTESIAN_POINT ( 'NONE',  ( 26.29999999999998295, 13.62011893735970958, 95.42841645007781892 ) ) ;
#10045=CARTESIAN_POINT ( 'NONE',  ( 41.07500000054622546, 24.28113015263587471, 84.90069139318163138 ) ) ;
#10046=CARTESIAN_POINT ( 'NONE',  ( 36.79999999999998295, 15.59161060780646046, 84.72553407664153724 ) ) ;
#10048=CARTESIAN_POINT ( 'NONE',  ( 43.87500000054622973, 17.63344945572769973, 98.07665518445361386 ) ) ;
#10050=CARTESIAN_POINT ( 'NONE',  ( 22.95000000109246230, 26.37988106264029398, 86.15790661882942914 ) ) ;
#10051=DIRECTION ( 'NONE',  ( 0.000000000000000000, 0.000000000000000000, 1.000000000000000000 ) ) ;
#10054=ORIENTED_EDGE ( 'NONE', *, *, #8294, .F. ) ;
#10055=DIRECTION ( 'NONE',  ( 1.000000000000000000, -0.000000000000000000, -0.000000000000000000 ) ) ;
#10059=CARTESIAN_POINT ( 'NONE',  ( 27.67500000054623044, 22.36655054427230027, 98.07665518445361386 ) ) ;
#10060=CARTESIAN_POINT ( 'NONE',  ( 28.27500000054622475, 13.07298590277314254, 93.04388485072563242 ) ) ;
#10063=ORIENTED_EDGE ( 'NONE', *, *, #12193, .T. ) ;
#10064=CARTESIAN_POINT ( 'NONE',  ( 42.75000000109245946, 22.43689772174679575, 83.29316153445363113 ) ) ;
#10066=VERTEX_POINT ( 'NONE', #1694 ) ;
#10067=CARTESIAN_POINT ( 'NONE',  ( 32.65000000109246514, 20.00000000000000355, 83.29316153445364534 ) ) ;
#10075=LINE ( 'NONE', #11084, #11729 ) ;
#10077=CARTESIAN_POINT ( 'NONE',  ( -50.00000000000001421, 0.000000000000000000, 169.9999999999999716 ) ) ;
#10084=EDGE_CURVE ( 'NONE', #1716, #6066, #4682, .T. ) ;
#10085=FACE_OUTER_BOUND ( 'NONE', #7724, .T. ) ;
#10086=CARTESIAN_POINT ( 'NONE',  ( 43.27500000054622120, 26.92701409722686634, 88.54243821818162985 ) ) ;
#10087=CARTESIAN_POINT ( 'NONE',  ( 25.37500000054622973, 26.92701409722686634, 93.04388485072563242 ) ) ;
#10088=CARTESIAN_POINT ( 'NONE',  ( 6.614382007193625235, 12.50000328913819381, 90.53699374271461409 ) ) ;
#10092=CARTESIAN_POINT ( 'NONE',  ( 29.77500000054622831, 20.00000000000000355, 98.07665518445361386 ) ) ;
#10094=FACE_OUTER_BOUND ( 'NONE', #4272, .T. ) ;
#10097=ORIENTED_EDGE ( 'NONE', *, *, #2722, .F. ) ;
#10100=VECTOR ( 'NONE', #6375, 1000.000000000000000 ) ;
#10101=CARTESIAN_POINT ( 'NONE',  ( 29.47500000054622404, 26.92701409722686634, 93.04388485072563242 ) ) ;
#10102=CARTESIAN_POINT ( 'NONE',  ( -5.000000000000004441, 20.00000000000000000, 145.0000000000000000 ) ) ;
#10103=CARTESIAN_POINT ( 'NONE',  ( 46.07500000054622546, 13.80429023900056507, 95.29460816699764791 ) ) ;
#10104=CARTESIAN_POINT ( 'NONE',  ( 33.97500000054620983, 17.63344945572769973, 98.07665518445361386 ) ) ;
#10105=CARTESIAN_POINT ( 'NONE',  ( 35.19999999999998863, 24.40838939219355197, 84.72553407664153724 ) ) ;
#10108=CARTESIAN_POINT ( 'NONE',  ( 48.87500000054622262, 22.36655054427230382, 83.50966788445364841 ) ) ;
#10110=CARTESIAN_POINT ( 'NONE',  ( 21.95000000109245875, 13.62011893735971135, 95.42841645007781892 ) ) ;
#10112=ORIENTED_EDGE ( 'NONE', *, *, #5202, .T. ) ;
#10115=VERTEX_POINT ( 'NONE', #12420 ) ;
#10118=CARTESIAN_POINT ( 'NONE',  ( 21.25000000109246301, 27.13292387221364876, 93.11078899226573924 ) ) ;
#10119=LINE ( 'NONE', #5298, #8864 ) ;
#10121=CIRCLE ( 'NONE', #6461, 7.499999999999978684 ) ;
#10122=CARTESIAN_POINT ( 'NONE',  ( 33.57500000054623257, 24.28113015263587116, 96.68563167572563088 ) ) ;
#10123=CARTESIAN_POINT ( 'NONE',  ( 26.57500000054622191, 13.80429023900056684, 86.29171490190961435 ) ) ;
#10125=VECTOR ( 'NONE', #8351, 1000.000000000000000 ) ;
#10127=VERTEX_POINT ( 'NONE', #10507 ) ;
#10128=CARTESIAN_POINT ( 'NONE',  ( 45.75000000109246656, 17.56310227825320425, 98.29316153445363113 ) ) ;
#10133=ORIENTED_EDGE ( 'NONE', *, *, #11465, .T. ) ;
#10136=DIRECTION ( 'NONE',  ( 0.000000000000000000, 0.000000000000000000, -1.000000000000000000 ) ) ;
#10140=DIRECTION ( 'NONE',  ( 1.000000000000000000, 0.000000000000000000, 0.000000000000000000 ) ) ;
#10142=CARTESIAN_POINT ( 'NONE',  ( 33.99999999999998579, 20.00000000000000355, 98.29316153445363113 ) ) ;
#10143=ORIENTED_EDGE ( 'NONE', *, *, #908, .F. ) ;
#10148=CARTESIAN_POINT ( 'NONE',  ( 41.57500000054622546, 26.19570976099943493, 95.29460816699764791 ) ) ;
#10149=CARTESIAN_POINT ( 'NONE',  ( 24.17500000054622689, 13.07298590277314254, 93.04388485072563242 ) ) ;
#10150=( BOUNDED_CURVE ( )  B_SPLINE_CURVE ( 2, ( #7295, #4257, #4378, #331, #4194, #9084, #1410, #8131, #10038, #2292, #2355 ),
 .UNSPECIFIED., .F., .F. ) 
 B_SPLINE_CURVE_WITH_KNOTS ( ( 3, 2, 2, 2, 2, 3 ),
 ( 0.3666666666666666963, 0.3733333333333333504, 0.3799999999999999489, 0.3866666666666666030, 0.3933333333333332016, 0.3999999999999998557 ),
 .UNSPECIFIED. ) 
 CURVE ( )  GEOMETRIC_REPRESENTATION_ITEM ( )  RATIONAL_B_SPLINE_CURVE ( ( 0.9999999999999995559, 0.9510565162951539753, 1.000000000000000000, 0.9510565162951535312, 1.000000000000000000, 0.9510565162951535312, 1.000000000000000000, 0.9510565162951535312, 1.000000000000000000, 0.9510565162951547524, 0.9999999999999987788 ) ) 
 REPRESENTATION_ITEM ( '' )  );
#10151=CARTESIAN_POINT ( 'NONE',  ( 8.033354630240914673, 14.03538636471792778, 86.22229691711790167 ) ) ;
#10152=LINE ( 'NONE', #567, #11005 ) ;
#10155=ORIENTED_EDGE ( 'NONE', *, *, #2996, .F. ) ;
#10156=VECTOR ( 'NONE', #9473, 1000.000000000000000 ) ;
#10158=ORIENTED_EDGE ( 'NONE', *, *, #12049, .F. ) ;
#10159=CARTESIAN_POINT ( 'NONE',  ( 36.99999999999995026, 40.00000000000000000, 69.99999999999998579 ) ) ;
#10160=ORIENTED_EDGE ( 'NONE', *, *, #9992, .T. ) ;
#10163=CARTESIAN_POINT ( 'NONE',  ( 30.17500000054621978, 13.80429023900056507, 95.29460816699764791 ) ) ;
#10165=CARTESIAN_POINT ( 'NONE',  ( 46.97500000054623115, 24.28113015263587471, 84.90069139318163138 ) ) ;
#10166=CARTESIAN_POINT ( 'NONE',  ( 34.07500000054622546, 15.71886984736413417, 96.68563167572563088 ) ) ;
#10167=CARTESIAN_POINT ( 'NONE',  ( 33.59999999999999432, 27.13292387221364876, 93.11078899226573924 ) ) ;
#10168=CARTESIAN_POINT ( 'NONE',  ( 43.07500000054622546, 26.19570976099943493, 86.29171490190961435 ) ) ;
#10169=ORIENTED_EDGE ( 'NONE', *, *, #3200, .F. ) ;
#10170=CARTESIAN_POINT ( 'NONE',  ( 21.85000000109246443, 15.59161060780645691, 96.86078899226572503 ) ) ;
#10172=ORIENTED_EDGE ( 'NONE', *, *, #5676, .T. ) ;
#10177=LINE ( 'NONE', #11067, #288 ) ;
#10178=CARTESIAN_POINT ( 'NONE',  ( 26.67500000054622689, 17.63344945572770328, 83.50966788445364841 ) ) ;
#10179=CARTESIAN_POINT ( 'NONE',  ( 25.47500000054622404, 26.92701409722686634, 93.04388485072563242 ) ) ;
#10184=VERTEX_POINT ( 'NONE', #4552 ) ;
#10185=CARTESIAN_POINT ( 'NONE',  ( 44.15000000109247225, 12.11403331821300533, 90.79316153445363113 ) ) ;
#10186=CARTESIAN_POINT ( 'NONE',  ( 45.99999999999998579, 20.00000000000000355, 98.29316153445363113 ) ) ;
#10188=DIRECTION ( 'NONE',  ( 1.000000000000000000, -0.000000000000000000, -0.000000000000000000 ) ) ;
#10189=ORIENTED_EDGE ( 'NONE', *, *, #7470, .F. ) ;
#10196=CARTESIAN_POINT ( 'NONE',  ( 42.29999999999998295, 13.62011893735970958, 95.42841645007781892 ) ) ;
#10198=LINE ( 'NONE', #9255, #12467 ) ;
#10199=VECTOR ( 'NONE', #6584, 1000.000000000000114 ) ;
#10200=CARTESIAN_POINT ( 'NONE',  ( 23.89999999999998792, 22.43689772174679575, 98.29316153445363113 ) ) ;
#10203=CARTESIAN_POINT ( 'NONE',  ( 43.17500000054621978, 26.19570976099943493, 86.29171490190961435 ) ) ;
#10204=VECTOR ( 'NONE', #2637, 1000.000000000000000 ) ;
#10205=CARTESIAN_POINT ( 'NONE',  ( 28.17500000054622689, 13.07298590277314254, 93.04388485072563242 ) ) ;
#10206=LINE ( 'NONE', #4372, #1197 ) ;
#10207=PLANE ( 'NONE',  #10676 ) ;
#10208=CARTESIAN_POINT ( 'NONE',  ( 33.79999999999999005, 24.40838939219354842, 96.86078899226572503 ) ) ;
#10209=DIRECTION ( 'NONE',  ( -0.000000000000000000, -0.7071067811865511255, -0.7071067811865440200 ) ) ;
#10212=VERTEX_POINT ( 'NONE', #2585 ) ;
#10213=CYLINDRICAL_SURFACE ( 'NONE', #7925, 7.499999999999992895 ) ;
#10217=( BOUNDED_SURFACE ( )  B_SPLINE_SURFACE ( 1, 2, ( 
 ( #10864, #914, #4782, #8647, #12519, #7699, #11566, #3252, #1230, #10108, #7118, #3192, #4386, #12133, #6112, #344, #10930, #7053, #10993, #4207, #402, #2302, #9920, #3441, #7305, #2421, #9158, #2245, #11115, #5099, #6298, #3373, #9982, #11056, #8964, #2363, #11178, #8203, #6047, #1475, #277, #9032, #5287, #4140, #8015, #1419, #11948, #463, #11886, #6171, #6234, #5347, #526, #1291, #5164, #8080, #1358, #4325, #12072, #10048, #5225, #9095, #7243, #4266, #8142, #8264, #12008, #10168, #3311, #9219, #7178, #2735, #6535, #2481, #1538, #1772, #11302, #1715, #6357, #5411, #10403, #8386, #5596, #10224, #2608, #7494, #5657, #9529, #7366, #585, #8570, #10340, #9467, #4635, #4451, #8329, #12441, #11365, #9345, #5538, #4698, #9282, #2672, #3558, #766, #3739, #6594, #8506, #12195, #3495, #828, #6477, #11426, #4511, #1597, #6416, #1657, #9404, #11235, #2544, #12381, #5478, #7431, #10280, #648, #12255, #10462, #7620, #3679, #706, #7557, #4575, #8447, #12316, #3615, #1155, #3933, #1838, #8882, #10715, #8630, #4830, #7745, #5781, #9655, #11742, #7807, #2794, #1964, #9587, #8696, #3049, #5966, #5720, #6910, #8816, #3869, #894, #10777, #9777, #9715, #9842, #4764, #2921, #11613, #5844, #5017, #135, #5, #1030, #6784, #6656, #2986, #10651, #12500, #200, #4056, #11548, #962, #3805, #7684, #4892, #8752, #68, #11680, #10525, #11484, #2859, #7872, #2026, #6720, #3994, #10587, #2090, #1899, #6852, #5909, #1087, #4953, #678, #10092, #5510, #3528, #9377, #10914, #7999, #2159, #8190, #5149, #5271, #1218, #5084, #9968, #2287, #1276, #2229, #3176, #3238, #11871, #2578, #10311, #6158, #9015, #12226, #326, #4252, #9143, #2351, #1630, #3298, #8124, #1406, #7401, #11272, #6976, #9905, #10033, #7936, #7039, #11994, #9079, #449, #6449, #6218, #1342, #11799, #7099, #3107, #10846, #4311, #5209, #6097, #4189, #265, #6031, #8952, #4121, #10980, #7163, #8064, #11933, #388, #11040, #12412, #8481, #2830, #5754, #12473, #10622, #10500, #3710, #8420, #9625, #11459, #9563, #11519, #2766, #6695, #10563, #1686, #3775, #8603, #6570, #3590, #1935, #6628, #933, #12535, #12290, #10435, #10373, #3651, #5568, #7653, #740, #7529, #1811, #7593, #8545, #12352, #7719 ),
 ( #11396, #863, #9438, #1746, #4800, #4545, #1873, #2705, #5697, #5627, #2894, #4733, #9501, #4607, #8665, #804, #3843, #11586, #5815, #6757, #9688, #7465, #11339, #6509, #2644, #4674, #9545, #1911, #11563, #3882, #1045, #20, #8644, #2997, #910, #10416, #5859, #7756, #12516, #5674, #2808, #6608, #781, #11628, #83, #4779, #5796, #6799, #4906, #8765, #2872, #5734, #843, #10665, #1975, #9666, #7823, #3820, #6733, #1730, #9728, #976, #5609, #4650, #8520, #3691, #7570, #11438, #10479, #4711, #3755, #11500, #6672, #10542, #1852, #2300, #10727, #214, #149, #5980, #4006, #9980, #3061, #9854, #4138, #9918, #10861, #2103, #10045, #2171, #1289, #1169, #12006, #5162, #3121, #1356, #5222, #7949, #5032, #3189, #11752, #4071, #8078, #6864, #9029, #6044, #1227, #5097, #9093, #8962, #8011, #11884, #7050, #10928, #7116, #2242, #4263, #341, #3250, #4204, #11945, #400, #1101, #8140, #2040, #5920, #9790, #4967, #8830, #10221, #5345, #6295, #11113, #11175, #3371, #10336, #5535, #1534, #4383, #7428, #9216, #3492, #644, #10276, #9400, #11231, #7363, #5475, #3554, #11298, #2361, #6353, #6231, #7176, #4507, #2418, #8260, #461, #10166, #10104, #2604, #1654, #9341, #8200, #8383, #2478, #12251, #522, #9278, #703, #8325, #5284, #4571, #6413, #4323, #12130, #3438, #1472, #7300, #6474, #1594, #11053, #5407, #9155, #582, #8443, #3308, #12070, #7240, #4448, #4694, #10400, #11610, #10585, #10521, #10648, #5593, #3736, #12438, #6653, #6781, #959, #824, #2791, #9526, #7490, #3802, #8567, #9464, #1961, #5841, #12376, #6590, #4633, #762, #7617, #10459, #1834, #11480, #3612, #9712, #1027, #8692, #2854, #8503, #4827, #11361, #2, #9651, #3676, #4760, #2669, #8627, #4888, #1896, #12313, #7742, #6532, #2732, #11545, #1711, #7554, #7681, #5653, #6717, #11424, #5717, #12497, #2918, #1769, #9584, #890, #5778, #3866, #11866, #10911, #10712, #6849, #6155, #5081, #3046, #11796, #10977, #2983, #1215, #9839, #8949, #10030, #9012, #262, #8749, #7805, #8061, #5014, #5146, #10773, #7869, #132, #8879, #4118, #2285, #2156, #4053, #65, #9966, #3103, #7996, #3173, #6973, #7036, #2226, #5904, #6094, #1273, #2087, #11677, #1338, #10842, #323, #4186, #3930 ) ),
 .UNSPECIFIED., .F., .F., .F. ) 
 B_SPLINE_SURFACE_WITH_KNOTS ( ( 2, 2 ),
 ( 3, 2, 2, 2, 2, 2, 2, 2, 2, 2, 2, 2, 2, 2, 2, 2, 2, 2, 2, 2, 2, 2, 2, 2, 2, 2, 2, 2, 2, 2, 2, 2, 2, 2, 2, 2, 2, 2, 2, 2, 2, 2, 2, 2, 2, 2, 2, 2, 2, 2, 2, 2, 2, 2, 2, 2, 2, 2, 2, 2, 2, 2, 2, 2, 2, 2, 2, 2, 2, 2, 2, 2, 2, 2, 2, 2, 2, 2, 2, 2, 2, 2, 2, 2, 2, 2, 2, 2, 2, 2, 2, 2, 2, 2, 2, 2, 2, 2, 2, 2, 2, 2, 2, 2, 2, 2, 2, 2, 2, 2, 2, 2, 2, 2, 2, 2, 2, 2, 2, 2, 2, 2, 2, 2, 2, 2, 2, 2, 2, 2, 2, 2, 2, 2, 2, 2, 2, 2, 2, 2, 2, 2, 2, 2, 2, 2, 2, 2, 2, 2, 3 ),
 ( 0.000000000000000000, 1.000000000000000000 ),
 ( 0.000000000000000000, 0.006666666666666667095, 0.01333333333333333419, 0.02000000000000000042, 0.02666666666666666838, 0.03333333333333333287, 0.04000000000000000083, 0.04666666666666666879, 0.05333333333333333676, 0.05999999999999999778, 0.06666666666666666574, 0.07333333333333333370, 0.08000000000000000167, 0.08666666666666666963, 0.09333333333333333759, 0.1000000000000000056, 0.1066666666666666735, 0.1133333333333333276, 0.1199999999999999956, 0.1266666666666666774, 0.1333333333333333315, 0.1400000000000000133, 0.1466666666666666674, 0.1533333333333333215, 0.1600000000000000033, 0.1666666666666666574, 0.1733333333333333393, 0.1799999999999999933, 0.1866666666666666752, 0.1933333333333333293, 0.2000000000000000111, 0.2066666666666666652, 0.2133333333333333470, 0.2200000000000000011, 0.2266666666666666552, 0.2333333333333333370, 0.2399999999999999911, 0.2466666666666666730, 0.2533333333333333548, 0.2600000000000000089, 0.2666666666666666630, 0.2733333333333333171, 0.2800000000000000266, 0.2866666666666666807, 0.2933333333333333348, 0.2999999999999999889, 0.3066666666666666430, 0.3133333333333333526, 0.3200000000000000067, 0.3266666666666666607, 0.3333333333333333148, 0.3400000000000000244, 0.3466666666666666785, 0.3533333333333333326, 0.3599999999999999867, 0.3666666666666666408, 0.3733333333333333504, 0.3800000000000000044, 0.3866666666666666585, 0.3933333333333333126, 0.4000000000000000222, 0.4066666666666666763, 0.4133333333333333304, 0.4199999999999999845, 0.4266666666666666941, 0.4333333333333333481, 0.4400000000000000022, 0.4466666666666666563, 0.4533333333333333104, 0.4600000000000000200, 0.4666666666666666741, 0.4733333333333333282, 0.4799999999999999822, 0.4866666666666666918, 0.4933333333333333459, 0.5000000000000000000, 0.5066666666666667096, 0.5133333333333333082, 0.5200000000000000178, 0.5266666666666666163, 0.5333333333333333259, 0.5400000000000000355, 0.5466666666666666341, 0.5533333333333333437, 0.5600000000000000533, 0.5666666666666666519, 0.5733333333333333615, 0.5799999999999999600, 0.5866666666666666696, 0.5933333333333333792, 0.5999999999999999778, 0.6066666666666666874, 0.6133333333333332860, 0.6199999999999999956, 0.6266666666666667052, 0.6333333333333333037, 0.6400000000000000133, 0.6466666666666666119, 0.6533333333333333215, 0.6600000000000000311, 0.6666666666666666297, 0.6733333333333333393, 0.6800000000000000488, 0.6866666666666666474, 0.6933333333333333570, 0.6999999999999999556, 0.7066666666666666652, 0.7133333333333333748, 0.7199999999999999734, 0.7266666666666666829, 0.7333333333333332815, 0.7399999999999999911, 0.7466666666666667007, 0.7533333333333332993, 0.7600000000000000089, 0.7666666666666667185, 0.7733333333333333171, 0.7800000000000000266, 0.7866666666666666252, 0.7933333333333333348, 0.8000000000000000444, 0.8066666666666666430, 0.8133333333333333526, 0.8199999999999999512, 0.8266666666666666607, 0.8333333333333333703, 0.8399999999999999689, 0.8466666666666666785, 0.8533333333333333881, 0.8599999999999999867, 0.8666666666666666963, 0.8733333333333332948, 0.8800000000000000044, 0.8866666666666667140, 0.8933333333333333126, 0.9000000000000000222, 0.9066666666666666208, 0.9133333333333333304, 0.9200000000000000400, 0.9266666666666666385, 0.9333333333333333481, 0.9399999999999999467, 0.9466666666666666563, 0.9533333333333333659, 0.9599999999999999645, 0.9666666666666666741, 0.9733333333333333837, 0.9799999999999999822, 0.9866666666666666918, 0.9933333333333332904, 1.000000000000000000 ),
 .UNSPECIFIED. ) 
 GEOMETRIC_REPRESENTATION_ITEM ( )  RATIONAL_B_SPLINE_SURFACE ( (
 ( 1.000000000000000000, 0.9510565162951535312, 1.000000000000000000, 0.9510565162951535312, 1.000000000000000000, 0.9510565162951535312, 1.000000000000000000, 0.9510565162951535312, 1.000000000000000000, 0.9510565162951535312, 1.000000000000000000, 0.9510565162951535312, 1.000000000000000000, 0.9510565162951535312, 1.000000000000000000, 0.9510565162951535312, 1.000000000000000000, 0.9510565162951535312, 1.000000000000000000, 0.9510565162951535312, 1.000000000000000000, 0.9510565162951535312, 1.000000000000000000, 0.9510565162951535312, 1.000000000000000000, 0.9510565162951535312, 1.000000000000000000, 0.9510565162951535312, 1.000000000000000000, 0.9510565162951535312, 1.000000000000000000, 0.9510565162951535312, 1.000000000000000000, 0.9510565162951535312, 1.000000000000000000, 0.9510565162951535312, 1.000000000000000000, 0.9510565162951535312, 1.000000000000000000, 0.9510565162951535312, 1.000000000000000000, 0.9510565162951535312, 1.000000000000000000, 0.9510565162951535312, 1.000000000000000000, 0.9510565162951535312, 1.000000000000000000, 0.9510565162951535312, 1.000000000000000000, 0.9510565162951535312, 1.000000000000000000, 0.9510565162951535312, 1.000000000000000000, 0.9510565162951535312, 1.000000000000000000, 0.9510565162951535312, 1.000000000000000000, 0.9510565162951535312, 1.000000000000000000, 0.9510565162951535312, 1.000000000000000000, 0.9510565162951535312, 1.000000000000000000, 0.9510565162951535312, 1.000000000000000000, 0.9510565162951535312, 1.000000000000000000, 0.9510565162951535312, 1.000000000000000000, 0.9510565162951535312, 1.000000000000000000, 0.9510565162951535312, 1.000000000000000000, 0.9510565162951535312, 1.000000000000000000, 0.9510565162951535312, 1.000000000000000000, 0.9510565162951535312, 1.000000000000000000, 0.9510565162951535312, 1.000000000000000000, 0.9510565162951535312, 1.000000000000000000, 0.9510565162951535312, 1.000000000000000000, 0.9510565162951535312, 1.000000000000000000, 0.9510565162951535312, 1.000000000000000000, 0.9510565162951535312, 1.000000000000000000, 0.9510565162951535312, 1.000000000000000000, 0.9510565162951535312, 1.000000000000000000, 0.9510565162951535312, 1.000000000000000000, 0.9510565162951535312, 1.000000000000000000, 0.9510565162951535312, 1.000000000000000000, 0.9510565162951535312, 1.000000000000000000, 0.9510565162951535312, 1.000000000000000000, 0.9510565162951535312, 1.000000000000000000, 0.9510565162951535312, 1.000000000000000000, 0.9510565162951535312, 1.000000000000000000, 0.9510565162951535312, 1.000000000000000000, 0.9510565162951535312, 1.000000000000000000, 0.9510565162951535312, 1.000000000000000000, 0.9510565162951535312, 1.000000000000000000, 0.9510565162951535312, 1.000000000000000000, 0.9510565162951535312, 1.000000000000000000, 0.9510565162951535312, 1.000000000000000000, 0.9510565162951535312, 1.000000000000000000, 0.9510565162951535312, 1.000000000000000000, 0.9510565162951535312, 1.000000000000000000, 0.9510565162951535312, 1.000000000000000000, 0.9510565162951535312, 1.000000000000000000, 0.9510565162951535312, 1.000000000000000000, 0.9510565162951535312, 1.000000000000000000, 0.9510565162951535312, 1.000000000000000000, 0.9510565162951535312, 1.000000000000000000, 0.9510565162951535312, 1.000000000000000000, 0.9510565162951535312, 1.000000000000000000, 0.9510565162951535312, 1.000000000000000000, 0.9510565162951535312, 1.000000000000000000, 0.9510565162951535312, 1.000000000000000000, 0.9510565162951535312, 1.000000000000000000, 0.9510565162951535312, 1.000000000000000000, 0.9510565162951535312, 1.000000000000000000, 0.9510565162951535312, 1.000000000000000000, 0.9510565162951535312, 1.000000000000000000, 0.9510565162951535312, 1.000000000000000000, 0.9510565162951535312, 1.000000000000000000, 0.9510565162951535312, 1.000000000000000000, 0.9510565162951535312, 1.000000000000000000, 0.9510565162951535312, 1.000000000000000000, 0.9510565162951535312, 1.000000000000000000, 0.9510565162951535312, 1.000000000000000000, 0.9510565162951535312, 1.000000000000000000, 0.9510565162951535312, 1.000000000000000000, 0.9510565162951535312, 1.000000000000000000, 0.9510565162951535312, 1.000000000000000000, 0.9510565162951535312, 1.000000000000000000, 0.9510565162951535312, 1.000000000000000000, 0.9510565162951535312, 1.000000000000000000, 0.9510565162951535312, 1.000000000000000000, 0.9510565162951535312, 1.000000000000000000, 0.9510565162951535312, 1.000000000000000000, 0.9510565162951535312, 1.000000000000000000, 0.9510565162951535312, 1.000000000000000000, 0.9510565162951535312, 1.000000000000000000, 0.9510565162951535312, 1.000000000000000000, 0.9510565162951535312, 1.000000000000000000, 0.9510565162951535312, 1.000000000000000000, 0.9510565162951535312, 1.000000000000000000, 0.9510565162951535312, 1.000000000000000000, 0.9510565162951535312, 1.000000000000000000, 0.9510565162951535312, 1.000000000000000000, 0.9510565162951535312, 1.000000000000000000, 0.9510565162951535312, 1.000000000000000000, 0.9510565162951535312, 1.000000000000000000, 0.9510565162951535312, 1.000000000000000000, 0.9510565162951535312, 1.000000000000000000, 0.9510565162951535312, 1.000000000000000000, 0.9510565162951535312, 1.000000000000000000, 0.9510565162951535312, 1.000000000000000000, 0.9510565162951535312, 1.000000000000000000, 0.9510565162951535312, 1.000000000000000000, 0.9510565162951535312, 1.000000000000000000, 0.9510565162951535312, 1.000000000000000000, 0.9510565162951535312, 1.000000000000000000, 0.9510565162951535312, 1.000000000000000000, 0.9510565162951535312, 1.000000000000000000, 0.9510565162951535312, 1.000000000000000000, 0.9510565162951535312, 1.000000000000000000, 0.9510565162951535312, 1.000000000000000000, 0.9510565162951535312, 1.000000000000000000, 0.9510565162951535312, 1.000000000000000000, 0.9510565162951535312, 1.000000000000000000, 0.9510565162951535312, 1.000000000000000000, 0.9510565162951535312, 1.000000000000000000, 0.9510565162951535312, 1.000000000000000000, 0.9510565162951535312, 1.000000000000000000, 0.9510565162951535312, 1.000000000000000000, 0.9510565162951535312, 1.000000000000000000, 0.9510565162951535312, 1.000000000000000000, 0.9510565162951535312, 1.000000000000000000, 0.9510565162951535312, 1.000000000000000000, 0.9510565162951535312, 1.000000000000000000, 0.9510565162951535312, 1.000000000000000000, 0.9510565162951535312, 1.000000000000000000, 0.9510565162951535312, 1.000000000000000000, 0.9510565162951535312, 1.000000000000000000, 0.9510565162951535312, 1.000000000000000000, 0.9510565162951535312, 1.000000000000000000, 0.9510565162951535312, 1.000000000000000000, 0.9510565162951535312, 1.000000000000000000, 0.9510565162951535312, 1.000000000000000000, 0.9510565162951535312, 1.000000000000000000, 0.9510565162951535312, 1.000000000000000000),
 ( 1.000000000000000000, 0.9510565162951535312, 1.000000000000000000, 0.9510565162951535312, 1.000000000000000000, 0.9510565162951535312, 1.000000000000000000, 0.9510565162951535312, 1.000000000000000000, 0.9510565162951535312, 1.000000000000000000, 0.9510565162951535312, 1.000000000000000000, 0.9510565162951535312, 1.000000000000000000, 0.9510565162951535312, 1.000000000000000000, 0.9510565162951535312, 1.000000000000000000, 0.9510565162951535312, 1.000000000000000000, 0.9510565162951535312, 1.000000000000000000, 0.9510565162951535312, 1.000000000000000000, 0.9510565162951535312, 1.000000000000000000, 0.9510565162951535312, 1.000000000000000000, 0.9510565162951535312, 1.000000000000000000, 0.9510565162951535312, 1.000000000000000000, 0.9510565162951535312, 1.000000000000000000, 0.9510565162951535312, 1.000000000000000000, 0.9510565162951535312, 1.000000000000000000, 0.9510565162951535312, 1.000000000000000000, 0.9510565162951535312, 1.000000000000000000, 0.9510565162951535312, 1.000000000000000000, 0.9510565162951535312, 1.000000000000000000, 0.9510565162951535312, 1.000000000000000000, 0.9510565162951535312, 1.000000000000000000, 0.9510565162951535312, 1.000000000000000000, 0.9510565162951535312, 1.000000000000000000, 0.9510565162951535312, 1.000000000000000000, 0.9510565162951535312, 1.000000000000000000, 0.9510565162951535312, 1.000000000000000000, 0.9510565162951535312, 1.000000000000000000, 0.9510565162951535312, 1.000000000000000000, 0.9510565162951535312, 1.000000000000000000, 0.9510565162951535312, 1.000000000000000000, 0.9510565162951535312, 1.000000000000000000, 0.9510565162951535312, 1.000000000000000000, 0.9510565162951535312, 1.000000000000000000, 0.9510565162951535312, 1.000000000000000000, 0.9510565162951535312, 1.000000000000000000, 0.9510565162951535312, 1.000000000000000000, 0.9510565162951535312, 1.000000000000000000, 0.9510565162951535312, 1.000000000000000000, 0.9510565162951535312, 1.000000000000000000, 0.9510565162951535312, 1.000000000000000000, 0.9510565162951535312, 1.000000000000000000, 0.9510565162951535312, 1.000000000000000000, 0.9510565162951535312, 1.000000000000000000, 0.9510565162951535312, 1.000000000000000000, 0.9510565162951535312, 1.000000000000000000, 0.9510565162951535312, 1.000000000000000000, 0.9510565162951535312, 1.000000000000000000, 0.9510565162951535312, 1.000000000000000000, 0.9510565162951535312, 1.000000000000000000, 0.9510565162951535312, 1.000000000000000000, 0.9510565162951535312, 1.000000000000000000, 0.9510565162951535312, 1.000000000000000000, 0.9510565162951535312, 1.000000000000000000, 0.9510565162951535312, 1.000000000000000000, 0.9510565162951535312, 1.000000000000000000, 0.9510565162951535312, 1.000000000000000000, 0.9510565162951535312, 1.000000000000000000, 0.9510565162951535312, 1.000000000000000000, 0.9510565162951535312, 1.000000000000000000, 0.9510565162951535312, 1.000000000000000000, 0.9510565162951535312, 1.000000000000000000, 0.9510565162951535312, 1.000000000000000000, 0.9510565162951535312, 1.000000000000000000, 0.9510565162951535312, 1.000000000000000000, 0.9510565162951535312, 1.000000000000000000, 0.9510565162951535312, 1.000000000000000000, 0.9510565162951535312, 1.000000000000000000, 0.9510565162951535312, 1.000000000000000000, 0.9510565162951535312, 1.000000000000000000, 0.9510565162951535312, 1.000000000000000000, 0.9510565162951535312, 1.000000000000000000, 0.9510565162951535312, 1.000000000000000000, 0.9510565162951535312, 1.000000000000000000, 0.9510565162951535312, 1.000000000000000000, 0.9510565162951535312, 1.000000000000000000, 0.9510565162951535312, 1.000000000000000000, 0.9510565162951535312, 1.000000000000000000, 0.9510565162951535312, 1.000000000000000000, 0.9510565162951535312, 1.000000000000000000, 0.9510565162951535312, 1.000000000000000000, 0.9510565162951535312, 1.000000000000000000, 0.9510565162951535312, 1.000000000000000000, 0.9510565162951535312, 1.000000000000000000, 0.9510565162951535312, 1.000000000000000000, 0.9510565162951535312, 1.000000000000000000, 0.9510565162951535312, 1.000000000000000000, 0.9510565162951535312, 1.000000000000000000, 0.9510565162951535312, 1.000000000000000000, 0.9510565162951535312, 1.000000000000000000, 0.9510565162951535312, 1.000000000000000000, 0.9510565162951535312, 1.000000000000000000, 0.9510565162951535312, 1.000000000000000000, 0.9510565162951535312, 1.000000000000000000, 0.9510565162951535312, 1.000000000000000000, 0.9510565162951535312, 1.000000000000000000, 0.9510565162951535312, 1.000000000000000000, 0.9510565162951535312, 1.000000000000000000, 0.9510565162951535312, 1.000000000000000000, 0.9510565162951535312, 1.000000000000000000, 0.9510565162951535312, 1.000000000000000000, 0.9510565162951535312, 1.000000000000000000, 0.9510565162951535312, 1.000000000000000000, 0.9510565162951535312, 1.000000000000000000, 0.9510565162951535312, 1.000000000000000000, 0.9510565162951535312, 1.000000000000000000, 0.9510565162951535312, 1.000000000000000000, 0.9510565162951535312, 1.000000000000000000, 0.9510565162951535312, 1.000000000000000000, 0.9510565162951535312, 1.000000000000000000, 0.9510565162951535312, 1.000000000000000000, 0.9510565162951535312, 1.000000000000000000, 0.9510565162951535312, 1.000000000000000000, 0.9510565162951535312, 1.000000000000000000, 0.9510565162951535312, 1.000000000000000000, 0.9510565162951535312, 1.000000000000000000, 0.9510565162951535312, 1.000000000000000000, 0.9510565162951535312, 1.000000000000000000, 0.9510565162951535312, 1.000000000000000000, 0.9510565162951535312, 1.000000000000000000, 0.9510565162951535312, 1.000000000000000000, 0.9510565162951535312, 1.000000000000000000, 0.9510565162951535312, 1.000000000000000000, 0.9510565162951535312, 1.000000000000000000, 0.9510565162951535312, 1.000000000000000000, 0.9510565162951535312, 1.000000000000000000, 0.9510565162951535312, 1.000000000000000000, 0.9510565162951535312, 1.000000000000000000, 0.9510565162951535312, 1.000000000000000000, 0.9510565162951535312, 1.000000000000000000, 0.9510565162951535312, 1.000000000000000000, 0.9510565162951535312, 1.000000000000000000, 0.9510565162951535312, 1.000000000000000000, 0.9510565162951535312, 1.000000000000000000, 0.9510565162951535312, 1.000000000000000000, 0.9510565162951535312, 1.000000000000000000, 0.9510565162951535312, 1.000000000000000000, 0.9510565162951535312, 1.000000000000000000, 0.9510565162951535312, 1.000000000000000000, 0.9510565162951535312, 1.000000000000000000, 0.9510565162951535312, 1.000000000000000000, 0.9510565162951535312, 1.000000000000000000, 0.9510565162951535312, 1.000000000000000000, 0.9510565162951535312, 1.000000000000000000, 0.9510565162951535312, 1.000000000000000000, 0.9510565162951535312, 1.000000000000000000, 0.9510565162951535312, 1.000000000000000000) ) ) 
 REPRESENTATION_ITEM ( '' )  SURFACE ( )  );
#10218=CARTESIAN_POINT ( 'NONE',  ( 34.67500000054622689, 15.71886984736413773, 84.90069139318163138 ) ) ;
#10220=CARTESIAN_POINT ( 'NONE',  ( 45.47500000054623115, 26.19570976099943849, 95.29460816699764791 ) ) ;
#10221=CARTESIAN_POINT ( 'NONE',  ( 36.97500000054623115, 22.36655054427230382, 83.50966788445364841 ) ) ;
#10222=CARTESIAN_POINT ( 'NONE',  ( 33.49999999999998579, 27.88596668178699645, 90.79316153445363113 ) ) ;
#10224=CARTESIAN_POINT ( 'NONE',  ( 41.47500000054623115, 26.19570976099943493, 95.29460816699764791 ) ) ;
#10226=AXIS2_PLACEMENT_3D ( 'NONE', #9699, #8494, #8680 ) ;
#10227=CARTESIAN_POINT ( 'NONE',  ( 26.25000000109246656, 12.86707612778636012, 88.47553407664152303 ) ) ;
#10233=FACE_OUTER_BOUND ( 'NONE', #2303, .T. ) ;
#10235=CARTESIAN_POINT ( 'NONE',  ( 36.35000000109246798, 13.62011893735970958, 86.15790661882942914 ) ) ;
#10236=CARTESIAN_POINT ( 'NONE',  ( 32.25000000109245946, 12.86707612778636012, 88.47553407664152303 ) ) ;
#10238=CARTESIAN_POINT ( 'NONE',  ( 25.47500000054622760, 26.19570976099943493, 95.29460816699764791 ) ) ;
#10239=CARTESIAN_POINT ( 'NONE',  ( 27.07500000054622546, 24.28113015263587471, 84.90069139318163138 ) ) ;
#10241=CARTESIAN_POINT ( 'NONE',  ( 20.27158385259951956, 22.00000000000000000, 170.0000119999999697 ) ) ;
#10243=VECTOR ( 'NONE', #11148, 1000.000000000000000 ) ;
#10244=CARTESIAN_POINT ( 'NONE',  ( 42.85000000109246798, 24.40838939219355197, 84.72553407664153724 ) ) ;
#10250=CARTESIAN_POINT ( 'NONE',  ( 20.27500000054623186, 12.34168156654572535, 90.79316153445363113 ) ) ;
#10253=ADVANCED_FACE ( 'NONE', ( #7916 ), #4169, .F. ) ;
#10259=CARTESIAN_POINT ( 'NONE',  ( 49.99999999999998579, 20.00000000000000355, 90.79316153445363113 ) ) ;
#10260=CARTESIAN_POINT ( 'NONE',  ( 47.65000000109246514, 20.00000000000000355, 98.29316153445363113 ) ) ;
#10261=CARTESIAN_POINT ( 'NONE',  ( 39.57500000054623257, 26.19570976099943493, 95.29460816699764791 ) ) ;
#10262=AXIS2_PLACEMENT_3D ( 'NONE', #19, #4710, #82 ) ;
#10263=CARTESIAN_POINT ( 'NONE',  ( 25.17500000054623044, 26.92701409722686634, 88.54243821818162985 ) ) ;
#10264=CARTESIAN_POINT ( 'NONE',  ( 6.614374549531869540, 12.49999671209873497, 91.04913669327301307 ) ) ;
#10265=CARTESIAN_POINT ( 'NONE',  ( 22.65000000109246514, 20.00000000000000355, 83.29316153445364534 ) ) ;
#10266=CARTESIAN_POINT ( 'NONE',  ( -2.000000000000015543, 20.00000000000000355, 90.79316153445363113 ) ) ;
#10267=CARTESIAN_POINT ( 'NONE',  ( 31.09999999999998721, 22.43689772174679575, 83.29316153445363113 ) ) ;
#10273=CARTESIAN_POINT ( 'NONE',  ( 31.67500000054622333, 24.28113015263587116, 96.68563167572563088 ) ) ;
#10274=CARTESIAN_POINT ( 'NONE',  ( 27.65000000109246514, 20.00000000000000355, 98.29316153445363113 ) ) ;
#10275=CARTESIAN_POINT ( 'NONE',  ( 47.37500000054622973, 26.92701409722686634, 93.04388485072563242 ) ) ;
#10276=CARTESIAN_POINT ( 'NONE',  ( 35.57500000054623257, 26.19570976099943493, 95.29460816699764791 ) ) ;
#10277=CARTESIAN_POINT ( 'NONE',  ( 37.59999999999998721, 27.13292387221364876, 93.11078899226573924 ) ) ;
#10279=EDGE_CURVE ( 'NONE', #707, #10641, #2149, .T. ) ;
#10280=CARTESIAN_POINT ( 'NONE',  ( 37.47500000054623825, 26.19570976099943493, 95.29460816699764791 ) ) ;
#10281=ORIENTED_EDGE ( 'NONE', *, *, #6802, .F. ) ;
#10282=CARTESIAN_POINT ( 'NONE',  ( 21.15000000109246514, 27.88596668178699645, 90.79316153445363113 ) ) ;
#10283=CARTESIAN_POINT ( 'NONE',  ( -50.00000000000001421, 55.00000000000000000, 166.8533255156881694 ) ) ;
#10287=( BOUNDED_CURVE ( )  B_SPLINE_CURVE ( 2, ( #11497, #10352, #12452, #4709, #6548, #11314, #6730, #6606, #5732, #2870, #4523 ),
 .UNSPECIFIED., .F., .F. ) 
 B_SPLINE_CURVE_WITH_KNOTS ( ( 3, 2, 2, 2, 2, 3 ),
 ( 0.9666666666666666741, 0.9733333333333333837, 0.9799999999999999822, 0.9866666666666666918, 0.9933333333333332904, 1.000000000000000000 ),
 .UNSPECIFIED. ) 
 CURVE ( )  GEOMETRIC_REPRESENTATION_ITEM ( )  RATIONAL_B_SPLINE_CURVE ( ( 1.000000000000000000, 0.9510565162951535312, 1.000000000000000000, 0.9510565162951535312, 1.000000000000000000, 0.9510565162951535312, 1.000000000000000000, 0.9510565162951535312, 1.000000000000000000, 0.9510565162951535312, 1.000000000000000000 ) ) 
 REPRESENTATION_ITEM ( '' )  );
#10290=CARTESIAN_POINT ( 'NONE',  ( 4.999999999999999112, 22.00000000000000000, 169.9999999999999716 ) ) ;
#10291=CARTESIAN_POINT ( 'NONE',  ( 25.89999999999998792, 22.43689772174679575, 98.29316153445363113 ) ) ;
#10292=CARTESIAN_POINT ( 'NONE',  ( 24.17500000054622689, 13.07298590277314254, 93.04388485072563242 ) ) ;
#10293=CARTESIAN_POINT ( 'NONE',  ( 25.97500000054622049, 17.63344945572769973, 98.07665518445361386 ) ) ;
#10294=DIRECTION ( 'NONE',  ( 0.000000000000000000, 0.000000000000000000, 1.000000000000000000 ) ) ;
#10295=CARTESIAN_POINT ( 'NONE',  ( -2.000000000000015543, 20.00000000000000355, 83.29316153445364534 ) ) ;
#10297=VERTEX_POINT ( 'NONE', #5128 ) ;
#10298=CARTESIAN_POINT ( 'NONE',  ( 36.35000000109246798, 13.62011893735971135, 86.15790661882942914 ) ) ;
#10300=VERTEX_POINT ( 'NONE', #11722 ) ;
#10301=LINE ( 'NONE', #3578, #8292 ) ;
#10308=CARTESIAN_POINT ( 'NONE',  ( 4.999999999999999112, 0.000000000000000000, 169.9999999999999716 ) ) ;
#10309=CARTESIAN_POINT ( 'NONE',  ( 42.09999999999997300, 17.56310227825320425, 98.29316153445363113 ) ) ;
#10311=CARTESIAN_POINT ( 'NONE',  ( 27.77500000054622831, 20.00000000000000355, 98.07665518445361386 ) ) ;
#10313=CARTESIAN_POINT ( 'NONE',  ( 46.65000000109246514, 20.00000000000000355, 83.29316153445364534 ) ) ;
#10317=EDGE_CURVE ( 'NONE', #10297, #4126, #3975, .T. ) ;
#10319=CARTESIAN_POINT ( 'NONE',  ( 37.77500000054623541, 20.00000000000000355, 98.07665518445361386 ) ) ;
#10320=CARTESIAN_POINT ( 'NONE',  ( 38.87500000054622262, 20.00000000000000355, 83.50966788445364841 ) ) ;
#10321=CARTESIAN_POINT ( 'NONE',  ( 29.17500000054623044, 26.92701409722686634, 88.54243821818162985 ) ) ;
#10322=CARTESIAN_POINT ( 'NONE',  ( 6.732675160020738403, 12.60562763040432621, 89.51398028008233609 ) ) ;
#10324=DIRECTION ( 'NONE',  ( 1.000000000000000000, -0.000000000000000000, -0.000000000000000000 ) ) ;
#10325=DIRECTION ( 'NONE',  ( 1.000000000000000000, -0.000000000000000000, -0.000000000000000000 ) ) ;
#10326=EDGE_CURVE ( 'NONE', #223, #11822, #11151, .T. ) ;
#10330=VECTOR ( 'NONE', #2030, 1000.000000000000000 ) ;
#10331=DIRECTION ( 'NONE',  ( -1.000000000000000000, 0.000000000000000000, -0.000000000000000000 ) ) ;
#10333=CARTESIAN_POINT ( 'NONE',  ( 35.17500000054621268, 26.19570976099943849, 86.29171490190961435 ) ) ;
#10334=CARTESIAN_POINT ( 'NONE',  ( 26.95000000109246585, 26.37988106264029398, 86.15790661882942914 ) ) ;
#10335=CARTESIAN_POINT ( 'NONE',  ( 46.17500000054623399, 13.07298590277314254, 93.04388485072563242 ) ) ;
#10336=CARTESIAN_POINT ( 'NONE',  ( 36.37500000054623683, 12.34168156654572535, 90.79316153445363113 ) ) ;
#10337=CARTESIAN_POINT ( 'NONE',  ( 30.19999999999998863, 15.59161060780645691, 96.86078899226572503 ) ) ;
#10340=CARTESIAN_POINT ( 'NONE',  ( 40.67500000054623399, 17.63344945572770328, 83.50966788445364841 ) ) ;
#10342=CARTESIAN_POINT ( 'NONE',  ( 49.57500000054623257, 24.28113015263587116, 96.68563167572563088 ) ) ;
#10343=CARTESIAN_POINT ( 'NONE',  ( 27.85000000109246443, 15.59161060780645691, 96.86078899226572503 ) ) ;
#10346=EDGE_LOOP ( 'NONE', ( #6677, #24 ) ) ;
#10351=EDGE_CURVE ( 'NONE', #9812, #5818, #11848, .T. ) ;
#10352=CARTESIAN_POINT ( 'NONE',  ( 20.89999999999999147, 17.56310227825320425, 83.29316153445363113 ) ) ;
#10353=CARTESIAN_POINT ( 'NONE',  ( 24.47500000054623115, 13.80429023900056684, 86.29171490190961435 ) ) ;
#10354=CARTESIAN_POINT ( 'NONE',  ( 21.87500000054622618, 20.00000000000000355, 98.07665518445361386 ) ) ;
#10357=DIRECTION ( 'NONE',  ( 1.000000000000000000, -0.000000000000000000, -0.000000000000000000 ) ) ;
#10359=CARTESIAN_POINT ( 'NONE',  ( 35.45000000109246940, 24.40838939219354842, 96.86078899226572503 ) ) ;
#10360=CARTESIAN_POINT ( 'NONE',  ( 24.99999999999998579, 20.00000000000000355, 83.29316153445364534 ) ) ;
#10362=CARTESIAN_POINT ( 'NONE',  ( 47.79999999999999005, 24.40838939219354842, 96.86078899226572503 ) ) ;
#10364=CARTESIAN_POINT ( 'NONE',  ( -50.00000000000001421, 55.00000000000000000, 124.8533255156881694 ) ) ;
#10373=CARTESIAN_POINT ( 'NONE',  ( 20.77500000054622831, 20.00000000000000355, 83.50966788445364841 ) ) ;
#10374=DIRECTION ( 'NONE',  ( 1.000000000000000000, -0.000000000000000000, -0.000000000000000000 ) ) ;
#10378=VECTOR ( 'NONE', #4260, 1000.000000000000000 ) ;
#10381=CARTESIAN_POINT ( 'NONE',  ( 39.77500000054622831, 20.00000000000000355, 98.07665518445361386 ) ) ;
#10382=CARTESIAN_POINT ( 'NONE',  ( 40.37500000054621552, 12.34168156654572535, 90.79316153445363113 ) ) ;
#10385=CARTESIAN_POINT ( 'NONE',  ( 20.77500000054622831, 20.00000000000000355, 83.50966788445364841 ) ) ;
#10386=CARTESIAN_POINT ( 'NONE',  ( 10.00000000000000355, 20.00000000000000355, 69.99999999999998579 ) ) ;
#10387=CARTESIAN_POINT ( 'NONE',  ( -50.00000000000001421, 18.00000000000000355, 188.4007504869563263 ) ) ;
#10389=CARTESIAN_POINT ( 'NONE',  ( 35.89999999999999147, 22.43689772174678154, 98.29316153445364534 ) ) ;
#10394=LINE ( 'NONE', #2725, #5306 ) ;
#10396=VECTOR ( 'NONE', #249, 1000.000000000000000 ) ;
#10398=CARTESIAN_POINT ( 'NONE',  ( 27.45000000109246585, 24.40838939219354842, 96.86078899226572503 ) ) ;
#10399=CARTESIAN_POINT ( 'NONE',  ( 37.07500000054621836, 26.19570976099943849, 86.29171490190961435 ) ) ;
#10400=CARTESIAN_POINT ( 'NONE',  ( 30.77500000054621765, 17.63344945572770328, 83.50966788445364841 ) ) ;
#10401=CARTESIAN_POINT ( 'NONE',  ( 30.89999999999998437, 17.56310227825321135, 83.29316153445363113 ) ) ;
#10403=CARTESIAN_POINT ( 'NONE',  ( 41.77500000054622831, 20.00000000000000355, 98.07665518445361386 ) ) ;
#10405=CARTESIAN_POINT ( 'NONE',  ( 20.75000000109246656, 22.43689772174679575, 83.29316153445363113 ) ) ;
#10408=AXIS2_PLACEMENT_3D ( 'NONE', #7951, #5983, #22 ) ;
#10412=CARTESIAN_POINT ( 'NONE',  ( 23.10660171779821326, 27.49999999999999645, 140.6066017177982133 ) ) ;
#10413=DIRECTION ( 'NONE',  ( 1.000000000000000000, -0.000000000000000000, -0.000000000000000000 ) ) ;
#10414=CARTESIAN_POINT ( 'NONE',  ( 42.87500000054622262, 20.00000000000000355, 83.50966788445364841 ) ) ;
#10416=CARTESIAN_POINT ( 'NONE',  ( 46.37500000054621552, 12.34168156654572535, 90.79316153445363113 ) ) ;
#10417=CARTESIAN_POINT ( 'NONE',  ( 46.39999999999999147, 12.86707612778636012, 93.11078899226572503 ) ) ;
#10418=CIRCLE ( 'NONE', #1115, 7.499999999999978684 ) ;
#10420=CARTESIAN_POINT ( 'NONE',  ( 39.65000000109246514, 20.00000000000000355, 98.29316153445363113 ) ) ;
#10422=CARTESIAN_POINT ( 'NONE',  ( 34.75000000109245235, 22.43689772174679575, 83.29316153445363113 ) ) ;
#10424=CARTESIAN_POINT ( 'NONE',  ( -2.000000000000015543, 20.00000000000000355, 90.79316153445363113 ) ) ;
#10429=CARTESIAN_POINT ( 'NONE',  ( -50.00000000000001421, 20.00000000000000000, 145.0000000000000000 ) ) ;
#10433=DIRECTION ( 'NONE',  ( 0.000000000000000000, 1.000000000000000000, 0.000000000000000000 ) ) ;
#10435=CARTESIAN_POINT ( 'NONE',  ( 20.87500000054622973, 22.36655054427230382, 83.50966788445364841 ) ) ;
#10439=ORIENTED_EDGE ( 'NONE', *, *, #4904, .T. ) ;
#10443=CARTESIAN_POINT ( 'NONE',  ( 35.17500000054621268, 26.19570976099943493, 86.29171490190961435 ) ) ;
#10444=CARTESIAN_POINT ( 'NONE',  ( 23.07500000054622902, 26.19570976099943849, 86.29171490190961435 ) ) ;
#10445=DIRECTION ( 'NONE',  ( 0.000000000000000000, 0.000000000000000000, 1.000000000000000000 ) ) ;
#10456=CARTESIAN_POINT ( 'NONE',  ( 24.47500000054622404, 13.07298590277314432, 88.54243821818161564 ) ) ;
#10457=CARTESIAN_POINT ( 'NONE',  ( 36.39999999999999147, 12.86707612778636012, 93.11078899226572503 ) ) ;
#10458=CARTESIAN_POINT ( 'NONE',  ( 42.47500000054622404, 13.80429023900056684, 86.29171490190961435 ) ) ;
#10459=CARTESIAN_POINT ( 'NONE',  ( 28.27500000054622475, 13.07298590277314254, 93.04388485072563242 ) ) ;
#10460=CARTESIAN_POINT ( 'NONE',  ( 28.19999999999998863, 15.59161060780645691, 96.86078899226572503 ) ) ;
#10462=CARTESIAN_POINT ( 'NONE',  ( 37.17500000054622689, 26.92701409722686634, 88.54243821818162985 ) ) ;
#10463=ORIENTED_EDGE ( 'NONE', *, *, #8117, .T. ) ;
#10464=CARTESIAN_POINT ( 'NONE',  ( 47.77500000054622831, 20.00000000000000355, 98.07665518445361386 ) ) ;
#10472=CYLINDRICAL_SURFACE ( 'NONE', #9649, 7.499999999999992895 ) ;
#10474=CARTESIAN_POINT ( 'NONE',  ( 44.67500000054621978, 15.71886984736413773, 84.90069139318163138 ) ) ;
#10478=FACE_OUTER_BOUND ( 'NONE', #8608, .T. ) ;
#10479=CARTESIAN_POINT ( 'NONE',  ( 43.07500000054622546, 24.28113015263587471, 84.90069139318163138 ) ) ;
#10480=CARTESIAN_POINT ( 'NONE',  ( 20.27500000054622475, 13.07298590277314254, 93.04388485072563242 ) ) ;
#10481=DIRECTION ( 'NONE',  ( 0.000000000000000000, 0.000000000000000000, -1.000000000000000000 ) ) ;
#10482=DIRECTION ( 'NONE',  ( 0.000000000000000000, 0.000000000000000000, -1.000000000000000000 ) ) ;
#10483=ORIENTED_EDGE ( 'NONE', *, *, #6380, .T. ) ;
#10484=CARTESIAN_POINT ( 'NONE',  ( 35.05000000109246372, 27.13292387221364876, 88.47553407664153724 ) ) ;
#10488=ADVANCED_FACE ( 'NONE', ( #975 ), #6863, .F. ) ;
#10491=CYLINDRICAL_SURFACE ( 'NONE', #8262, 7.499999999999978684 ) ;
#10499=FACE_OUTER_BOUND ( 'NONE', #12276, .T. ) ;
#10500=CARTESIAN_POINT ( 'NONE',  ( 22.87500000054623328, 22.36655054427230382, 83.50966788445364841 ) ) ;
#10504=VERTEX_POINT ( 'NONE', #1910 ) ;
#10507=CARTESIAN_POINT ( 'NONE',  ( -50.00000000000001421, 18.00000000000000355, 169.9999999999999716 ) ) ;
#10509=MECHANICAL_DESIGN_GEOMETRIC_PRESENTATION_REPRESENTATION('',(#1005),#8290);
#10510=DIRECTION ( 'NONE',  ( -1.000000000000000000, 0.000000000000000000, 0.000000000000000000 ) ) ;
#10515=ORIENTED_EDGE ( 'NONE', *, *, #7992, .F. ) ;
#10518=CARTESIAN_POINT ( 'NONE',  ( 27.27500000054622475, 26.92701409722686634, 88.54243821818162985 ) ) ;
#10519=CARTESIAN_POINT ( 'NONE',  ( 28.85000000109246443, 24.40838939219355197, 84.72553407664153724 ) ) ;
#10520=CARTESIAN_POINT ( 'NONE',  ( 42.37500000054622262, 13.07298590277314432, 88.54243821818161564 ) ) ;
#10521=CARTESIAN_POINT ( 'NONE',  ( 30.47500000054622404, 13.07298590277314432, 88.54243821818161564 ) ) ;
#10522=CARTESIAN_POINT ( 'NONE',  ( 32.29999999999999005, 13.62011893735971135, 95.42841645007781892 ) ) ;
#10524=CARTESIAN_POINT ( 'NONE',  ( -50.00000000000001421, 0.000000000000000000, 121.2488769092545198 ) ) ;
#10525=CARTESIAN_POINT ( 'NONE',  ( 31.27500000054622831, 27.65831843345427998, 90.79316153445363113 ) ) ;
#10526=VERTEX_POINT ( 'NONE', #3881 ) ;
#10528=CARTESIAN_POINT ( 'NONE',  ( 48.67500000054623399, 17.63344945572770328, 83.50966788445364841 ) ) ;
#10529=CARTESIAN_POINT ( 'NONE',  ( 28.15000000109246159, 12.11403331821300533, 90.79316153445363113 ) ) ;
#10530=EDGE_LOOP ( 'NONE', ( #999, #8465, #10626, #9069, #3242 ) ) ;
#10536=CARTESIAN_POINT ( 'NONE',  ( 32.09999999999998721, 17.56310227825320425, 98.29316153445363113 ) ) ;
#10538=VECTOR ( 'NONE', #3983, 1000.000000000000000 ) ;
#10539=CARTESIAN_POINT ( 'NONE',  ( 47.37500000054622262, 27.65831843345427998, 90.79316153445363113 ) ) ;
#10542=CARTESIAN_POINT ( 'NONE',  ( 42.57500000054622546, 13.80429023900056684, 86.29171490190961435 ) ) ;
#10543=CARTESIAN_POINT ( 'NONE',  ( 19.97500000054622404, 17.63344945572769973, 98.07665518445361386 ) ) ;
#10545=CARTESIAN_POINT ( 'NONE',  ( 0.000000000000000000, 20.00000000000000355, 109.9999999999999858 ) ) ;
#10547=CARTESIAN_POINT ( 'NONE',  ( 39.05000000109247082, 27.13292387221364876, 88.47553407664153724 ) ) ;
#10549=EDGE_LOOP ( 'NONE', ( #2702, #1999, #1037, #10981, #6853 ) ) ;
#10551=VECTOR ( 'NONE', #6856, 1000.000000000000000 ) ;
#10552=EDGE_CURVE ( 'NONE', #1942, #7750, #6671, .T. ) ;
#10553=ORIENTED_EDGE ( 'NONE', *, *, #9100, .F. ) ;
#10557=ADVANCED_FACE ( 'NONE', ( #10478 ), #7634, .F. ) ;
#10562=CARTESIAN_POINT ( 'NONE',  ( 47.75000000109246656, 17.56310227825322556, 98.29316153445364534 ) ) ;
#10563=CARTESIAN_POINT ( 'NONE',  ( 21.97500000054622760, 15.71886984736413417, 96.68563167572563088 ) ) ;
#10565=CARTESIAN_POINT ( 'NONE',  ( 45.95000000109245519, 13.62011893735970958, 95.42841645007781892 ) ) ;
#10567=ORIENTED_EDGE ( 'NONE', *, *, #1653, .T. ) ;
#10568=ORIENTED_EDGE ( 'NONE', *, *, #1801, .F. ) ;
#10577=DIRECTION ( 'NONE',  ( -0.000000000000000000, -0.000000000000000000, 1.000000000000000000 ) ) ;
#10578=CARTESIAN_POINT ( 'NONE',  ( -2.000000000000015543, 20.00000000000000355, 90.79316153445363113 ) ) ;
#10582=CARTESIAN_POINT ( 'NONE',  ( 47.87500000054622262, 20.00000000000000355, 98.07665518445361386 ) ) ;
#10584=CARTESIAN_POINT ( 'NONE',  ( 39.07500000054621836, 26.19570976099943849, 86.29171490190961435 ) ) ;
#10585=CARTESIAN_POINT ( 'NONE',  ( 30.57500000054622191, 13.80429023900056684, 86.29171490190961435 ) ) ;
#10586=CARTESIAN_POINT ( 'NONE',  ( 31.59999999999999076, 27.13292387221364876, 93.11078899226573924 ) ) ;
#10587=CARTESIAN_POINT ( 'NONE',  ( 30.57500000054622902, 15.71886984736413773, 84.90069139318163138 ) ) ;
#10588=ORIENTED_EDGE ( 'NONE', *, *, #396, .T. ) ;
#10590=VERTEX_POINT ( 'NONE', #2039 ) ;
#10594=CARTESIAN_POINT ( 'NONE',  ( 32.79999999999999005, 15.59161060780646046, 84.72553407664153724 ) ) ;
#10595=LINE ( 'NONE', #2035, #2584 ) ;
#10596=CARTESIAN_POINT ( 'NONE',  ( 47.17500000054622689, 26.19570976099943849, 86.29171490190961435 ) ) ;
#10597=CARTESIAN_POINT ( 'NONE',  ( 41.65000000109246514, 20.00000000000000355, 98.29316153445363113 ) ) ;
#10598=CARTESIAN_POINT ( 'NONE',  ( 21.47500000054622404, 26.92701409722686634, 93.04388485072563242 ) ) ;
#10599=VECTOR ( 'NONE', #2885, 1000.000000000000000 ) ;
#10600=CARTESIAN_POINT ( 'NONE',  ( 45.19999999999998863, 24.40838939219355197, 84.72553407664153724 ) ) ;
#10604=CARTESIAN_POINT ( 'NONE',  ( 34.15000000109245804, 12.11403331821300533, 90.79316153445363113 ) ) ;
#10605=CARTESIAN_POINT ( 'NONE',  ( -20.00000000000001776, 20.00000000000000000, 137.5000000000000000 ) ) ;
#10606=ORIENTED_EDGE ( 'NONE', *, *, #11334, .F. ) ;
#10607=CARTESIAN_POINT ( 'NONE',  ( -5.000000000000000888, 22.00000000000000000, 218.7511230907454944 ) ) ;
#10609=LINE ( 'NONE', #9554, #4243 ) ;
#10614=( BOUNDED_CURVE ( )  B_SPLINE_CURVE ( 3, ( #5708, #7480, #6772, #9637 ),
 .UNSPECIFIED., .F., .F. ) 
 B_SPLINE_CURVE_WITH_KNOTS ( ( 4, 4 ),
 ( 0.000000000000000000, 1.570796326794896558 ),
 .UNSPECIFIED. ) 
 CURVE ( )  GEOMETRIC_REPRESENTATION_ITEM ( )  RATIONAL_B_SPLINE_CURVE ( ( 1.000000000000000000, 0.8047378541243649375, 0.8047378541243649375, 1.000000000000000000 ) ) 
 REPRESENTATION_ITEM ( '' )  );
#10615=CARTESIAN_POINT ( 'NONE',  ( 40.17500000054623399, 13.07298590277314254, 93.04388485072563242 ) ) ;
#10616=CARTESIAN_POINT ( 'NONE',  ( 35.15000000109246514, 27.88596668178699645, 90.79316153445363113 ) ) ;
#10617=DIRECTION ( 'NONE',  ( 0.000000000000000000, 0.000000000000000000, 1.000000000000000000 ) ) ;
#10618=CARTESIAN_POINT ( 'NONE',  ( 34.35000000109246798, 13.62011893735970958, 86.15790661882942914 ) ) ;
#10621=DIRECTION ( 'NONE',  ( 1.000000000000000000, -0.000000000000000000, -0.000000000000000000 ) ) ;
#10622=CARTESIAN_POINT ( 'NONE',  ( 22.97500000054622760, 24.28113015263587471, 84.90069139318163138 ) ) ;
#10623=ORIENTED_EDGE ( 'NONE', *, *, #1765, .T. ) ;
#10625=DIRECTION ( 'NONE',  ( 1.000000000000000000, 0.000000000000000000, 0.000000000000000000 ) ) ;
#10626=ORIENTED_EDGE ( 'NONE', *, *, #6521, .F. ) ;
#10629=ORIENTED_EDGE ( 'NONE', *, *, #1474, .T. ) ;
#10630=FACE_OUTER_BOUND ( 'NONE', #12348, .T. ) ;
#10631=CARTESIAN_POINT ( 'NONE',  ( -27.49999999999999645, 12.50000000000001066, 145.0000000000000000 ) ) ;
#10633=EDGE_CURVE ( 'NONE', #1127, #9352, #6923, .T. ) ;
#10635=FACE_OUTER_BOUND ( 'NONE', #7371, .T. ) ;
#10637=PLANE ( 'NONE',  #5341 ) ;
#10639=VECTOR ( 'NONE', #7878, 1000.000000000000000 ) ;
#10641=VERTEX_POINT ( 'NONE', #8077 ) ;
#10645=CARTESIAN_POINT ( 'NONE',  ( 23.65000000109246514, 20.00000000000000355, 98.29316153445363113 ) ) ;
#10646=VECTOR ( 'NONE', #1163, 1000.000000000000000 ) ;
#10647=CARTESIAN_POINT ( 'NONE',  ( 37.47500000054623115, 26.19570976099943849, 95.29460816699764791 ) ) ;
#10648=CARTESIAN_POINT ( 'NONE',  ( 30.37500000054622618, 12.34168156654572535, 90.79316153445363113 ) ) ;
#10649=CARTESIAN_POINT ( 'NONE',  ( 22.89999999999998792, 17.56310227825321135, 83.29316153445363113 ) ) ;
#10650=DIRECTION ( 'NONE',  ( 1.000000000000000000, -0.000000000000000000, -0.000000000000000000 ) ) ;
#10651=CARTESIAN_POINT ( 'NONE',  ( 32.47500000054623825, 13.80429023900056684, 86.29171490190961435 ) ) ;
#10652=ORIENTED_EDGE ( 'NONE', *, *, #2428, .T. ) ;
#10653=ADVANCED_FACE ( 'NONE', ( #4005 ), #9917, .F. ) ;
#10657=ORIENTED_EDGE ( 'NONE', *, *, #5886, .F. ) ;
#10660=FACE_OUTER_BOUND ( 'NONE', #266, .T. ) ;
#10661=CARTESIAN_POINT ( 'NONE',  ( 43.97500000054622404, 17.63344945572769973, 98.07665518445361386 ) ) ;
#10665=CARTESIAN_POINT ( 'NONE',  ( 44.57500000054622546, 13.80429023900056684, 86.29171490190961435 ) ) ;
#10666=CARTESIAN_POINT ( 'NONE',  ( 40.09999999999998721, 17.56310227825320425, 98.29316153445363113 ) ) ;
#10668=CARTESIAN_POINT ( 'NONE',  ( 40.59999999999998721, 12.86707612778636012, 88.47553407664152303 ) ) ;
#10671=CARTESIAN_POINT ( 'NONE',  ( 34.45000000109246940, 15.59161060780646046, 84.72553407664153724 ) ) ;
#10672=CARTESIAN_POINT ( 'NONE',  ( -6.999999999999999112, 92.00000000000000000, 69.99999999999998579 ) ) ;
#10674=ORIENTED_EDGE ( 'NONE', *, *, #1701, .T. ) ;
#10676=AXIS2_PLACEMENT_3D ( 'NONE', #5147, #1518, #9013 ) ;
#10678=CARTESIAN_POINT ( 'NONE',  ( -2.000000000000015543, 20.00000000000000355, 98.29316153445363113 ) ) ;
#10679=CARTESIAN_POINT ( 'NONE',  ( 33.97500000054623115, 15.71886984736413417, 96.68563167572563088 ) ) ;
#10680=CARTESIAN_POINT ( 'NONE',  ( 37.97500000054621694, 17.63344945572769973, 98.07665518445361386 ) ) ;
#10681=CARTESIAN_POINT ( 'NONE',  ( 35.25000000109245946, 27.13292387221364876, 93.11078899226573924 ) ) ;
#10682=CARTESIAN_POINT ( 'NONE',  ( 43.75000000109248077, 17.56310227825318648, 98.29316153445363113 ) ) ;
#10684=EDGE_CURVE ( 'NONE', #852, #1585, #5635, .T. ) ;
#10687=ORIENTED_EDGE ( 'NONE', *, *, #1724, .T. ) ;
#10690=VERTEX_POINT ( 'NONE', #8829 ) ;
#10691=EDGE_CURVE ( 'NONE', #9799, #6453, #2966, .T. ) ;
#10692=( BOUNDED_CURVE ( )  B_SPLINE_CURVE ( 2, ( #10043, #1354, #5220, #12435, #9524, #8624, #10457, #2730, #4692, #2788, #6650 ),
 .UNSPECIFIED., .F., .F. ) 
 B_SPLINE_CURVE_WITH_KNOTS ( ( 3, 2, 2, 2, 2, 3 ),
 ( 0.4333333333333332926, 0.4399999999999999467, 0.4466666666666666008, 0.4533333333333332549, 0.4599999999999999645, 0.4666666666666666186 ),
 .UNSPECIFIED. ) 
 CURVE ( )  GEOMETRIC_REPRESENTATION_ITEM ( )  RATIONAL_B_SPLINE_CURVE ( ( 1.000000000000000444, 0.9510565162951531981, 1.000000000000000000, 0.9510565162951535312, 1.000000000000000000, 0.9510565162951535312, 1.000000000000000000, 0.9510565162951535312, 1.000000000000000000, 0.9510565162951539753, 0.9999999999999995559 ) ) 
 REPRESENTATION_ITEM ( '' )  );
#10694=CARTESIAN_POINT ( 'NONE',  ( 42.75000000109245235, 22.43689772174680641, 83.29316153445363113 ) ) ;
#10695=DIRECTION ( 'NONE',  ( 1.000000000000000000, -0.000000000000000000, -0.000000000000000000 ) ) ;
#10696=CARTESIAN_POINT ( 'NONE',  ( 8.353307965316590256, 25.50093297180406182, 95.89657251760699808 ) ) ;
#10697=CARTESIAN_POINT ( 'NONE',  ( 37.99999999999999289, 20.00000000000000355, 98.29316153445363113 ) ) ;
#10699=CARTESIAN_POINT ( 'NONE',  ( -20.27158385259951601, 22.00000000000000000, 169.9999999999999716 ) ) ;
#10701=AXIS2_PLACEMENT_3D ( 'NONE', #11979, #433, #8296 ) ;
#10704=CARTESIAN_POINT ( 'NONE',  ( 36.65000000109245804, 20.00000000000000355, 83.29316153445364534 ) ) ;
#10707=VECTOR ( 'NONE', #5780, 1000.000000000000000 ) ;
#10708=CARTESIAN_POINT ( 'NONE',  ( 23.47500000054622404, 26.92701409722686634, 93.04388485072563242 ) ) ;
#10709=CARTESIAN_POINT ( 'NONE',  ( 49.47500000054623115, 26.92701409722686634, 93.04388485072563242 ) ) ;
#10710=CARTESIAN_POINT ( 'NONE',  ( 34.27500000054622831, 12.34168156654572357, 90.79316153445363113 ) ) ;
#10712=CARTESIAN_POINT ( 'NONE',  ( 24.27500000054622475, 13.07298590277314254, 93.04388485072563242 ) ) ;
#10713=CARTESIAN_POINT ( 'NONE',  ( 23.69999999999998508, 26.37988106264029398, 95.42841645007781892 ) ) ;
#10714=CARTESIAN_POINT ( 'NONE',  ( 34.79999999999999005, 15.59161060780646046, 84.72553407664153724 ) ) ;
#10715=CARTESIAN_POINT ( 'NONE',  ( 35.87500000054622262, 17.63344945572769973, 98.07665518445361386 ) ) ;
#10718=ORIENTED_EDGE ( 'NONE', *, *, #7602, .F. ) ;
#10719=CARTESIAN_POINT ( 'NONE',  ( 49.15000000109245804, 27.88596668178699645, 90.79316153445363113 ) ) ;
#10724=CARTESIAN_POINT ( 'NONE',  ( 41.47500000054623115, 26.92701409722686634, 93.04388485072563242 ) ) ;
#10727=CARTESIAN_POINT ( 'NONE',  ( 42.27500000054622120, 13.07298590277314254, 93.04388485072563242 ) ) ;
#10728=CARTESIAN_POINT ( 'NONE',  ( 40.99999999999998579, 20.00000000000000355, 83.29316153445364534 ) ) ;
#10730=CARTESIAN_POINT ( 'NONE',  ( 40.29999999999997584, 13.62011893735970958, 95.42841645007781892 ) ) ;
#10733=CARTESIAN_POINT ( 'NONE',  ( 32.15000000109246514, 12.11403331821300533, 90.79316153445363113 ) ) ;
#10741=DIRECTION ( 'NONE',  ( 1.000000000000000000, -0.000000000000000000, -0.000000000000000000 ) ) ;
#10742=CARTESIAN_POINT ( 'NONE',  ( 36.87500000054622973, 22.36655054427230382, 83.50966788445364841 ) ) ;
#10743=CARTESIAN_POINT ( 'NONE',  ( 34.67500000054622689, 15.71886984736413773, 84.90069139318163138 ) ) ;
#10748=CARTESIAN_POINT ( 'NONE',  ( 47.95000000109246230, 13.62011893735971135, 95.42841645007781892 ) ) ;
#10750=ORIENTED_EDGE ( 'NONE', *, *, #10317, .F. ) ;
#10752=ORIENTED_EDGE ( 'NONE', *, *, #1189, .T. ) ;
#10754=VERTEX_POINT ( 'NONE', #943 ) ;
#10755=VECTOR ( 'NONE', #9335, 1000.000000000000114 ) ;
#10758=CARTESIAN_POINT ( 'NONE',  ( 8.665435081250036475, 25.00622661766839627, 96.39744239336449994 ) ) ;
#10759=CARTESIAN_POINT ( 'NONE',  ( 37.19999999999998863, 24.40838939219355197, 84.72553407664153724 ) ) ;
#10763=CARTESIAN_POINT ( 'NONE',  ( 43.37500000054622973, 26.92701409722686634, 93.04388485072563242 ) ) ;
#10765=ORIENTED_EDGE ( 'NONE', *, *, #1134, .F. ) ;
#10771=CARTESIAN_POINT ( 'NONE',  ( 49.17500000054622689, 26.19570976099943493, 86.29171490190961435 ) ) ;
#10772=CARTESIAN_POINT ( 'NONE',  ( 32.07500000054623257, 13.80429023900056507, 95.29460816699764791 ) ) ;
#10773=CARTESIAN_POINT ( 'NONE',  ( 22.37500000054622262, 12.34168156654572535, 90.79316153445363113 ) ) ;
#10774=CARTESIAN_POINT ( 'NONE',  ( 25.69999999999998508, 26.37988106264029398, 95.42841645007781892 ) ) ;
#10777=CARTESIAN_POINT ( 'NONE',  ( 33.97500000054623115, 15.71886984736413417, 96.68563167572563088 ) ) ;
#10778=EDGE_LOOP ( 'NONE', ( #12154, #1562, #4929, #8604 ) ) ;
#10783=EDGE_CURVE ( 'NONE', #10690, #3966, #8538, .T. ) ;
#10787=CARTESIAN_POINT ( 'NONE',  ( 41.17500000054621978, 26.19570976099943849, 86.29171490190961435 ) ) ;
#10788=CARTESIAN_POINT ( 'NONE',  ( 39.75000000109247367, 17.56310227825322556, 98.29316153445364534 ) ) ;
#10789=CARTESIAN_POINT ( 'NONE',  ( 25.99999999999998934, 20.00000000000000355, 98.29316153445363113 ) ) ;
#10790=CARTESIAN_POINT ( 'NONE',  ( 40.89999999999998437, 17.56310227825321135, 83.29316153445363113 ) ) ;
#10791=EDGE_CURVE ( 'NONE', #5818, #5150, #3914, .T. ) ;
#10797=CARTESIAN_POINT ( 'NONE',  ( 29.45000000109246230, 24.40838939219354842, 96.86078899226572503 ) ) ;
#10799=ORIENTED_EDGE ( 'NONE', *, *, #8392, .F. ) ;
#10801=CARTESIAN_POINT ( 'NONE',  ( 24.85000000109246443, 24.40838939219355197, 84.72553407664153724 ) ) ;
#10804=CARTESIAN_POINT ( 'NONE',  ( 28.17500000054622689, 13.07298590277314254, 93.04388485072563242 ) ) ;
#10805=CARTESIAN_POINT ( 'NONE',  ( 33.67500000054622689, 24.28113015263587116, 96.68563167572563088 ) ) ;
#10809=CARTESIAN_POINT ( 'NONE',  ( 34.15000000109245804, 12.11403331821300533, 90.79316153445363113 ) ) ;
#10812=DIRECTION ( 'NONE',  ( -0.000000000000000000, -1.000000000000000000, -0.000000000000000000 ) ) ;
#10813=ORIENTED_EDGE ( 'NONE', *, *, #9696, .F. ) ;
#10814=LINE ( 'NONE', #300, #7407 ) ;
#10819=DIRECTION ( 'NONE',  ( 0.000000000000000000, 0.000000000000000000, -1.000000000000000000 ) ) ;
#10821=CARTESIAN_POINT ( 'NONE',  ( 4.999999999999997335, 0.000000000000000000, 69.99999999999998579 ) ) ;
#10824=EDGE_CURVE ( 'NONE', #9224, #5074, #6514, .T. ) ;
#10826=VECTOR ( 'NONE', #2642, 1000.000000000000000 ) ;
#10830=CARTESIAN_POINT ( 'NONE',  ( 40.27500000054623541, 12.34168156654572535, 90.79316153445363113 ) ) ;
#10832=VERTEX_POINT ( 'NONE', #5000 ) ;
#10837=VECTOR ( 'NONE', #8469, 1000.000000000000000 ) ;
#10839=CARTESIAN_POINT ( 'NONE',  ( 22.37500000054622262, 12.34168156654572357, 90.79316153445363113 ) ) ;
#10841=CARTESIAN_POINT ( 'NONE',  ( 33.87500000054621552, 17.63344945572769973, 98.07665518445361386 ) ) ;
#10842=CARTESIAN_POINT ( 'NONE',  ( 20.17500000054622689, 13.80429023900056507, 95.29460816699764791 ) ) ;
#10843=CARTESIAN_POINT ( 'NONE',  ( 21.79999999999998650, 24.40838939219354842, 96.86078899226572503 ) ) ;
#10845=CARTESIAN_POINT ( 'NONE',  ( 49.09999999999998721, 22.43689772174678509, 83.29316153445363113 ) ) ;
#10846=CARTESIAN_POINT ( 'NONE',  ( 24.97500000054622760, 24.28113015263587471, 84.90069139318163138 ) ) ;
#10847=ORIENTED_EDGE ( 'NONE', *, *, #5232, .F. ) ;
#10849=EDGE_CURVE ( 'NONE', #10504, #9270, #9231, .T. ) ;
#10852=EDGE_LOOP ( 'NONE', ( #1797, #238, #5786, #7581, #10143 ) ) ;
#10855=ORIENTED_EDGE ( 'NONE', *, *, #8239, .F. ) ;
#10858=CARTESIAN_POINT ( 'NONE',  ( 38.37500000054622262, 12.34168156654572357, 90.79316153445363113 ) ) ;
#10860=CARTESIAN_POINT ( 'NONE',  ( 26.49999999999998934, 12.11403331821300533, 90.79316153445363113 ) ) ;
#10861=CARTESIAN_POINT ( 'NONE',  ( 41.27500000054622120, 26.92701409722686634, 88.54243821818162985 ) ) ;
#10862=CARTESIAN_POINT ( 'NONE',  ( 40.19999999999998863, 15.59161060780645691, 96.86078899226572503 ) ) ;
#10864=CARTESIAN_POINT ( 'NONE',  ( 49.77500000054622831, 20.00000000000000355, 98.07665518445361386 ) ) ;
#10865=VERTEX_POINT ( 'NONE', #2332 ) ;
#10866=CARTESIAN_POINT ( 'NONE',  ( 29.85000000109246443, 15.59161060780645691, 96.86078899226572503 ) ) ;
#10868=AXIS2_PLACEMENT_3D ( 'NONE', #9508, #6635, #1881 ) ;
#10869=EDGE_LOOP ( 'NONE', ( #10054, #6330, #7355, #6238, #8697 ) ) ;
#10873=CARTESIAN_POINT ( 'NONE',  ( -2.000000000000015543, 20.00000000000000355, 98.29316153445363113 ) ) ;
#10878=CARTESIAN_POINT ( 'NONE',  ( 32.57500000054623257, 15.71886984736413773, 84.90069139318163138 ) ) ;
#10879=CARTESIAN_POINT ( 'NONE',  ( 31.27500000054622831, 26.92701409722686634, 88.54243821818162985 ) ) ;
#10884=DIRECTION ( 'NONE',  ( 0.000000000000000000, 0.000000000000000000, -1.000000000000000000 ) ) ;
#10887=DIRECTION ( 'NONE',  ( 1.000000000000000000, 0.000000000000000000, 0.000000000000000000 ) ) ;
#10895=CIRCLE ( 'NONE', #12504, 7.499999999999978684 ) ;
#10896=CARTESIAN_POINT ( 'NONE',  ( 9.989996519715994339, 20.51596962592459406, 98.27983912618213935 ) ) ;
#10898=DIRECTION ( 'NONE',  ( 0.000000000000000000, -1.000000000000000000, -0.000000000000000000 ) ) ;
#10899=DIRECTION ( 'NONE',  ( 1.000000000000000000, -0.000000000000000000, -0.000000000000000000 ) ) ;
#10901=CARTESIAN_POINT ( 'NONE',  ( 41.77500000054622831, 20.00000000000000355, 98.07665518445361386 ) ) ;
#10905=LINE ( 'NONE', #8914, #11109 ) ;
#10906=EDGE_CURVE ( 'NONE', #9150, #3211, #11861, .T. ) ;
#10907=CARTESIAN_POINT ( 'NONE',  ( 21.27500000054622475, 26.92701409722686634, 88.54243821818162985 ) ) ;
#10908=CARTESIAN_POINT ( 'NONE',  ( 45.67500000054621978, 24.28113015263587116, 96.68563167572563088 ) ) ;
#10909=CARTESIAN_POINT ( 'NONE',  ( 34.87500000054622973, 22.36655054427230382, 83.50966788445364841 ) ) ;
#10911=CARTESIAN_POINT ( 'NONE',  ( 24.37500000054622262, 12.34168156654572535, 90.79316153445363113 ) ) ;
#10912=CARTESIAN_POINT ( 'NONE',  ( 23.49999999999998934, 27.88596668178699645, 90.79316153445363113 ) ) ;
#10914=CARTESIAN_POINT ( 'NONE',  ( 29.37500000054622973, 26.92701409722686634, 93.04388485072563242 ) ) ;
#10916=CARTESIAN_POINT ( 'NONE',  ( 22.75000000109246656, 22.43689772174679575, 83.29316153445363113 ) ) ;
#10917=ORIENTED_EDGE ( 'NONE', *, *, #7705, .F. ) ;
#10918=ORIENTED_EDGE ( 'NONE', *, *, #8153, .T. ) ;
#10923=AXIS2_PLACEMENT_3D ( 'NONE', #12059, #10325, #11160 ) ;
#10924=DIRECTION ( 'NONE',  ( -1.000000000000000000, 0.000000000000000000, -0.000000000000000000 ) ) ;
#10925=CARTESIAN_POINT ( 'NONE',  ( 39.47500000054622404, 26.92701409722686634, 93.04388485072563242 ) ) ;
#10927=EDGE_CURVE ( 'NONE', #10300, #9486, #2573, .T. ) ;
#10928=CARTESIAN_POINT ( 'NONE',  ( 38.57500000054622546, 13.80429023900056684, 86.29171490190961435 ) ) ;
#10929=CARTESIAN_POINT ( 'NONE',  ( 42.09999999999997300, 17.56310227825320425, 98.29316153445363113 ) ) ;
#10930=CARTESIAN_POINT ( 'NONE',  ( 48.17500000054623399, 13.07298590277314254, 93.04388485072563242 ) ) ;
#10932=ORIENTED_EDGE ( 'NONE', *, *, #4994, .T. ) ;
#10933=CARTESIAN_POINT ( 'NONE',  ( 23.75000000109246301, 17.56310227825320425, 98.29316153445363113 ) ) ;
#10937=CARTESIAN_POINT ( 'NONE',  ( 23.09999999999998721, 22.43689772174679575, 83.29316153445363113 ) ) ;
#10939=DIRECTION ( 'NONE',  ( 1.000000000000000000, -0.000000000000000000, -0.000000000000000000 ) ) ;
#10941=CARTESIAN_POINT ( 'NONE',  ( 48.99999999999998579, 20.00000000000000355, 83.29316153445364534 ) ) ;
#10943=CARTESIAN_POINT ( 'NONE',  ( 28.87500000054622262, 22.36655054427230382, 83.50966788445364841 ) ) ;
#10944=CARTESIAN_POINT ( 'NONE',  ( 31.57500000054622191, 26.19570976099943493, 95.29460816699764791 ) ) ;
#10949=ORIENTED_EDGE ( 'NONE', *, *, #12401, .F. ) ;
#10950=EDGE_CURVE ( 'NONE', #7418, #4704, #1268, .T. ) ;
#10951=FACE_OUTER_BOUND ( 'NONE', #5618, .T. ) ;
#10954=PLANE ( 'NONE',  #3764 ) ;
#10955=AXIS2_PLACEMENT_3D ( 'NONE', #10672, #92, #2878 ) ;
#10961=CARTESIAN_POINT ( 'NONE',  ( -34.99999999999999289, 20.00000000000000355, 170.0000119999999697 ) ) ;
#10964=CARTESIAN_POINT ( 'NONE',  ( 7.421492300118300633, 26.70405649111976842, 87.42232753731605044 ) ) ;
#10969=CARTESIAN_POINT ( 'NONE',  ( 42.17500000054622689, 13.07298590277314254, 93.04388485072563242 ) ) ;
#10971=ORIENTED_EDGE ( 'NONE', *, *, #391, .F. ) ;
#10974=CARTESIAN_POINT ( 'NONE',  ( 20.07500000054622546, 15.71886984736413417, 96.68563167572563088 ) ) ;
#10975=CARTESIAN_POINT ( 'NONE',  ( 46.47500000054622404, 13.07298590277314432, 88.54243821818161564 ) ) ;
#10976=CARTESIAN_POINT ( 'NONE',  ( 34.17500000054622689, 13.07298590277314254, 93.04388485072563242 ) ) ;
#10977=CARTESIAN_POINT ( 'NONE',  ( 23.67500000054622333, 24.28113015263587116, 96.68563167572563088 ) ) ;
#10980=CARTESIAN_POINT ( 'NONE',  ( 24.07500000054622902, 13.80429023900056507, 95.29460816699764791 ) ) ;
#10981=ORIENTED_EDGE ( 'NONE', *, *, #482, .F. ) ;
#10983=VERTEX_POINT ( 'NONE', #5749 ) ;
#10988=CARTESIAN_POINT ( 'NONE',  ( 37.77500000054622120, 22.36655054427230027, 98.07665518445361386 ) ) ;
#10991=CARTESIAN_POINT ( 'NONE',  ( 37.89999999999999147, 22.43689772174679575, 98.29316153445363113 ) ) ;
#10993=CARTESIAN_POINT ( 'NONE',  ( 47.97500000054622404, 15.71886984736413417, 96.68563167572563088 ) ) ;
#10994=ORIENTED_EDGE ( 'NONE', *, *, #12401, .T. ) ;
#10995=CARTESIAN_POINT ( 'NONE',  ( 25.65000000109246514, 20.00000000000000355, 98.29316153445363113 ) ) ;
#10997=ORIENTED_EDGE ( 'NONE', *, *, #4951, .T. ) ;
#11000=CARTESIAN_POINT ( 'NONE',  ( 24.95000000109246585, 26.37988106264029398, 86.15790661882942914 ) ) ;
#11002=CARTESIAN_POINT ( 'NONE',  ( 25.09999999999998366, 22.43689772174679575, 83.29316153445363113 ) ) ;
#11003=CARTESIAN_POINT ( 'NONE',  ( 31.37500000054622973, 26.92701409722686634, 93.04388485072563242 ) ) ;
#11004=CARTESIAN_POINT ( 'NONE',  ( 31.87500000054622262, 20.00000000000000355, 98.07665518445361386 ) ) ;
#11005=VECTOR ( 'NONE', #12057, 1000.000000000000000 ) ;
#11007=CARTESIAN_POINT ( 'NONE',  ( 49.99999999999998579, 0.000000000000000000, 82.99999999999995737 ) ) ;
#11008=ORIENTED_EDGE ( 'NONE', *, *, #9208, .T. ) ;
#11009=CARTESIAN_POINT ( 'NONE',  ( 46.05000000109246372, 12.86707612778636012, 93.11078899226572503 ) ) ;
#11011=EDGE_LOOP ( 'NONE', ( #2900, #6037, #11872, #11103, #8394, #9243, #4215, #6381, #1374, #4753, #6645, #1282, #10718 ) ) ;
#11012=CARTESIAN_POINT ( 'NONE',  ( -50.00000000000001421, 22.00000000000000000, 188.4007504869563263 ) ) ;
#11016=AXIS2_PLACEMENT_3D ( 'NONE', #7718, #10621, #7464 ) ;
#11021=CARTESIAN_POINT ( 'NONE',  ( 38.35000000109246798, 13.62011893735970958, 86.15790661882942914 ) ) ;
#11024=FACE_OUTER_BOUND ( 'NONE', #7367, .T. ) ;
#11026=VECTOR ( 'NONE', #2499, 1000.000000000000000 ) ;
#11033=CARTESIAN_POINT ( 'NONE',  ( 28.69999999999998508, 13.62011893735970958, 86.15790661882942914 ) ) ;
#11034=CARTESIAN_POINT ( 'NONE',  ( 44.97500000054621694, 22.36655054427230382, 83.50966788445364841 ) ) ;
#11035=CARTESIAN_POINT ( 'NONE',  ( 27.67500000054622689, 22.36655054427230027, 98.07665518445361386 ) ) ;
#11036=( BOUNDED_CURVE ( )  B_SPLINE_CURVE ( 2, ( #2793, #4696, #827, #1837, #12499, #12379, #9466, #2920, #8569, #6655, #12440 ),
 .UNSPECIFIED., .F., .F. ) 
 B_SPLINE_CURVE_WITH_KNOTS ( ( 3, 2, 2, 2, 2, 3 ),
 ( 0.6333333333333333037, 0.6400000000000000133, 0.6466666666666666119, 0.6533333333333333215, 0.6600000000000000311, 0.6666666666666666297 ),
 .UNSPECIFIED. ) 
 CURVE ( )  GEOMETRIC_REPRESENTATION_ITEM ( )  RATIONAL_B_SPLINE_CURVE ( ( 1.000000000000000000, 0.9510565162951535312, 1.000000000000000000, 0.9510565162951535312, 1.000000000000000000, 0.9510565162951535312, 1.000000000000000000, 0.9510565162951535312, 1.000000000000000000, 0.9510565162951535312, 1.000000000000000000 ) ) 
 REPRESENTATION_ITEM ( '' )  );
#11037=CARTESIAN_POINT ( 'NONE',  ( 10.00000000000000178, 19.47976500067654726, 83.29316153445364534 ) ) ;
#11039=CARTESIAN_POINT ( 'NONE',  ( -36.00000000000000711, 72.60660171779821326, 154.3533255156881694 ) ) ;
#11040=CARTESIAN_POINT ( 'NONE',  ( 23.57500000054622902, 24.28113015263587116, 96.68563167572563088 ) ) ;
#11042=ORIENTED_EDGE ( 'NONE', *, *, #4832, .T. ) ;
#11043=CARTESIAN_POINT ( 'NONE',  ( 32.65000000109246514, 20.00000000000000355, 83.29316153445364534 ) ) ;
#11044=ORIENTED_EDGE ( 'NONE', *, *, #3804, .F. ) ;
#11045=DIRECTION ( 'NONE',  ( 0.000000000000000000, 0.000000000000000000, -1.000000000000000000 ) ) ;
#11046=AXIS2_PLACEMENT_3D ( 'NONE', #5858, #1974, #2871 ) ;
#11048=CIRCLE ( 'NONE', #5579, 7.500000000000000000 ) ;
#11050=CARTESIAN_POINT ( 'NONE',  ( 33.07500000054622546, 24.28113015263587471, 84.90069139318163138 ) ) ;
#11051=LINE ( 'NONE', #5282, #10378 ) ;
#11052=CARTESIAN_POINT ( 'NONE',  ( 20.35000000109246088, 13.62011893735970958, 86.15790661882942914 ) ) ;
#11053=CARTESIAN_POINT ( 'NONE',  ( 31.77500000054622475, 22.36655054427230027, 98.07665518445361386 ) ) ;
#11054=EDGE_CURVE ( 'NONE', #7325, #1799, #799, .T. ) ;
#11055=CARTESIAN_POINT ( 'NONE',  ( 37.99999999999999289, 20.00000000000000355, 98.29316153445363113 ) ) ;
#11056=CARTESIAN_POINT ( 'NONE',  ( 46.47500000054623115, 13.80429023900056684, 86.29171490190961435 ) ) ;
#11057=ORIENTED_EDGE ( 'NONE', *, *, #12180, .F. ) ;
#11058=CARTESIAN_POINT ( 'NONE',  ( 27.35000000109246798, 26.37988106264029398, 95.42841645007781892 ) ) ;
#11063=ORIENTED_EDGE ( 'NONE', *, *, #4489, .F. ) ;
#11067=CARTESIAN_POINT ( 'NONE',  ( -2.000000000000015543, 20.00000000000000355, 98.29316153445363113 ) ) ;
#11068=CARTESIAN_POINT ( 'NONE',  ( 31.67500000054622689, 22.36655054427230027, 98.07665518445361386 ) ) ;
#11069=CARTESIAN_POINT ( 'NONE',  ( 24.27500000054622475, 13.07298590277314254, 93.04388485072563242 ) ) ;
#11070=DIRECTION ( 'NONE',  ( 0.000000000000000000, 0.000000000000000000, -1.000000000000000000 ) ) ;
#11073=CARTESIAN_POINT ( 'NONE',  ( 46.45000000109246230, 15.59161060780646046, 84.72553407664153724 ) ) ;
#11076=ORIENTED_EDGE ( 'NONE', *, *, #1568, .F. ) ;
#11084=CARTESIAN_POINT ( 'NONE',  ( 0.000000000000000000, 22.00000000000000000, 169.9999999999999716 ) ) ;
#11086=CYLINDRICAL_SURFACE ( 'NONE', #876, 7.500000000000007105 ) ;
#11094=CARTESIAN_POINT ( 'NONE',  ( 45.97500000054623115, 17.63344945572769973, 98.07665518445361386 ) ) ;
#11095=CARTESIAN_POINT ( 'NONE',  ( 24.47500000054623115, 13.80429023900056684, 86.29171490190961435 ) ) ;
#11096=CARTESIAN_POINT ( 'NONE',  ( 6.843016236096653770, 12.70761845378527610, 92.56370047283017755 ) ) ;
#11097=CARTESIAN_POINT ( 'NONE',  ( 45.55000000109246372, 22.43689772174676023, 98.29316153445364534 ) ) ;
#11098=DIRECTION ( 'NONE',  ( 0.000000000000000000, 0.000000000000000000, -1.000000000000000000 ) ) ;
#11099=CARTESIAN_POINT ( 'NONE',  ( -2.000000000000015543, 20.00000000000000355, 90.79316153445363113 ) ) ;
#11102=CARTESIAN_POINT ( 'NONE',  ( 34.99999999999998579, 20.00000000000000000, 137.5000000000000000 ) ) ;
#11103=ORIENTED_EDGE ( 'NONE', *, *, #1089, .F. ) ;
#11104=CARTESIAN_POINT ( 'NONE',  ( 0.000000000000000000, 20.00000000000000355, 69.99999999999998579 ) ) ;
#11105=ORIENTED_EDGE ( 'NONE', *, *, #4562, .T. ) ;
#11107=( BOUNDED_SURFACE ( )  B_SPLINE_SURFACE ( 1, 2, ( 
 ( #1213, #2020, #6846, #3928, #10709, #1025, #4885, #10771, #4115, #8747, #7803, #11675, #5902, #9771, #5079, #7866, #2084, #7740, #2852, #6715, #10582, #9648, #956, #2915, #8059, #2223, #8245, #5204, #5328, #1271, #5142, #10027, #2344, #1336, #10975, #3233, #4247, #2283, #6152, #11094, #4305, #8182, #10908, #9074, #11988, #7994, #12054, #443, #11863, #11034, #6092, #382, #12114, #2460, #9964, #3416, #9198, #8119, #9010, #7285, #6276, #6212, #6336, #321, #3293, #7156, #10086, #10203, #508, #1398, #5265, #9137, #3170, #3354, #7222, #4183, #1515, #5392, #11926, #4370, #7094, #7034, #2400, #10148, #1460, #11155, #9263, #564, #5872, #11645, #8489, #1753, #1991, #7774, #7344, #10382, #1578, #6517, #5517, #1695, #3538, #12175, #9510, #10261, #2952, #5456, #1637, #8307, #11214, #12361, #10320, #3661, #4427, #687, #9447, #3897, #6817, #9325, #2526, #10680, #12298, #7537, #6579, #11280, #4615, #7411, #9744, #5576, #2587, #4492, #9385, #749, #4554, #11404, #3478, #4857, #2714, #6397, #627, #8366, #8428, #991, #6459, #3598, #12235, #7474, #11348, #10443, #2654, #8722, #5637, #35, #10743, #4023, #3962, #5177, #8093, #3205, #5934, #6126, #230, #2257, #10805, #7009, #3268, #6061, #7838, #7130, #11768, #9994, #11707, #11959, #1307, #2121, #4087, #5998, #8782, #5113, #9871, #2054, #11004, #2316, #1118, #10944, #8845, #1058, #10879, #102, #7962, #3011, #1184, #9807, #6185, #4920, #8977, #9046, #6879, #4221, #4984, #2190, #165, #3138, #5050, #9934, #7898, #3074, #357, #6937, #8911, #11830, #1242, #291, #4154, #8029, #11900, #7067, #10060, #6313, #2497, #9360, #4525, #2376, #8155, #3570, #5363, #601, #12208, #4343, #10239, #477, #12272, #11191, #8217, #10123, #7255, #6372, #11129, #1552, #11316, #10293, #5425, #1371, #9109, #660, #10179, #6431, #12086, #9170, #1434, #1487, #538, #3455, #7192, #1611, #6245, #2435, #11069, #3388, #416, #5491, #8401, #3509, #5301, #2557, #9234, #11250, #4401, #7319, #7446, #9296, #4277, #2623, #8278, #5237, #12021, #12147, #4463, #3325, #8342, #7380, #10354, #9546, #4589, #12393, #10598, #977, #9420, #1912, #3821, #11439, #8462, #5797, #4780, #4712, #4842, #12331, #10480, #6609, #844, #10543, #7697 ),
 ( #1669, #11564, #3631, #8709, #7508, #3692, #5551, #722, #1853, #7571, #5735, #6491, #2749, #11501, #9667, #21, #11380, #2685, #3883, #1789, #9601, #8645, #782, #6673, #9482, #7757, #7635, #4651, #6550, #5675, #2809, #8583, #911, #11629, #6734, #12517, #10417, #1731, #5610, #12454, #2873, #8521, #3756, #6865, #11753, #5981, #8897, #84, #3190, #7824, #4007, #3947, #5921, #5860, #7051, #9981, #5098, #11690, #8012, #2104, #4139, #150, #215, #5163, #7950, #9729, #9030, #1102, #11885, #1046, #4968, #6924, #2934, #6991, #11815, #6800, #9855, #4907, #8831, #10929, #1290, #8766, #2243, #276, #7884, #2998, #6110, #1228, #1170, #342, #10728, #10790, #3062, #5033, #4205, #8079, #4072, #3122, #10862, #10666, #2172, #6045, #2041, #1976, #9791, #9919, #8963, #7177, #11946, #9217, #7117, #2419, #6170, #9156, #8141, #645, #6414, #1473, #462, #5346, #11055, #10991, #4449, #5223, #10277, #9094, #4324, #3251, #2301, #3439, #5285, #11176, #10046, #8201, #4384, #11232, #1595, #4264, #1357, #5476, #7241, #2479, #1535, #6232, #12131, #2362, #9342, #523, #10105, #12007, #12071, #8261, #3372, #7301, #4508, #12192, #6354, #401, #3309, #2542, #11114, #8326, #1418, #6296, #10167, #10222, #5408, #9279, #583, #3493, #7364, #9465, #5536, #11362, #11299, #12498, #2855, #10522, #704, #891, #7555, #9585, #5594, #1770, #10586, #825, #2605, #1897, #6533, #4761, #6475, #10401, #12377, #8384, #12439, #4695, #12252, #11425, #10337, #1712, #3803, #6718, #1655, #7682, #5718, #763, #9401, #11546, #6654, #6591, #5779, #4572, #3677, #8504, #2733, #9652, #8628, #4634, #10460, #5654, #3555, #3737, #9527, #8444, #960, #7429, #12314, #3613, #7491, #2670, #8568, #7618, #11481, #2792, #1835, #1028, #6095, #11867, #8880, #2157, #2227, #7997, #7743, #10774, #1962, #6908, #2024, #6850, #3867, #3931, #2088, #133, #8693, #6029, #11741, #9840, #11797, #3047, #3104, #6974, #5842, #4054, #198, #10713, #11611, #10912, #5964, #9903, #263, #3, #5905, #10649, #7806, #9713, #7934, #4889, #11678, #1153, #7870, #8814, #8750, #3174, #10843, #8950, #9775, #66, #4119, #9967, #1216, #5015, #5082, #7037, #3992, #1085, #4828, #2984, #4950, #2919, #6782, #8122, #11992 ) ),
 .UNSPECIFIED., .F., .F., .F. ) 
 B_SPLINE_SURFACE_WITH_KNOTS ( ( 2, 2 ),
 ( 3, 2, 2, 2, 2, 2, 2, 2, 2, 2, 2, 2, 2, 2, 2, 2, 2, 2, 2, 2, 2, 2, 2, 2, 2, 2, 2, 2, 2, 2, 2, 2, 2, 2, 2, 2, 2, 2, 2, 2, 2, 2, 2, 2, 2, 2, 2, 2, 2, 2, 2, 2, 2, 2, 2, 2, 2, 2, 2, 2, 2, 2, 2, 2, 2, 2, 2, 2, 2, 2, 2, 2, 2, 2, 2, 2, 2, 2, 2, 2, 2, 2, 2, 2, 2, 2, 2, 2, 2, 2, 2, 2, 2, 2, 2, 2, 2, 2, 2, 2, 2, 2, 2, 2, 2, 2, 2, 2, 2, 2, 2, 2, 2, 2, 2, 2, 2, 2, 2, 2, 2, 2, 2, 2, 2, 2, 2, 2, 2, 2, 2, 2, 2, 2, 2, 2, 2, 2, 2, 2, 2, 2, 2, 2, 2, 2, 2, 2, 2, 2, 3 ),
 ( 0.000000000000000000, 1.000000000000000000 ),
 ( 0.000000000000000000, 0.006666666666666667095, 0.01333333333333333419, 0.02000000000000000042, 0.02666666666666666838, 0.03333333333333333287, 0.04000000000000000083, 0.04666666666666666879, 0.05333333333333333676, 0.05999999999999999778, 0.06666666666666666574, 0.07333333333333333370, 0.08000000000000000167, 0.08666666666666666963, 0.09333333333333333759, 0.1000000000000000056, 0.1066666666666666735, 0.1133333333333333276, 0.1199999999999999956, 0.1266666666666666774, 0.1333333333333333315, 0.1400000000000000133, 0.1466666666666666674, 0.1533333333333333215, 0.1600000000000000033, 0.1666666666666666574, 0.1733333333333333393, 0.1799999999999999933, 0.1866666666666666752, 0.1933333333333333293, 0.2000000000000000111, 0.2066666666666666652, 0.2133333333333333470, 0.2200000000000000011, 0.2266666666666666552, 0.2333333333333333370, 0.2399999999999999911, 0.2466666666666666730, 0.2533333333333333548, 0.2600000000000000089, 0.2666666666666666630, 0.2733333333333333171, 0.2800000000000000266, 0.2866666666666666807, 0.2933333333333333348, 0.2999999999999999889, 0.3066666666666666430, 0.3133333333333333526, 0.3200000000000000067, 0.3266666666666666607, 0.3333333333333333148, 0.3400000000000000244, 0.3466666666666666785, 0.3533333333333333326, 0.3599999999999999867, 0.3666666666666666408, 0.3733333333333333504, 0.3800000000000000044, 0.3866666666666666585, 0.3933333333333333126, 0.4000000000000000222, 0.4066666666666666763, 0.4133333333333333304, 0.4199999999999999845, 0.4266666666666666941, 0.4333333333333333481, 0.4400000000000000022, 0.4466666666666666563, 0.4533333333333333104, 0.4600000000000000200, 0.4666666666666666741, 0.4733333333333333282, 0.4799999999999999822, 0.4866666666666666918, 0.4933333333333333459, 0.5000000000000000000, 0.5066666666666667096, 0.5133333333333333082, 0.5200000000000000178, 0.5266666666666666163, 0.5333333333333333259, 0.5400000000000000355, 0.5466666666666666341, 0.5533333333333333437, 0.5600000000000000533, 0.5666666666666666519, 0.5733333333333333615, 0.5799999999999999600, 0.5866666666666666696, 0.5933333333333333792, 0.5999999999999999778, 0.6066666666666666874, 0.6133333333333332860, 0.6199999999999999956, 0.6266666666666667052, 0.6333333333333333037, 0.6400000000000000133, 0.6466666666666666119, 0.6533333333333333215, 0.6600000000000000311, 0.6666666666666666297, 0.6733333333333333393, 0.6800000000000000488, 0.6866666666666666474, 0.6933333333333333570, 0.6999999999999999556, 0.7066666666666666652, 0.7133333333333333748, 0.7199999999999999734, 0.7266666666666666829, 0.7333333333333332815, 0.7399999999999999911, 0.7466666666666667007, 0.7533333333333332993, 0.7600000000000000089, 0.7666666666666667185, 0.7733333333333333171, 0.7800000000000000266, 0.7866666666666666252, 0.7933333333333333348, 0.8000000000000000444, 0.8066666666666666430, 0.8133333333333333526, 0.8199999999999999512, 0.8266666666666666607, 0.8333333333333333703, 0.8399999999999999689, 0.8466666666666666785, 0.8533333333333333881, 0.8599999999999999867, 0.8666666666666666963, 0.8733333333333332948, 0.8800000000000000044, 0.8866666666666667140, 0.8933333333333333126, 0.9000000000000000222, 0.9066666666666666208, 0.9133333333333333304, 0.9200000000000000400, 0.9266666666666666385, 0.9333333333333333481, 0.9399999999999999467, 0.9466666666666666563, 0.9533333333333333659, 0.9599999999999999645, 0.9666666666666666741, 0.9733333333333333837, 0.9799999999999999822, 0.9866666666666666918, 0.9933333333333332904, 1.000000000000000000 ),
 .UNSPECIFIED. ) 
 GEOMETRIC_REPRESENTATION_ITEM ( )  RATIONAL_B_SPLINE_SURFACE ( (
 ( 1.000000000000000000, 0.9510565162951535312, 1.000000000000000000, 0.9510565162951535312, 1.000000000000000000, 0.9510565162951535312, 1.000000000000000000, 0.9510565162951535312, 1.000000000000000000, 0.9510565162951535312, 1.000000000000000000, 0.9510565162951535312, 1.000000000000000000, 0.9510565162951535312, 1.000000000000000000, 0.9510565162951535312, 1.000000000000000000, 0.9510565162951535312, 1.000000000000000000, 0.9510565162951535312, 1.000000000000000000, 0.9510565162951535312, 1.000000000000000000, 0.9510565162951535312, 1.000000000000000000, 0.9510565162951535312, 1.000000000000000000, 0.9510565162951535312, 1.000000000000000000, 0.9510565162951535312, 1.000000000000000000, 0.9510565162951535312, 1.000000000000000000, 0.9510565162951535312, 1.000000000000000000, 0.9510565162951535312, 1.000000000000000000, 0.9510565162951535312, 1.000000000000000000, 0.9510565162951535312, 1.000000000000000000, 0.9510565162951535312, 1.000000000000000000, 0.9510565162951535312, 1.000000000000000000, 0.9510565162951535312, 1.000000000000000000, 0.9510565162951535312, 1.000000000000000000, 0.9510565162951535312, 1.000000000000000000, 0.9510565162951535312, 1.000000000000000000, 0.9510565162951535312, 1.000000000000000000, 0.9510565162951535312, 1.000000000000000000, 0.9510565162951535312, 1.000000000000000000, 0.9510565162951535312, 1.000000000000000000, 0.9510565162951535312, 1.000000000000000000, 0.9510565162951535312, 1.000000000000000000, 0.9510565162951535312, 1.000000000000000000, 0.9510565162951535312, 1.000000000000000000, 0.9510565162951535312, 1.000000000000000000, 0.9510565162951535312, 1.000000000000000000, 0.9510565162951535312, 1.000000000000000000, 0.9510565162951535312, 1.000000000000000000, 0.9510565162951535312, 1.000000000000000000, 0.9510565162951535312, 1.000000000000000000, 0.9510565162951535312, 1.000000000000000000, 0.9510565162951535312, 1.000000000000000000, 0.9510565162951535312, 1.000000000000000000, 0.9510565162951535312, 1.000000000000000000, 0.9510565162951535312, 1.000000000000000000, 0.9510565162951535312, 1.000000000000000000, 0.9510565162951535312, 1.000000000000000000, 0.9510565162951535312, 1.000000000000000000, 0.9510565162951535312, 1.000000000000000000, 0.9510565162951535312, 1.000000000000000000, 0.9510565162951535312, 1.000000000000000000, 0.9510565162951535312, 1.000000000000000000, 0.9510565162951535312, 1.000000000000000000, 0.9510565162951535312, 1.000000000000000000, 0.9510565162951535312, 1.000000000000000000, 0.9510565162951535312, 1.000000000000000000, 0.9510565162951535312, 1.000000000000000000, 0.9510565162951535312, 1.000000000000000000, 0.9510565162951535312, 1.000000000000000000, 0.9510565162951535312, 1.000000000000000000, 0.9510565162951535312, 1.000000000000000000, 0.9510565162951535312, 1.000000000000000000, 0.9510565162951535312, 1.000000000000000000, 0.9510565162951535312, 1.000000000000000000, 0.9510565162951535312, 1.000000000000000000, 0.9510565162951535312, 1.000000000000000000, 0.9510565162951535312, 1.000000000000000000, 0.9510565162951535312, 1.000000000000000000, 0.9510565162951535312, 1.000000000000000000, 0.9510565162951535312, 1.000000000000000000, 0.9510565162951535312, 1.000000000000000000, 0.9510565162951535312, 1.000000000000000000, 0.9510565162951535312, 1.000000000000000000, 0.9510565162951535312, 1.000000000000000000, 0.9510565162951535312, 1.000000000000000000, 0.9510565162951535312, 1.000000000000000000, 0.9510565162951535312, 1.000000000000000000, 0.9510565162951535312, 1.000000000000000000, 0.9510565162951535312, 1.000000000000000000, 0.9510565162951535312, 1.000000000000000000, 0.9510565162951535312, 1.000000000000000000, 0.9510565162951535312, 1.000000000000000000, 0.9510565162951535312, 1.000000000000000000, 0.9510565162951535312, 1.000000000000000000, 0.9510565162951535312, 1.000000000000000000, 0.9510565162951535312, 1.000000000000000000, 0.9510565162951535312, 1.000000000000000000, 0.9510565162951535312, 1.000000000000000000, 0.9510565162951535312, 1.000000000000000000, 0.9510565162951535312, 1.000000000000000000, 0.9510565162951535312, 1.000000000000000000, 0.9510565162951535312, 1.000000000000000000, 0.9510565162951535312, 1.000000000000000000, 0.9510565162951535312, 1.000000000000000000, 0.9510565162951535312, 1.000000000000000000, 0.9510565162951535312, 1.000000000000000000, 0.9510565162951535312, 1.000000000000000000, 0.9510565162951535312, 1.000000000000000000, 0.9510565162951535312, 1.000000000000000000, 0.9510565162951535312, 1.000000000000000000, 0.9510565162951535312, 1.000000000000000000, 0.9510565162951535312, 1.000000000000000000, 0.9510565162951535312, 1.000000000000000000, 0.9510565162951535312, 1.000000000000000000, 0.9510565162951535312, 1.000000000000000000, 0.9510565162951535312, 1.000000000000000000, 0.9510565162951535312, 1.000000000000000000, 0.9510565162951535312, 1.000000000000000000, 0.9510565162951535312, 1.000000000000000000, 0.9510565162951535312, 1.000000000000000000, 0.9510565162951535312, 1.000000000000000000, 0.9510565162951535312, 1.000000000000000000, 0.9510565162951535312, 1.000000000000000000, 0.9510565162951535312, 1.000000000000000000, 0.9510565162951535312, 1.000000000000000000, 0.9510565162951535312, 1.000000000000000000, 0.9510565162951535312, 1.000000000000000000, 0.9510565162951535312, 1.000000000000000000, 0.9510565162951535312, 1.000000000000000000, 0.9510565162951535312, 1.000000000000000000, 0.9510565162951535312, 1.000000000000000000, 0.9510565162951535312, 1.000000000000000000, 0.9510565162951535312, 1.000000000000000000, 0.9510565162951535312, 1.000000000000000000, 0.9510565162951535312, 1.000000000000000000, 0.9510565162951535312, 1.000000000000000000, 0.9510565162951535312, 1.000000000000000000, 0.9510565162951535312, 1.000000000000000000, 0.9510565162951535312, 1.000000000000000000, 0.9510565162951535312, 1.000000000000000000, 0.9510565162951535312, 1.000000000000000000, 0.9510565162951535312, 1.000000000000000000, 0.9510565162951535312, 1.000000000000000000, 0.9510565162951535312, 1.000000000000000000, 0.9510565162951535312, 1.000000000000000000, 0.9510565162951535312, 1.000000000000000000, 0.9510565162951535312, 1.000000000000000000, 0.9510565162951535312, 1.000000000000000000, 0.9510565162951535312, 1.000000000000000000, 0.9510565162951535312, 1.000000000000000000, 0.9510565162951535312, 1.000000000000000000, 0.9510565162951535312, 1.000000000000000000, 0.9510565162951535312, 1.000000000000000000, 0.9510565162951535312, 1.000000000000000000, 0.9510565162951535312, 1.000000000000000000, 0.9510565162951535312, 1.000000000000000000, 0.9510565162951535312, 1.000000000000000000, 0.9510565162951535312, 1.000000000000000000, 0.9510565162951535312, 1.000000000000000000, 0.9510565162951535312, 1.000000000000000000),
 ( 1.000000000000000000, 0.9510565162951535312, 1.000000000000000000, 0.9510565162951535312, 1.000000000000000000, 0.9510565162951535312, 1.000000000000000000, 0.9510565162951535312, 1.000000000000000000, 0.9510565162951535312, 1.000000000000000000, 0.9510565162951535312, 1.000000000000000000, 0.9510565162951535312, 1.000000000000000000, 0.9510565162951535312, 1.000000000000000000, 0.9510565162951535312, 1.000000000000000000, 0.9510565162951535312, 1.000000000000000000, 0.9510565162951535312, 1.000000000000000000, 0.9510565162951535312, 1.000000000000000000, 0.9510565162951535312, 1.000000000000000000, 0.9510565162951535312, 1.000000000000000000, 0.9510565162951535312, 1.000000000000000000, 0.9510565162951535312, 1.000000000000000000, 0.9510565162951535312, 1.000000000000000000, 0.9510565162951535312, 1.000000000000000000, 0.9510565162951535312, 1.000000000000000000, 0.9510565162951535312, 1.000000000000000000, 0.9510565162951535312, 1.000000000000000000, 0.9510565162951535312, 1.000000000000000000, 0.9510565162951535312, 1.000000000000000000, 0.9510565162951535312, 1.000000000000000000, 0.9510565162951535312, 1.000000000000000000, 0.9510565162951535312, 1.000000000000000000, 0.9510565162951535312, 1.000000000000000000, 0.9510565162951535312, 1.000000000000000000, 0.9510565162951535312, 1.000000000000000000, 0.9510565162951535312, 1.000000000000000000, 0.9510565162951535312, 1.000000000000000000, 0.9510565162951535312, 1.000000000000000000, 0.9510565162951535312, 1.000000000000000000, 0.9510565162951535312, 1.000000000000000000, 0.9510565162951535312, 1.000000000000000000, 0.9510565162951535312, 1.000000000000000000, 0.9510565162951535312, 1.000000000000000000, 0.9510565162951535312, 1.000000000000000000, 0.9510565162951535312, 1.000000000000000000, 0.9510565162951535312, 1.000000000000000000, 0.9510565162951535312, 1.000000000000000000, 0.9510565162951535312, 1.000000000000000000, 0.9510565162951535312, 1.000000000000000000, 0.9510565162951535312, 1.000000000000000000, 0.9510565162951535312, 1.000000000000000000, 0.9510565162951535312, 1.000000000000000000, 0.9510565162951535312, 1.000000000000000000, 0.9510565162951535312, 1.000000000000000000, 0.9510565162951535312, 1.000000000000000000, 0.9510565162951535312, 1.000000000000000000, 0.9510565162951535312, 1.000000000000000000, 0.9510565162951535312, 1.000000000000000000, 0.9510565162951535312, 1.000000000000000000, 0.9510565162951535312, 1.000000000000000000, 0.9510565162951535312, 1.000000000000000000, 0.9510565162951535312, 1.000000000000000000, 0.9510565162951535312, 1.000000000000000000, 0.9510565162951535312, 1.000000000000000000, 0.9510565162951535312, 1.000000000000000000, 0.9510565162951535312, 1.000000000000000000, 0.9510565162951535312, 1.000000000000000000, 0.9510565162951535312, 1.000000000000000000, 0.9510565162951535312, 1.000000000000000000, 0.9510565162951535312, 1.000000000000000000, 0.9510565162951535312, 1.000000000000000000, 0.9510565162951535312, 1.000000000000000000, 0.9510565162951535312, 1.000000000000000000, 0.9510565162951535312, 1.000000000000000000, 0.9510565162951535312, 1.000000000000000000, 0.9510565162951535312, 1.000000000000000000, 0.9510565162951535312, 1.000000000000000000, 0.9510565162951535312, 1.000000000000000000, 0.9510565162951535312, 1.000000000000000000, 0.9510565162951535312, 1.000000000000000000, 0.9510565162951535312, 1.000000000000000000, 0.9510565162951535312, 1.000000000000000000, 0.9510565162951535312, 1.000000000000000000, 0.9510565162951535312, 1.000000000000000000, 0.9510565162951535312, 1.000000000000000000, 0.9510565162951535312, 1.000000000000000000, 0.9510565162951535312, 1.000000000000000000, 0.9510565162951535312, 1.000000000000000000, 0.9510565162951535312, 1.000000000000000000, 0.9510565162951535312, 1.000000000000000000, 0.9510565162951535312, 1.000000000000000000, 0.9510565162951535312, 1.000000000000000000, 0.9510565162951535312, 1.000000000000000000, 0.9510565162951535312, 1.000000000000000000, 0.9510565162951535312, 1.000000000000000000, 0.9510565162951535312, 1.000000000000000000, 0.9510565162951535312, 1.000000000000000000, 0.9510565162951535312, 1.000000000000000000, 0.9510565162951535312, 1.000000000000000000, 0.9510565162951535312, 1.000000000000000000, 0.9510565162951535312, 1.000000000000000000, 0.9510565162951535312, 1.000000000000000000, 0.9510565162951535312, 1.000000000000000000, 0.9510565162951535312, 1.000000000000000000, 0.9510565162951535312, 1.000000000000000000, 0.9510565162951535312, 1.000000000000000000, 0.9510565162951535312, 1.000000000000000000, 0.9510565162951535312, 1.000000000000000000, 0.9510565162951535312, 1.000000000000000000, 0.9510565162951535312, 1.000000000000000000, 0.9510565162951535312, 1.000000000000000000, 0.9510565162951535312, 1.000000000000000000, 0.9510565162951535312, 1.000000000000000000, 0.9510565162951535312, 1.000000000000000000, 0.9510565162951535312, 1.000000000000000000, 0.9510565162951535312, 1.000000000000000000, 0.9510565162951535312, 1.000000000000000000, 0.9510565162951535312, 1.000000000000000000, 0.9510565162951535312, 1.000000000000000000, 0.9510565162951535312, 1.000000000000000000, 0.9510565162951535312, 1.000000000000000000, 0.9510565162951535312, 1.000000000000000000, 0.9510565162951535312, 1.000000000000000000, 0.9510565162951535312, 1.000000000000000000, 0.9510565162951535312, 1.000000000000000000, 0.9510565162951535312, 1.000000000000000000, 0.9510565162951535312, 1.000000000000000000, 0.9510565162951535312, 1.000000000000000000, 0.9510565162951535312, 1.000000000000000000, 0.9510565162951535312, 1.000000000000000000, 0.9510565162951535312, 1.000000000000000000, 0.9510565162951535312, 1.000000000000000000, 0.9510565162951535312, 1.000000000000000000, 0.9510565162951535312, 1.000000000000000000, 0.9510565162951535312, 1.000000000000000000, 0.9510565162951535312, 1.000000000000000000, 0.9510565162951535312, 1.000000000000000000, 0.9510565162951535312, 1.000000000000000000, 0.9510565162951535312, 1.000000000000000000, 0.9510565162951535312, 1.000000000000000000, 0.9510565162951535312, 1.000000000000000000, 0.9510565162951535312, 1.000000000000000000, 0.9510565162951535312, 1.000000000000000000, 0.9510565162951535312, 1.000000000000000000, 0.9510565162951535312, 1.000000000000000000, 0.9510565162951535312, 1.000000000000000000, 0.9510565162951535312, 1.000000000000000000, 0.9510565162951535312, 1.000000000000000000, 0.9510565162951535312, 1.000000000000000000, 0.9510565162951535312, 1.000000000000000000, 0.9510565162951535312, 1.000000000000000000, 0.9510565162951535312, 1.000000000000000000, 0.9510565162951535312, 1.000000000000000000, 0.9510565162951535312, 1.000000000000000000, 0.9510565162951535312, 1.000000000000000000, 0.9510565162951535312, 1.000000000000000000) ) ) 
 REPRESENTATION_ITEM ( '' )  SURFACE ( )  );
#11109=VECTOR ( 'NONE', #7841, 1000.000000000000000 ) ;
#11110=CARTESIAN_POINT ( 'NONE',  ( 32.67500000054622689, 15.71886984736413773, 84.90069139318163138 ) ) ;
#11112=CARTESIAN_POINT ( 'NONE',  ( 47.47500000054623115, 26.19570976099943849, 95.29460816699764791 ) ) ;
#11113=CARTESIAN_POINT ( 'NONE',  ( 36.67500000054622689, 15.71886984736413773, 84.90069139318163138 ) ) ;
#11114=CARTESIAN_POINT ( 'NONE',  ( 33.99999999999998579, 20.00000000000000355, 98.29316153445363113 ) ) ;
#11115=CARTESIAN_POINT ( 'NONE',  ( 46.97500000054623115, 24.28113015263587471, 84.90069139318163138 ) ) ;
#11117=CARTESIAN_POINT ( 'NONE',  ( 22.85000000109246443, 24.40838939219355197, 84.72553407664153724 ) ) ;
#11122=EDGE_LOOP ( 'NONE', ( #1644, #9174, #4997, #10799 ) ) ;
#11123=CARTESIAN_POINT ( 'NONE',  ( 0.000000000000000000, 0.000000000000000000, 169.9999999999999716 ) ) ;
#11124=LINE ( 'NONE', #2430, #2625 ) ;
#11125=LINE ( 'NONE', #6369, #5435 ) ;
#11126=FACE_OUTER_BOUND ( 'NONE', #3890, .T. ) ;
#11127=VECTOR ( 'NONE', #10617, 1000.000000000000000 ) ;
#11128=CARTESIAN_POINT ( 'NONE',  ( 24.77500000054622831, 20.00000000000000355, 83.50966788445364841 ) ) ;
#11129=CARTESIAN_POINT ( 'NONE',  ( 26.27500000054622475, 13.07298590277314254, 93.04388485072563242 ) ) ;
#11134=CARTESIAN_POINT ( 'NONE',  ( 44.65000000109246514, 20.00000000000000355, 83.29316153445364534 ) ) ;
#11137=CARTESIAN_POINT ( 'NONE',  ( 29.65000000109246514, 20.00000000000000355, 98.29316153445363113 ) ) ;
#11148=DIRECTION ( 'NONE',  ( -0.000000000000000000, -0.000000000000000000, 1.000000000000000000 ) ) ;
#11151=( BOUNDED_CURVE ( )  B_SPLINE_CURVE ( 3, ( #116, #11594, #2068, #2903 ),
 .UNSPECIFIED., .F., .F. ) 
 B_SPLINE_CURVE_WITH_KNOTS ( ( 4, 4 ),
 ( 3.411525449423196132, 4.712388980384689674 ),
 .UNSPECIFIED. ) 
 CURVE ( )  GEOMETRIC_REPRESENTATION_ITEM ( )  RATIONAL_B_SPLINE_CURVE ( ( 1.000000000000000000, 0.8638816171694809753, 0.8638816171694809753, 1.000000000000000000 ) ) 
 REPRESENTATION_ITEM ( '' )  );
#11153=CARTESIAN_POINT ( 'NONE',  ( -2.000000000000015543, 20.00000000000000355, 90.79316153445363113 ) ) ;
#11154=DIRECTION ( 'NONE',  ( 0.4999999999999892308, 0.000000000000000000, -0.8660254037844448138 ) ) ;
#11155=CARTESIAN_POINT ( 'NONE',  ( 41.37500000054622973, 27.65831843345427998, 90.79316153445363113 ) ) ;
#11156=CARTESIAN_POINT ( 'NONE',  ( 28.07500000054622902, 13.80429023900056507, 95.29460816699764791 ) ) ;
#11158=CARTESIAN_POINT ( 'NONE',  ( -6.999999999999999112, 92.00000000000000000, 69.99999999999998579 ) ) ;
#11160=DIRECTION ( 'NONE',  ( 0.000000000000000000, 0.000000000000000000, -1.000000000000000000 ) ) ;
#11164=ORIENTED_EDGE ( 'NONE', *, *, #10691, .F. ) ;
#11165=CARTESIAN_POINT ( 'NONE',  ( 48.65000000109246514, 20.00000000000000355, 83.29316153445364534 ) ) ;
#11169=( BOUNDED_CURVE ( )  B_SPLINE_CURVE ( 2, ( #159, #7958, #4082, #7186, #1301, #1179, #410, #11000, #10801, #2310, #9040 ),
 .UNSPECIFIED., .F., .F. ) 
 B_SPLINE_CURVE_WITH_KNOTS ( ( 3, 2, 2, 2, 2, 3 ),
 ( 0.8000000000000000444, 0.8066666666666666430, 0.8133333333333333526, 0.8199999999999999512, 0.8266666666666666607, 0.8333333333333333703 ),
 .UNSPECIFIED. ) 
 CURVE ( )  GEOMETRIC_REPRESENTATION_ITEM ( )  RATIONAL_B_SPLINE_CURVE ( ( 1.000000000000000000, 0.9510565162951535312, 1.000000000000000000, 0.9510565162951535312, 1.000000000000000000, 0.9510565162951535312, 1.000000000000000000, 0.9510565162951535312, 1.000000000000000000, 0.9510565162951535312, 1.000000000000000000 ) ) 
 REPRESENTATION_ITEM ( '' )  );
#11171=CARTESIAN_POINT ( 'NONE',  ( 32.47500000054621694, 13.07298590277314432, 88.54243821818161564 ) ) ;
#11174=CARTESIAN_POINT ( 'NONE',  ( 44.87500000054623683, 22.36655054427230382, 83.50966788445364841 ) ) ;
#11175=CARTESIAN_POINT ( 'NONE',  ( 36.57500000054621125, 13.80429023900056684, 86.29171490190961435 ) ) ;
#11176=CARTESIAN_POINT ( 'NONE',  ( 36.89999999999997726, 17.56310227825321135, 83.29316153445363113 ) ) ;
#11178=CARTESIAN_POINT ( 'NONE',  ( 46.17500000054623399, 13.07298590277314254, 93.04388485072563242 ) ) ;
#11180=CARTESIAN_POINT ( 'NONE',  ( 27.25000000109246656, 27.13292387221364876, 93.11078899226573924 ) ) ;
#11186=DIRECTION ( 'NONE',  ( 0.000000000000000000, 0.000000000000000000, -1.000000000000000000 ) ) ;
#11190=CARTESIAN_POINT ( 'NONE',  ( 27.37500000054622973, 26.92701409722686634, 93.04388485072563242 ) ) ;
#11191=CARTESIAN_POINT ( 'NONE',  ( 26.77500000054622475, 17.63344945572770328, 83.50966788445364841 ) ) ;
#11192=LINE ( 'NONE', #8156, #11026 ) ;
#11196=VERTEX_POINT ( 'NONE', #5999 ) ;
#11197=CARTESIAN_POINT ( 'NONE',  ( 30.25000000109246656, 12.86707612778636012, 88.47553407664152303 ) ) ;
#11198=ORIENTED_EDGE ( 'NONE', *, *, #3891, .F. ) ;
#11201=CARTESIAN_POINT ( 'NONE',  ( 20.57500000054622902, 15.71886984736413773, 84.90069139318163138 ) ) ;
#11208=CARTESIAN_POINT ( 'NONE',  ( 47.05000000109247082, 27.13292387221364876, 88.47553407664153724 ) ) ;
#11209=VERTEX_POINT ( 'NONE', #8979 ) ;
#11212=EDGE_CURVE ( 'NONE', #5229, #2895, #9457, .T. ) ;
#11213=DIRECTION ( 'NONE',  ( 0.000000000000000000, -0.000000000000000000, 1.000000000000000000 ) ) ;
#11214=CARTESIAN_POINT ( 'NONE',  ( 39.07500000054622546, 24.28113015263587471, 84.90069139318163138 ) ) ;
#11216=CARTESIAN_POINT ( 'NONE',  ( 28.47500000054622760, 13.80429023900056684, 86.29171490190961435 ) ) ;
#11217=CARTESIAN_POINT ( 'NONE',  ( 7.146575930227264450, 13.00402921949032731, 93.50701428624745404 ) ) ;
#11218=DIRECTION ( 'NONE',  ( -0.000000000000000000, -1.000000000000000000, -0.000000000000000000 ) ) ;
#11219=AXIS2_PLACEMENT_3D ( 'NONE', #3124, #9858, #2175 ) ;
#11221=CARTESIAN_POINT ( 'NONE',  ( 34.99999999999999289, 20.00000000000000355, 83.29316153445364534 ) ) ;
#11222=ORIENTED_EDGE ( 'NONE', *, *, #12102, .T. ) ;
#11223=CARTESIAN_POINT ( 'NONE',  ( -50.00000000000001421, 18.00000000000000355, 152.2284161474004520 ) ) ;
#11224=ORIENTED_EDGE ( 'NONE', *, *, #10950, .T. ) ;
#11225=DIRECTION ( 'NONE',  ( -0.000000000000000000, -0.000000000000000000, 1.000000000000000000 ) ) ;
#11228=CARTESIAN_POINT ( 'NONE',  ( 30.47500000054622404, 13.07298590277314432, 88.54243821818161564 ) ) ;
#11230=CARTESIAN_POINT ( 'NONE',  ( 46.37500000054622973, 13.07298590277314432, 88.54243821818161564 ) ) ;
#11231=CARTESIAN_POINT ( 'NONE',  ( 35.37500000054622973, 27.65831843345427998, 90.79316153445363113 ) ) ;
#11232=CARTESIAN_POINT ( 'NONE',  ( 36.49999999999998579, 12.11403331821300533, 90.79316153445363113 ) ) ;
#11235=CARTESIAN_POINT ( 'NONE',  ( 37.97500000054623115, 15.71886984736413417, 96.68563167572563088 ) ) ;
#11238=CARTESIAN_POINT ( 'NONE',  ( 45.67500000054621978, 22.36655054427230027, 98.07665518445361386 ) ) ;
#11243=ORIENTED_EDGE ( 'NONE', *, *, #7190, .F. ) ;
#11245=CARTESIAN_POINT ( 'NONE',  ( 4.999999999999997335, 20.00000000000000000, 137.5000000000000000 ) ) ;
#11248=CARTESIAN_POINT ( 'NONE',  ( 32.55000000109247082, 17.56310227825320425, 83.29316153445363113 ) ) ;
#11249=CARTESIAN_POINT ( 'NONE',  ( 26.47500000054623115, 13.80429023900056684, 86.29171490190961435 ) ) ;
#11250=CARTESIAN_POINT ( 'NONE',  ( 23.37500000054621907, 27.65831843345427998, 90.79316153445363113 ) ) ;
#11251=DIRECTION ( 'NONE',  ( 1.000000000000000000, -0.000000000000000000, -0.000000000000000000 ) ) ;
#11253=ORIENTED_EDGE ( 'NONE', *, *, #4726, .F. ) ;
#11255=CARTESIAN_POINT ( 'NONE',  ( 36.85000000109246798, 24.40838939219355197, 84.72553407664153724 ) ) ;
#11261=ADVANCED_FACE ( 'NONE', ( #6246 ), #8094, .F. ) ;
#11262=VERTEX_POINT ( 'NONE', #9997 ) ;
#11263=CARTESIAN_POINT ( 'NONE',  ( 33.65000000109246514, 20.00000000000000355, 98.29316153445363113 ) ) ;
#11265=CARTESIAN_POINT ( 'NONE',  ( 19.77500000054622831, 20.00000000000000355, 98.07665518445361386 ) ) ;
#11268=CARTESIAN_POINT ( 'NONE',  ( 38.05000000109246372, 12.86707612778636012, 93.11078899226572503 ) ) ;
#11272=CARTESIAN_POINT ( 'NONE',  ( 26.47500000054623115, 13.80429023900056684, 86.29171490190961435 ) ) ;
#11277=DIRECTION ( 'NONE',  ( 1.000000000000000000, 0.000000000000000000, -0.000000000000000000 ) ) ;
#11278=FACE_OUTER_BOUND ( 'NONE', #12134, .T. ) ;
#11279=CARTESIAN_POINT ( 'NONE',  ( 38.17500000054622689, 13.07298590277314254, 93.04388485072563242 ) ) ;
#11280=CARTESIAN_POINT ( 'NONE',  ( 37.57500000054623257, 26.19570976099943493, 95.29460816699764791 ) ) ;
#11282=CARTESIAN_POINT ( 'NONE',  ( 28.67500000054623044, 17.63344945572770328, 83.50966788445364841 ) ) ;
#11287=CARTESIAN_POINT ( 'NONE',  ( 31.39999999999998437, 27.13292387221364876, 88.47553407664153724 ) ) ;
#11288=ORIENTED_EDGE ( 'NONE', *, *, #5683, .T. ) ;
#11291=ADVANCED_FACE ( 'NONE', ( #9236 ), #11961, .T. ) ;
#11295=CARTESIAN_POINT ( 'NONE',  ( 30.77500000054622120, 17.63344945572770328, 83.50966788445364841 ) ) ;
#11296=CARTESIAN_POINT ( 'NONE',  ( 27.05000000109246372, 27.13292387221364876, 88.47553407664153724 ) ) ;
#11297=CARTESIAN_POINT ( 'NONE',  ( 44.37500000054622973, 13.07298590277314432, 88.54243821818161564 ) ) ;
#11298=CARTESIAN_POINT ( 'NONE',  ( 34.97500000054622404, 22.36655054427230382, 83.50966788445364841 ) ) ;
#11299=CARTESIAN_POINT ( 'NONE',  ( 32.59999999999998721, 12.86707612778636012, 88.47553407664152303 ) ) ;
#11302=CARTESIAN_POINT ( 'NONE',  ( 42.17500000054622689, 13.07298590277314254, 93.04388485072563242 ) ) ;
#11304=CARTESIAN_POINT ( 'NONE',  ( 20.85000000109246443, 24.40838939219355197, 84.72553407664153724 ) ) ;
#11311=CARTESIAN_POINT ( 'NONE',  ( 21.20617189303578698, 14.62220435867159374, 151.2938281069642130 ) ) ;
#11312=EDGE_CURVE ( 'NONE', #12151, #7259, #12087, .T. ) ;
#11313=CARTESIAN_POINT ( 'NONE',  ( 10.00000000000000355, 20.00000000000000355, 109.9999999999999858 ) ) ;
#11314=CARTESIAN_POINT ( 'NONE',  ( 20.49999999999998224, 12.11403331821300533, 90.79316153445363113 ) ) ;
#11315=CARTESIAN_POINT ( 'NONE',  ( 24.37500000054622618, 13.07298590277314432, 88.54243821818161564 ) ) ;
#11316=CARTESIAN_POINT ( 'NONE',  ( 26.07500000054622546, 15.71886984736413417, 96.68563167572563088 ) ) ;
#11321=CARTESIAN_POINT ( 'NONE',  ( 37.15000000109246514, 27.88596668178699645, 90.79316153445363113 ) ) ;
#11329=CARTESIAN_POINT ( 'NONE',  ( 31.15000000109246159, 27.88596668178699645, 90.79316153445363113 ) ) ;
#11331=CARTESIAN_POINT ( 'NONE',  ( -50.00000000000001421, 18.00000000000000355, 152.2284161474004520 ) ) ;
#11334=EDGE_CURVE ( 'NONE', #5416, #1035, #11192, .T. ) ;
#11339=CARTESIAN_POINT ( 'NONE',  ( 47.67500000054622689, 24.28113015263587116, 96.68563167572563088 ) ) ;
#11343=ADVANCED_FACE ( 'NONE', ( #7069 ), #2259, .T. ) ;
#11347=CARTESIAN_POINT ( 'NONE',  ( 34.47500000054623115, 13.80429023900056684, 86.29171490190961435 ) ) ;
#11348=CARTESIAN_POINT ( 'NONE',  ( 35.27500000054622120, 26.92701409722686634, 88.54243821818162985 ) ) ;
#11349=CARTESIAN_POINT ( 'NONE',  ( 21.97500000054622760, 15.71886984736413417, 96.68563167572563088 ) ) ;
#11352=CARTESIAN_POINT ( 'NONE',  ( -2.000000000000015543, 20.00000000000000355, 90.79316153445363113 ) ) ;
#11353=DIRECTION ( 'NONE',  ( 0.000000000000000000, 0.000000000000000000, 1.000000000000000000 ) ) ;
#11355=ORIENTED_EDGE ( 'NONE', *, *, #2114, .T. ) ;
#11358=CARTESIAN_POINT ( 'NONE',  ( 25.17500000054622689, 26.19570976099943849, 86.29171490190961435 ) ) ;
#11360=CARTESIAN_POINT ( 'NONE',  ( 46.27500000054622120, 12.34168156654572357, 90.79316153445363113 ) ) ;
#11361=CARTESIAN_POINT ( 'NONE',  ( 27.27500000054622475, 26.92701409722686634, 88.54243821818162985 ) ) ;
#11362=CARTESIAN_POINT ( 'NONE',  ( 32.69999999999999574, 13.62011893735971135, 86.15790661882942914 ) ) ;
#11365=CARTESIAN_POINT ( 'NONE',  ( 40.07500000054623257, 13.80429023900056507, 95.29460816699764791 ) ) ;
#11367=CARTESIAN_POINT ( 'NONE',  ( 47.47500000054623115, 26.19570976099943493, 95.29460816699764791 ) ) ;
#11368=CARTESIAN_POINT ( 'NONE',  ( -27.49999999999999645, 20.00000000000000355, 169.9999999999999716 ) ) ;
#11369=ORIENTED_EDGE ( 'NONE', *, *, #2008, .T. ) ;
#11371=ORIENTED_EDGE ( 'NONE', *, *, #11999, .F. ) ;
#11374=CARTESIAN_POINT ( 'NONE',  ( 27.50000000000000355, 12.50000000000001066, 145.0000000000000000 ) ) ;
#11375=CARTESIAN_POINT ( 'NONE',  ( -7.000000000000006217, 84.49999999999998579, 146.8533255156881978 ) ) ;
#11376=CARTESIAN_POINT ( 'NONE',  ( 43.77500000054621410, 22.36655054427230027, 98.07665518445361386 ) ) ;
#11377=FACE_OUTER_BOUND ( 'NONE', #6423, .T. ) ;
#11379=CARTESIAN_POINT ( 'NONE',  ( 23.67500000054622333, 22.36655054427230027, 98.07665518445361386 ) ) ;
#11380=CARTESIAN_POINT ( 'NONE',  ( 48.39999999999999147, 12.86707612778636012, 93.11078899226572503 ) ) ;
#11383=CARTESIAN_POINT ( 'NONE',  ( 38.45000000109246230, 15.59161060780646046, 84.72553407664153724 ) ) ;
#11384=ORIENTED_EDGE ( 'NONE', *, *, #2837, .T. ) ;
#11385=ADVANCED_FACE ( 'NONE', ( #661 ), #9603, .F. ) ;
#11390=DIRECTION ( 'NONE',  ( -0.000000000000000000, -0.000000000000000000, 1.000000000000000000 ) ) ;
#11391=LINE ( 'NONE', #10308, #7476 ) ;
#11396=CARTESIAN_POINT ( 'NONE',  ( 49.87500000054622262, 20.00000000000000355, 98.07665518445361386 ) ) ;
#11398=CARTESIAN_POINT ( 'NONE',  ( 46.85000000109246798, 24.40838939219355197, 84.72553407664153724 ) ) ;
#11401=AXIS2_PLACEMENT_3D ( 'NONE', #9665, #5094, #6988 ) ;
#11403=DIRECTION ( 'NONE',  ( 1.000000000000000000, -0.000000000000000000, -0.000000000000000000 ) ) ;
#11404=CARTESIAN_POINT ( 'NONE',  ( 36.57500000054621125, 13.80429023900056684, 86.29171490190961435 ) ) ;
#11405=CARTESIAN_POINT ( 'NONE',  ( 22.77500000054622831, 20.00000000000000355, 83.50966788445364841 ) ) ;
#11406=CARTESIAN_POINT ( 'NONE',  ( 10.00000000000001599, 19.48622803733975672, 98.29316153445364534 ) ) ;
#11407=PLANE ( 'NONE',  #2579 ) ;
#11408=EDGE_CURVE ( 'NONE', #5738, #8904, #4822, .T. ) ;
#11412=CARTESIAN_POINT ( 'NONE',  ( 49.99999999999998579, 20.00000000000000355, 90.79316153445363113 ) ) ;
#11419=CARTESIAN_POINT ( 'NONE',  ( 24.67500000054622689, 15.71886984736413773, 84.90069139318163138 ) ) ;
#11422=CARTESIAN_POINT ( 'NONE',  ( 38.17500000054622689, 13.07298590277314254, 93.04388485072563242 ) ) ;
#11424=CARTESIAN_POINT ( 'NONE',  ( 25.37500000054622618, 27.65831843345427998, 90.79316153445363113 ) ) ;
#11425=CARTESIAN_POINT ( 'NONE',  ( 30.29999999999998295, 13.62011893735971135, 95.42841645007781892 ) ) ;
#11426=CARTESIAN_POINT ( 'NONE',  ( 38.57500000054622546, 15.71886984736413773, 84.90069139318163138 ) ) ;
#11428=CARTESIAN_POINT ( 'NONE',  ( 19.85000000109246443, 15.59161060780645691, 96.86078899226572503 ) ) ;
#11433=CARTESIAN_POINT ( 'NONE',  ( 0.000000000000000000, 0.000000000000000000, 0.000000000000000000 ) ) ;
#11434=CARTESIAN_POINT ( 'NONE',  ( 49.87500000054622262, 20.00000000000000355, 98.07665518445361386 ) ) ;
#11436=CARTESIAN_POINT ( 'NONE',  ( 45.97500000054622404, 17.63344945572769973, 98.07665518445361386 ) ) ;
#11437=CARTESIAN_POINT ( 'NONE',  ( 23.65000000109246514, 20.00000000000000355, 98.29316153445363113 ) ) ;
#11438=CARTESIAN_POINT ( 'NONE',  ( 43.17500000054621978, 26.19570976099943493, 86.29171490190961435 ) ) ;
#11439=CARTESIAN_POINT ( 'NONE',  ( 20.97500000054622404, 22.36655054427230382, 83.50966788445364841 ) ) ;
#11440=VECTOR ( 'NONE', #4644, 1000.000000000000000 ) ;
#11441=CARTESIAN_POINT ( 'NONE',  ( 41.19999999999998863, 24.40838939219355197, 84.72553407664153724 ) ) ;
#11442=CARTESIAN_POINT ( 'NONE',  ( -5.000000000000004441, 0.000000000000000000, 69.99999999999998579 ) ) ;
#11444=CARTESIAN_POINT ( 'NONE',  ( 35.25000000109245946, 27.13292387221364876, 93.11078899226573924 ) ) ;
#11445=CARTESIAN_POINT ( 'NONE',  ( -50.00000000000001421, 31.99999999999960565, 124.8533255156881694 ) ) ;
#11447=ORIENTED_EDGE ( 'NONE', *, *, #3831, .T. ) ;
#11448=EDGE_CURVE ( 'NONE', #3939, #1799, #8196, .T. ) ;
#11459=CARTESIAN_POINT ( 'NONE',  ( 22.47500000054623115, 13.80429023900056684, 86.29171490190961435 ) ) ;
#11461=DIRECTION ( 'NONE',  ( 0.000000000000000000, 0.000000000000000000, -1.000000000000000000 ) ) ;
#11464=CARTESIAN_POINT ( 'NONE',  ( 21.29999999999999005, 26.37988106264029398, 86.15790661882942914 ) ) ;
#11465=EDGE_CURVE ( 'NONE', #9270, #5416, #692, .T. ) ;
#11467=CARTESIAN_POINT ( 'NONE',  ( 20.27500000054622831, 12.34168156654572357, 90.79316153445363113 ) ) ;
#11471=CARTESIAN_POINT ( 'NONE',  ( 49.99999999999998579, 22.00000000000000000, 69.99999999999998579 ) ) ;
#11473=DIRECTION ( 'NONE',  ( 1.000000000000000000, -0.000000000000000000, -0.000000000000000000 ) ) ;
#11474=ORIENTED_EDGE ( 'NONE', *, *, #8993, .F. ) ;
#11478=CARTESIAN_POINT ( 'NONE',  ( 29.35000000109245732, 26.37988106264029398, 95.42841645007781892 ) ) ;
#11479=CARTESIAN_POINT ( 'NONE',  ( 41.47500000054623115, 26.19570976099943849, 95.29460816699764791 ) ) ;
#11480=CARTESIAN_POINT ( 'NONE',  ( 28.07500000054622546, 15.71886984736413417, 96.68563167572563088 ) ) ;
#11481=CARTESIAN_POINT ( 'NONE',  ( 26.79999999999998650, 15.59161060780646046, 84.72553407664153724 ) ) ;
#11484=CARTESIAN_POINT ( 'NONE',  ( 31.17500000054622689, 26.92701409722686634, 88.54243821818162985 ) ) ;
#11486=CARTESIAN_POINT ( 'NONE',  ( 49.47500000054621694, 26.19570976099943493, 95.29460816699764791 ) ) ;
#11493=CARTESIAN_POINT ( 'NONE',  ( 42.45000000109246940, 15.59161060780646046, 84.72553407664153724 ) ) ;
#11496=CARTESIAN_POINT ( 'NONE',  ( 41.67500000054622689, 24.28113015263587116, 96.68563167572563088 ) ) ;
#11497=CARTESIAN_POINT ( 'NONE',  ( 20.99999999999998579, 20.00000000000000355, 83.29316153445364534 ) ) ;
#11500=CARTESIAN_POINT ( 'NONE',  ( 42.77500000054622831, 17.63344945572770328, 83.50966788445364841 ) ) ;
#11501=CARTESIAN_POINT ( 'NONE',  ( 48.69999999999998153, 13.62011893735971135, 86.15790661882942914 ) ) ;
#11503=PLANE ( 'NONE',  #5441 ) ;
#11505=CARTESIAN_POINT ( 'NONE',  ( 40.55000000109247082, 17.56310227825321135, 83.29316153445363113 ) ) ;
#11506=ORIENTED_EDGE ( 'NONE', *, *, #8095, .T. ) ;
#11507=DIRECTION ( 'NONE',  ( 0.000000000000000000, 0.000000000000000000, -1.000000000000000000 ) ) ;
#11512=( BOUNDED_CURVE ( )  B_SPLINE_CURVE ( 2, ( #12374, #3674, #1767, #11478, #8564, #7551, #2601, #9339, #10519, #12310, #3733 ),
 .UNSPECIFIED., .F., .F. ) 
 B_SPLINE_CURVE_WITH_KNOTS ( ( 3, 2, 2, 2, 2, 3 ),
 ( 0.6666666666666666297, 0.6733333333333333393, 0.6800000000000000488, 0.6866666666666666474, 0.6933333333333333570, 0.6999999999999999556 ),
 .UNSPECIFIED. ) 
 CURVE ( )  GEOMETRIC_REPRESENTATION_ITEM ( )  RATIONAL_B_SPLINE_CURVE ( ( 1.000000000000000000, 0.9510565162951535312, 1.000000000000000000, 0.9510565162951535312, 1.000000000000000000, 0.9510565162951535312, 1.000000000000000000, 0.9510565162951535312, 1.000000000000000000, 0.9510565162951535312, 1.000000000000000000 ) ) 
 REPRESENTATION_ITEM ( '' )  );
#11513=VECTOR ( 'NONE', #4874, 1000.000000000000000 ) ;
#11515=CARTESIAN_POINT ( 'NONE',  ( 22.09999999999998366, 17.56310227825320425, 98.29316153445363113 ) ) ;
#11518=CARTESIAN_POINT ( 'NONE',  ( 48.65000000109246514, 20.00000000000000355, 83.29316153445364534 ) ) ;
#11519=CARTESIAN_POINT ( 'NONE',  ( 22.27500000054622475, 12.34168156654572535, 90.79316153445363113 ) ) ;
#11521=CARTESIAN_POINT ( 'NONE',  ( -20.27158385259951956, 22.00000000000000000, 152.2284161474004520 ) ) ;
#11522=CARTESIAN_POINT ( 'NONE',  ( -28.50000000000001066, 77.00000000000000000, 104.8533255156881836 ) ) ;
#11528=CARTESIAN_POINT ( 'NONE',  ( 42.85000000109246798, 24.40838939219355197, 84.72553407664153724 ) ) ;
#11530=CARTESIAN_POINT ( 'NONE',  ( 21.57500000054622546, 24.28113015263587116, 96.68563167572563088 ) ) ;
#11532=VECTOR ( 'NONE', #12118, 1000.000000000000000 ) ;
#11533=CARTESIAN_POINT ( 'NONE',  ( 10.00000000000000355, 20.00000000000000355, 98.29316153445363113 ) ) ;
#11535=CARTESIAN_POINT ( 'NONE',  ( -6.500000000000214051, 40.00000000000000000, 26.49999999999998934 ) ) ;
#11536=CARTESIAN_POINT ( 'NONE',  ( -20.27158385259951956, 22.00000000000000000, 170.0000119999999697 ) ) ;
#11537=VECTOR ( 'NONE', #8396, 1000.000000000000000 ) ;
#11538=DIRECTION ( 'NONE',  ( 0.000000000000000000, 0.000000000000000000, -1.000000000000000000 ) ) ;
#11542=CARTESIAN_POINT ( 'NONE',  ( 26.07500000054622546, 15.71886984736413417, 96.68563167572563088 ) ) ;
#11544=CARTESIAN_POINT ( 'NONE',  ( 42.07500000054623257, 13.80429023900056507, 95.29460816699764791 ) ) ;
#11545=CARTESIAN_POINT ( 'NONE',  ( 25.97500000054622049, 17.63344945572769973, 98.07665518445361386 ) ) ;
#11546=CARTESIAN_POINT ( 'NONE',  ( 29.29999999999998650, 26.37988106264029398, 86.15790661882942914 ) ) ;
#11547=CARTESIAN_POINT ( 'NONE',  ( 49.99999999999998579, 18.00000000000000355, 152.2284161474004520 ) ) ;
#11548=CARTESIAN_POINT ( 'NONE',  ( 32.07500000054623257, 13.80429023900056507, 95.29460816699764791 ) ) ;
#11552=EDGE_CURVE ( 'NONE', #12402, #7152, #2999, .T. ) ;
#11553=DIRECTION ( 'NONE',  ( 0.000000000000000000, 1.000000000000000000, 0.000000000000000000 ) ) ;
#11554=ORIENTED_EDGE ( 'NONE', *, *, #5968, .T. ) ;
#11557=CARTESIAN_POINT ( 'NONE',  ( 49.99999999999998579, 20.00000000000000000, 145.0000000000000000 ) ) ;
#11558=CARTESIAN_POINT ( 'NONE',  ( -34.99999999999997868, 20.00000000000000000, 137.5000000000000000 ) ) ;
#11559=FACE_OUTER_BOUND ( 'NONE', #5772, .T. ) ;
#11560=AXIS2_PLACEMENT_3D ( 'NONE', #3363, #1408, #5274 ) ;
#11563=CARTESIAN_POINT ( 'NONE',  ( 47.07500000054622546, 24.28113015263587471, 84.90069139318163138 ) ) ;
#11564=CARTESIAN_POINT ( 'NONE',  ( 49.89999999999998437, 22.43689772174679575, 98.29316153445363113 ) ) ;
#11565=DIRECTION ( 'NONE',  ( -0.000000000000000000, 1.000000000000000000, -0.000000000000000000 ) ) ;
#11566=CARTESIAN_POINT ( 'NONE',  ( 49.17500000054622689, 26.92701409722686634, 88.54243821818162985 ) ) ;
#11569=CARTESIAN_POINT ( 'NONE',  ( 34.25000000109245946, 12.86707612778636012, 88.47553407664152303 ) ) ;
#11572=AXIS2_PLACEMENT_3D ( 'NONE', #1425, #12077, #4456 ) ;
#11575=DIRECTION ( 'NONE',  ( -0.000000000000000000, -0.000000000000000000, 1.000000000000000000 ) ) ;
#11576=EDGE_CURVE ( 'NONE', #9005, #3772, #7822, .T. ) ;
#11579=CARTESIAN_POINT ( 'NONE',  ( 38.67500000054623399, 17.63344945572770328, 83.50966788445364841 ) ) ;
#11585=DIRECTION ( 'NONE',  ( 0.000000000000000000, 0.000000000000000000, -1.000000000000000000 ) ) ;
#11586=CARTESIAN_POINT ( 'NONE',  ( 48.17500000054622689, 13.80429023900056507, 95.29460816699764791 ) ) ;
#11590=ORIENTED_EDGE ( 'NONE', *, *, #6688, .F. ) ;
#11592=( BOUNDED_CURVE ( )  B_SPLINE_CURVE ( 2, ( #1632, #742, #7531, #3409, #1573, #5386, #11208, #9257, #11398, #9440, #10313 ),
 .UNSPECIFIED., .F., .F. ) 
 B_SPLINE_CURVE_WITH_KNOTS ( ( 3, 2, 2, 2, 2, 3 ),
 ( 0.06666666666666672125, 0.07333333333333338921, 0.08000000000000007105, 0.08666666666666673902, 0.09333333333333342086, 0.1000000000000000888 ),
 .UNSPECIFIED. ) 
 CURVE ( )  GEOMETRIC_REPRESENTATION_ITEM ( )  RATIONAL_B_SPLINE_CURVE ( ( 0.9999999999999995559, 0.9510565162951539753, 1.000000000000000000, 0.9510565162951535312, 1.000000000000000000, 0.9510565162951535312, 1.000000000000000000, 0.9510565162951535312, 1.000000000000000000, 0.9510565162951529761, 1.000000000000000666 ) ) 
 REPRESENTATION_ITEM ( '' )  );
#11593=CARTESIAN_POINT ( 'NONE',  ( 43.25000000109246656, 27.13292387221364876, 93.11078899226573924 ) ) ;
#11594=CARTESIAN_POINT ( 'NONE',  ( -33.79382810696421302, 25.37779564132840804, 151.2938281069642130 ) ) ;
#11598=CARTESIAN_POINT ( 'NONE',  ( 19.77500000054622831, 20.00000000000000355, 98.07665518445361386 ) ) ;
#11604=EDGE_CURVE ( 'NONE', #10983, #8716, #9606, .T. ) ;
#11605=CARTESIAN_POINT ( 'NONE',  ( 28.17500000054621978, 13.80429023900056507, 95.29460816699764791 ) ) ;
#11606=DIRECTION ( 'NONE',  ( 0.000000000000000000, 0.000000000000000000, -1.000000000000000000 ) ) ;
#11608=EDGE_CURVE ( 'NONE', #7259, #6104, #152, .T. ) ;
#11609=CARTESIAN_POINT ( 'NONE',  ( 38.37500000054622973, 13.07298590277314432, 88.54243821818161564 ) ) ;
#11610=CARTESIAN_POINT ( 'NONE',  ( 30.67500000054622333, 15.71886984736413773, 84.90069139318163138 ) ) ;
#11611=CARTESIAN_POINT ( 'NONE',  ( 23.59999999999999076, 27.13292387221364876, 93.11078899226573924 ) ) ;
#11612=CARTESIAN_POINT ( 'NONE',  ( 34.39999999999998437, 12.86707612778636012, 93.11078899226572503 ) ) ;
#11613=CARTESIAN_POINT ( 'NONE',  ( 33.37500000054622973, 26.92701409722686634, 93.04388485072563242 ) ) ;
#11616=ORIENTED_EDGE ( 'NONE', *, *, #1352, .T. ) ;
#11619=AXIS2_PLACEMENT_3D ( 'NONE', #4484, #7400, #9317 ) ;
#11621=FACE_OUTER_BOUND ( 'NONE', #1941, .T. ) ;
#11624=CARTESIAN_POINT ( 'NONE',  ( 42.97500000054622404, 22.36655054427230382, 83.50966788445364841 ) ) ;
#11625=CARTESIAN_POINT ( 'NONE',  ( -2.000000000000015543, 20.00000000000000355, 90.79316153445363113 ) ) ;
#11626=EDGE_CURVE ( 'NONE', #5275, #4582, #4131, .T. ) ;
#11628=CARTESIAN_POINT ( 'NONE',  ( 45.57500000054621836, 26.19570976099943493, 95.29460816699764791 ) ) ;
#11629=CARTESIAN_POINT ( 'NONE',  ( 46.69999999999998153, 13.62011893735971135, 86.15790661882942914 ) ) ;
#11631=CARTESIAN_POINT ( 'NONE',  ( 45.69999999999998863, 26.37988106264029398, 95.42841645007781892 ) ) ;
#11635=EDGE_CURVE ( 'NONE', #2031, #7888, #3451, .T. ) ;
#11636=CARTESIAN_POINT ( 'NONE',  ( 32.35000000109246088, 13.62011893735971135, 86.15790661882942914 ) ) ;
#11640=DIRECTION ( 'NONE',  ( -1.000000000000000000, 0.000000000000000000, 0.000000000000000000 ) ) ;
#11643=CARTESIAN_POINT ( 'NONE',  ( 47.99999999999998579, 20.00000000000000355, 98.29316153445363113 ) ) ;
#11644=CARTESIAN_POINT ( 'NONE',  ( 34.57500000054623257, 15.71886984736413773, 84.90069139318163138 ) ) ;
#11645=CARTESIAN_POINT ( 'NONE',  ( 40.97500000054622404, 22.36655054427230382, 83.50966788445364841 ) ) ;
#11649=ORIENTED_EDGE ( 'NONE', *, *, #5104, .T. ) ;
#11650=EDGE_CURVE ( 'NONE', #8904, #9005, #777, .T. ) ;
#11652=EDGE_LOOP ( 'NONE', ( #6872, #9020, #654, #10855 ) ) ;
#11657=ORIENTED_EDGE ( 'NONE', *, *, #7312, .F. ) ;
#11663=CARTESIAN_POINT ( 'NONE',  ( 7.615685201709251118, 26.48948478036892595, 94.58229401248311774 ) ) ;
#11666=CARTESIAN_POINT ( 'NONE',  ( -6.999999999999999112, 92.00000000000000000, 166.8533255156881694 ) ) ;
#11669=DIRECTION ( 'NONE',  ( -1.000000000000000000, 0.000000000000000000, 0.000000000000000000 ) ) ;
#11670=ORIENTED_EDGE ( 'NONE', *, *, #5505, .T. ) ;
#11674=CARTESIAN_POINT ( 'NONE',  ( 22.47500000054622404, 13.07298590277314432, 88.54243821818161564 ) ) ;
#11675=CARTESIAN_POINT ( 'NONE',  ( 48.77500000054623541, 17.63344945572770328, 83.50966788445364841 ) ) ;
#11676=CARTESIAN_POINT ( 'NONE',  ( 38.57500000054622546, 15.71886984736413773, 84.90069139318163138 ) ) ;
#11677=CARTESIAN_POINT ( 'NONE',  ( 20.37500000054621907, 12.34168156654572535, 90.79316153445363113 ) ) ;
#11678=CARTESIAN_POINT ( 'NONE',  ( 22.39999999999998437, 12.86707612778636012, 93.11078899226572503 ) ) ;
#11679=( LENGTH_UNIT ( ) NAMED_UNIT ( * ) SI_UNIT ( .MILLI., .METRE. ) );
#11680=CARTESIAN_POINT ( 'NONE',  ( 31.37500000054622973, 26.92701409722686634, 93.04388485072563242 ) ) ;
#11684=LINE ( 'NONE', #4958, #7314 ) ;
#11688=CARTESIAN_POINT ( 'NONE',  ( 38.77500000054622831, 17.63344945572770328, 83.50966788445364841 ) ) ;
#11689=FACE_OUTER_BOUND ( 'NONE', #11011, .T. ) ;
#11690=CARTESIAN_POINT ( 'NONE',  ( 44.29999999999999716, 13.62011893735971135, 95.42841645007781892 ) ) ;
#11692=CARTESIAN_POINT ( 'NONE',  ( -50.00000000000001421, 92.00000000000000000, 69.99999999999998579 ) ) ;
#11693=ADVANCED_FACE ( 'NONE', ( #6281 ), #6401, .F. ) ;
#11695=VERTEX_POINT ( 'NONE', #1642 ) ;
#11696=CARTESIAN_POINT ( 'NONE',  ( 30.55000000109246372, 17.56310227825321135, 83.29316153445363113 ) ) ;
#11699=ADVANCED_FACE ( 'NONE', ( #7479 ), #7416, .F. ) ;
#11704=CARTESIAN_POINT ( 'NONE',  ( 48.29999999999999005, 13.62011893735970958, 95.42841645007781892 ) ) ;
#11706=CARTESIAN_POINT ( 'NONE',  ( 37.67500000054623399, 22.36655054427230027, 98.07665518445361386 ) ) ;
#11707=CARTESIAN_POINT ( 'NONE',  ( 32.87500000054622262, 20.00000000000000355, 83.50966788445364841 ) ) ;
#11708=CARTESIAN_POINT ( 'NONE',  ( 44.45000000109246230, 15.59161060780646046, 84.72553407664153724 ) ) ;
#11709=CYLINDRICAL_SURFACE ( 'NONE', #774, 7.499999999999992895 ) ;
#11710=ORIENTED_EDGE ( 'NONE', *, *, #490, .T. ) ;
#11711=CARTESIAN_POINT ( 'NONE',  ( 48.55000000109246372, 17.56310227825321135, 83.29316153445363113 ) ) ;
#11712=CARTESIAN_POINT ( 'NONE',  ( -6.999999999999999112, 55.00000000000000000, 147.8533255156883399 ) ) ;
#11713=ORIENTED_EDGE ( 'NONE', *, *, #4489, .T. ) ;
#11715=( BOUNDED_CURVE ( )  B_SPLINE_CURVE ( 2, ( #5668, #12264, #11493, #6602, #3812, #5604, #837, #12448, #2617, #7630, #655 ),
 .UNSPECIFIED., .F., .F. ) 
 B_SPLINE_CURVE_WITH_KNOTS ( ( 3, 2, 2, 2, 2, 3 ),
 ( 0.2333333333333333093, 0.2399999999999999634, 0.2466666666666666452, 0.2533333333333333548, 0.2600000000000000089, 0.2666666666666666630 ),
 .UNSPECIFIED. ) 
 CURVE ( )  GEOMETRIC_REPRESENTATION_ITEM ( )  RATIONAL_B_SPLINE_CURVE ( ( 1.000000000000000222, 0.9510565162951533091, 1.000000000000000000, 0.9510565162951535312, 1.000000000000000000, 0.9510565162951535312, 1.000000000000000000, 0.9510565162951535312, 1.000000000000000000, 0.9510565162951535312, 1.000000000000000000 ) ) 
 REPRESENTATION_ITEM ( '' )  );
#11719=LINE ( 'NONE', #10961, #1162 ) ;
#11722=CARTESIAN_POINT ( 'NONE',  ( 49.99999999999998579, 18.00000000000000355, 169.9999999999999716 ) ) ;
#11723=CARTESIAN_POINT ( 'NONE',  ( 9.620555948181120698, 22.73892591121550666, 97.77955592743285251 ) ) ;
#11725=CARTESIAN_POINT ( 'NONE',  ( -2.000000000000015543, 20.00000000000000355, 83.29316153445364534 ) ) ;
#11727=EDGE_CURVE ( 'NONE', #3312, #5544, #453, .T. ) ;
#11729=VECTOR ( 'NONE', #2451, 1000.000000000000000 ) ;
#11730=CARTESIAN_POINT ( 'NONE',  ( 41.57500000054623257, 24.28113015263587116, 96.68563167572563088 ) ) ;
#11731=DIRECTION ( 'NONE',  ( -0.000000000000000000, -0.000000000000000000, 1.000000000000000000 ) ) ;
#11736=CARTESIAN_POINT ( 'NONE',  ( 21.07500000054622191, 24.28113015263587471, 84.90069139318163138 ) ) ;
#11738=CARTESIAN_POINT ( 'NONE',  ( 30.17500000054623044, 13.07298590277314254, 93.04388485072563242 ) ) ;
#11741=CARTESIAN_POINT ( 'NONE',  ( 24.59999999999998721, 12.86707612778636012, 88.47553407664152303 ) ) ;
#11742=CARTESIAN_POINT ( 'NONE',  ( 35.27500000054622831, 27.65831843345427998, 90.79316153445363113 ) ) ;
#11746=LINE ( 'NONE', #6982, #10551 ) ;
#11747=ORIENTED_EDGE ( 'NONE', *, *, #396, .F. ) ;
#11750=CARTESIAN_POINT ( 'NONE',  ( 40.47500000054622404, 13.07298590277314432, 88.54243821818161564 ) ) ;
#11751=DIRECTION ( 'NONE',  ( 0.000000000000000000, 0.000000000000000000, -1.000000000000000000 ) ) ;
#11752=CARTESIAN_POINT ( 'NONE',  ( 39.87500000054622262, 20.00000000000000355, 98.07665518445361386 ) ) ;
#11753=CARTESIAN_POINT ( 'NONE',  ( 45.59999999999998721, 27.13292387221364876, 93.11078899226573924 ) ) ;
#11756=DIRECTION ( 'NONE',  ( 0.000000000000000000, 0.000000000000000000, -1.000000000000000000 ) ) ;
#11758=CARTESIAN_POINT ( 'NONE',  ( 34.05000000109246372, 12.86707612778636012, 93.11078899226572503 ) ) ;
#11760=ORIENTED_EDGE ( 'NONE', *, *, #5503, .F. ) ;
#11762=AXIS2_PLACEMENT_3D ( 'NONE', #10578, #5895, #1076 ) ;
#11766=CARTESIAN_POINT ( 'NONE',  ( -2.000000000000015543, 20.00000000000000355, 83.29316153445364534 ) ) ;
#11767=CARTESIAN_POINT ( 'NONE',  ( 29.87500000054622618, 17.63344945572769973, 98.07665518445361386 ) ) ;
#11768=CARTESIAN_POINT ( 'NONE',  ( 33.07500000054622546, 24.28113015263587471, 84.90069139318163138 ) ) ;
#11770=CARTESIAN_POINT ( 'NONE',  ( 31.00470515163596730, 27.49999999999999645, 148.5047051516359318 ) ) ;
#11773=CARTESIAN_POINT ( 'NONE',  ( 48.37500000054621552, 12.34168156654572357, 90.79316153445363113 ) ) ;
#11774=CARTESIAN_POINT ( 'NONE',  ( 47.35000000109245377, 26.37988106264029398, 95.42841645007781892 ) ) ;
#11775=ORIENTED_EDGE ( 'NONE', *, *, #11212, .F. ) ;
#11776=CARTESIAN_POINT ( 'NONE',  ( 34.99999999999999289, 15.60660171779822569, 137.5000000000000000 ) ) ;
#11777=VERTEX_POINT ( 'NONE', #1464 ) ;
#11778=FACE_OUTER_BOUND ( 'NONE', #3908, .T. ) ;
#11782=EDGE_CURVE ( 'NONE', #1317, #9736, #3039, .T. ) ;
#11783=CARTESIAN_POINT ( 'NONE',  ( 8.867874694687726489, 24.64263244605503900, 96.70324107235252598 ) ) ;
#11784=DIRECTION ( 'NONE',  ( 1.000000000000000000, -0.000000000000000000, -0.000000000000000000 ) ) ;
#11785=CARTESIAN_POINT ( 'NONE',  ( -50.00000000000001421, 18.00000000000000355, 188.4007504869563263 ) ) ;
#11786=CARTESIAN_POINT ( 'NONE',  ( 4.999999999999999112, 22.00000000000000000, 218.7511230907454944 ) ) ;
#11788=CARTESIAN_POINT ( 'NONE',  ( 44.27500000054622120, 12.34168156654572535, 90.79316153445363113 ) ) ;
#11795=CARTESIAN_POINT ( 'NONE',  ( 35.37500000054622973, 26.92701409722686634, 93.04388485072563242 ) ) ;
#11796=CARTESIAN_POINT ( 'NONE',  ( 23.77500000054622475, 22.36655054427230027, 98.07665518445361386 ) ) ;
#11797=CARTESIAN_POINT ( 'NONE',  ( 24.39999999999998792, 12.86707612778636012, 93.11078899226572503 ) ) ;
#11799=CARTESIAN_POINT ( 'NONE',  ( 25.27500000054622475, 27.65831843345427998, 90.79316153445363113 ) ) ;
#11806=ORIENTED_EDGE ( 'NONE', *, *, #8117, .F. ) ;
#11807=( NAMED_UNIT ( * ) SI_UNIT ( $, .STERADIAN. ) SOLID_ANGLE_UNIT ( ) );
#11809=AXIS2_PLACEMENT_3D ( 'NONE', #4069, #7947, #274 ) ;
#11810=CARTESIAN_POINT ( 'NONE',  ( -2.000000000000015543, 20.00000000000000355, 90.79316153445363113 ) ) ;
#11812=CARTESIAN_POINT ( 'NONE',  ( 36.87500000054622262, 20.00000000000000355, 83.50966788445364841 ) ) ;
#11813=CARTESIAN_POINT ( 'NONE',  ( 0.000000000000000000, 92.00000000000000000, 0.000000000000000000 ) ) ;
#11814=CARTESIAN_POINT ( 'NONE',  ( 26.59999999999998721, 12.86707612778636012, 88.47553407664152303 ) ) ;
#11815=CARTESIAN_POINT ( 'NONE',  ( 42.59999999999998721, 12.86707612778636012, 88.47553407664152303 ) ) ;
#11816=CARTESIAN_POINT ( 'NONE',  ( 39.29999999999999005, 26.37988106264029398, 86.15790661882942914 ) ) ;
#11819=VECTOR ( 'NONE', #6838, 1000.000000000000000 ) ;
#11820=CARTESIAN_POINT ( 'NONE',  ( 31.85000000109246443, 15.59161060780645691, 96.86078899226572503 ) ) ;
#11822=VERTEX_POINT ( 'NONE', #5768 ) ;
#11823=VERTEX_POINT ( 'NONE', #54 ) ;
#11827=AXIS2_PLACEMENT_3D ( 'NONE', #9183, #4291, #5504 ) ;
#11829=CARTESIAN_POINT ( 'NONE',  ( 31.27500000054622831, 27.65831843345427998, 90.79316153445363113 ) ) ;
#11830=CARTESIAN_POINT ( 'NONE',  ( 28.97500000054622404, 22.36655054427230382, 83.50966788445364841 ) ) ;
#11834=DIRECTION ( 'NONE',  ( -0.000000000000000000, -0.000000000000000000, 1.000000000000000000 ) ) ;
#11835=ORIENTED_EDGE ( 'NONE', *, *, #3098, .T. ) ;
#11836=CARTESIAN_POINT ( 'NONE',  ( 48.17500000054622689, 13.80429023900056507, 95.29460816699764791 ) ) ;
#11837=CARTESIAN_POINT ( 'NONE',  ( 49.25000000109246656, 27.13292387221364876, 93.11078899226573924 ) ) ;
#11838=DIRECTION ( 'NONE',  ( 1.000000000000000000, -0.000000000000000000, -0.000000000000000000 ) ) ;
#11844=CARTESIAN_POINT ( 'NONE',  ( -2.000000000000015543, 20.00000000000000355, 90.79316153445363113 ) ) ;
#11848=LINE ( 'NONE', #9822, #3786 ) ;
#11849=CARTESIAN_POINT ( 'NONE',  ( 7.063104035062243824, 27.07982170659911958, 93.28061500048886501 ) ) ;
#11855=CARTESIAN_POINT ( 'NONE',  ( 44.77500000054623541, 20.00000000000000355, 83.50966788445364841 ) ) ;
#11857=ORIENTED_EDGE ( 'NONE', *, *, #10317, .T. ) ;
#11861=CIRCLE ( 'NONE', #4555, 7.500000000000007105 ) ;
#11862=CARTESIAN_POINT ( 'NONE',  ( 21.77500000054622475, 22.36655054427230027, 98.07665518445361386 ) ) ;
#11863=CARTESIAN_POINT ( 'NONE',  ( 45.07500000054622546, 24.28113015263587471, 84.90069139318163138 ) ) ;
#11865=CARTESIAN_POINT ( 'NONE',  ( 36.17500000054622689, 13.07298590277314254, 93.04388485072563242 ) ) ;
#11866=CARTESIAN_POINT ( 'NONE',  ( 24.47500000054622404, 13.07298590277314432, 88.54243821818161564 ) ) ;
#11867=CARTESIAN_POINT ( 'NONE',  ( 26.29999999999998295, 13.62011893735971135, 95.42841645007781892 ) ) ;
#11870=CARTESIAN_POINT ( 'NONE',  ( 49.39999999999998437, 27.13292387221364876, 88.47553407664153724 ) ) ;
#11871=CARTESIAN_POINT ( 'NONE',  ( 27.97500000054623115, 15.71886984736413417, 96.68563167572563088 ) ) ;
#11872=ORIENTED_EDGE ( 'NONE', *, *, #94, .T. ) ;
#11873=CARTESIAN_POINT ( 'NONE',  ( 32.75000000109245946, 22.43689772174679575, 83.29316153445363113 ) ) ;
#11874=EDGE_LOOP ( 'NONE', ( #5169, #7296, #4834, #10155 ) ) ;
#11875=ORIENTED_EDGE ( 'NONE', *, *, #12350, .T. ) ;
#11876=CARTESIAN_POINT ( 'NONE',  ( -20.27158385259951956, 22.00000000000000000, 152.2284161474004520 ) ) ;
#11877=VERTEX_POINT ( 'NONE', #9636 ) ;
#11880=CARTESIAN_POINT ( 'NONE',  ( 39.57500000054622546, 26.19570976099943849, 95.29460816699764791 ) ) ;
#11881=CARTESIAN_POINT ( 'NONE',  ( 39.85000000109246798, 15.59161060780645691, 96.86078899226572503 ) ) ;
#11882=ADVANCED_FACE ( 'NONE', ( #5828 ), #5640, .T. ) ;
#11884=CARTESIAN_POINT ( 'NONE',  ( 38.77500000054622831, 17.63344945572770328, 83.50966788445364841 ) ) ;
#11885=CARTESIAN_POINT ( 'NONE',  ( 43.19999999999998863, 24.40838939219355197, 84.72553407664153724 ) ) ;
#11886=CARTESIAN_POINT ( 'NONE',  ( 44.97500000054623115, 24.28113015263587471, 84.90069139318163138 ) ) ;
#11887=ORIENTED_EDGE ( 'NONE', *, *, #9992, .F. ) ;
#11888=CARTESIAN_POINT ( 'NONE',  ( 26.75000000109245946, 22.43689772174679575, 83.29316153445363113 ) ) ;
#11889=LINE ( 'NONE', #3195, #8921 ) ;
#11892=EDGE_CURVE ( 'NONE', #2741, #11966, #813, .T. ) ;
#11893=CARTESIAN_POINT ( 'NONE',  ( 49.99999999999998579, 0.000000000000000000, 82.99999999999995737 ) ) ;
#11897=DIRECTION ( 'NONE',  ( 1.000000000000000000, -0.000000000000000000, -0.000000000000000000 ) ) ;
#11899=CARTESIAN_POINT ( 'NONE',  ( 28.27500000054622475, 12.34168156654572535, 90.79316153445363113 ) ) ;
#11900=CARTESIAN_POINT ( 'NONE',  ( 28.47500000054622404, 13.07298590277314432, 88.54243821818161564 ) ) ;
#11904=ORIENTED_EDGE ( 'NONE', *, *, #4951, .F. ) ;
#11913=AXIS2_PLACEMENT_3D ( 'NONE', #79, #5975, #4839 ) ;
#11914=CARTESIAN_POINT ( 'NONE',  ( 6.731970158774189805, 27.39502174583683569, 89.51723080467371574 ) ) ;
#11919=CARTESIAN_POINT ( 'NONE',  ( 43.87500000054622973, 17.63344945572769973, 98.07665518445361386 ) ) ;
#11922=VECTOR ( 'NONE', #10482, 1000.000000000000000 ) ;
#11925=CARTESIAN_POINT ( 'NONE',  ( 21.97500000054622049, 17.63344945572769973, 98.07665518445361386 ) ) ;
#11926=CARTESIAN_POINT ( 'NONE',  ( 42.07500000054622546, 15.71886984736413417, 96.68563167572563088 ) ) ;
#11927=CARTESIAN_POINT ( 'NONE',  ( 30.87500000054622618, 22.36655054427230382, 83.50966788445364841 ) ) ;
#11928=( BOUNDED_CURVE ( )  B_SPLINE_CURVE ( 3, ( #994, #9747, #232, #7714 ),
 .UNSPECIFIED., .F., .F. ) 
 B_SPLINE_CURVE_WITH_KNOTS ( ( 4, 4 ),
 ( -8.881784197001252323E-16, 1.570796326794896558 ),
 .UNSPECIFIED. ) 
 CURVE ( )  GEOMETRIC_REPRESENTATION_ITEM ( )  RATIONAL_B_SPLINE_CURVE ( ( 1.000000000000000000, 0.8047378541243648264, 0.8047378541243648264, 1.000000000000000000 ) ) 
 REPRESENTATION_ITEM ( '' )  );
#11932=CARTESIAN_POINT ( 'NONE',  ( 49.69999999999998863, 26.37988106264029398, 95.42841645007781892 ) ) ;
#11933=CARTESIAN_POINT ( 'NONE',  ( 23.77500000054622831, 20.00000000000000355, 98.07665518445361386 ) ) ;
#11934=ORIENTED_EDGE ( 'NONE', *, *, #10015, .F. ) ;
#11935=CARTESIAN_POINT ( 'NONE',  ( 23.35000000109246443, 26.37988106264029398, 95.42841645007781892 ) ) ;
#11936=ORIENTED_EDGE ( 'NONE', *, *, #8133, .F. ) ;
#11940=DIRECTION ( 'NONE',  ( 0.000000000000000000, 0.000000000000000000, -1.000000000000000000 ) ) ;
#11942=CARTESIAN_POINT ( 'NONE',  ( 37.17500000054621978, 26.19570976099943849, 86.29171490190961435 ) ) ;
#11944=CARTESIAN_POINT ( 'NONE',  ( 20.65000000109246514, 20.00000000000000355, 83.29316153445364534 ) ) ;
#11945=CARTESIAN_POINT ( 'NONE',  ( 37.87500000054622262, 20.00000000000000355, 98.07665518445361386 ) ) ;
#11946=CARTESIAN_POINT ( 'NONE',  ( 39.19999999999998153, 24.40838939219355197, 84.72553407664153724 ) ) ;
#11948=CARTESIAN_POINT ( 'NONE',  ( 45.17500000054622689, 26.92701409722686634, 88.54243821818162985 ) ) ;
#11950=CARTESIAN_POINT ( 'NONE',  ( 25.95000000109246585, 13.62011893735971135, 95.42841645007781892 ) ) ;
#11955=FACE_OUTER_BOUND ( 'NONE', #3574, .T. ) ;
#11956=CARTESIAN_POINT ( 'NONE',  ( 40.95000000109246940, 26.37988106264029398, 86.15790661882942914 ) ) ;
#11957=CARTESIAN_POINT ( 'NONE',  ( 25.29999999999998295, 26.37988106264029398, 86.15790661882942914 ) ) ;
#11958=CARTESIAN_POINT ( 'NONE',  ( 31.47500000054623115, 26.19570976099943493, 95.29460816699764791 ) ) ;
#11959=CARTESIAN_POINT ( 'NONE',  ( 32.77500000054622831, 17.63344945572770328, 83.50966788445364841 ) ) ;
#11961=PLANE ( 'NONE',  #8595 ) ;
#11962=LINE ( 'NONE', #11007, #2790 ) ;
#11964=CARTESIAN_POINT ( 'NONE',  ( 42.95000000109246940, 26.37988106264029398, 86.15790661882942914 ) ) ;
#11966=VERTEX_POINT ( 'NONE', #3223 ) ;
#11978=CARTESIAN_POINT ( 'NONE',  ( 37.75000000109245946, 17.56310227825323977, 98.29316153445364534 ) ) ;
#11979=CARTESIAN_POINT ( 'NONE',  ( -50.00000000000001421, 20.00000000000000000, 145.0000000000000000 ) ) ;
#11988=CARTESIAN_POINT ( 'NONE',  ( 45.47500000054622404, 26.92701409722686634, 93.04388485072563242 ) ) ;
#11990=CARTESIAN_POINT ( 'NONE',  ( 26.57500000054622902, 15.71886984736413773, 84.90069139318163138 ) ) ;
#11991=CARTESIAN_POINT ( 'NONE',  ( 9.240229740357481347, 16.15179536300817986, 97.24847665116462281 ) ) ;
#11992=CARTESIAN_POINT ( 'NONE',  ( 19.99999999999998579, 20.00000000000000355, 98.29316153445363113 ) ) ;
#11994=CARTESIAN_POINT ( 'NONE',  ( 25.87500000054622262, 17.63344945572769973, 98.07665518445361386 ) ) ;
#11997=ORIENTED_EDGE ( 'NONE', *, *, #11727, .F. ) ;
#11999=EDGE_CURVE ( 'NONE', #8904, #12216, #4173, .T. ) ;
#12001=ORIENTED_EDGE ( 'NONE', *, *, #561, .T. ) ;
#12002=( BOUNDED_CURVE ( )  B_SPLINE_CURVE ( 3, ( #4365, #3095, #3163, #7028 ),
 .UNSPECIFIED., .F., .F. ) 
 B_SPLINE_CURVE_WITH_KNOTS ( ( 4, 4 ),
 ( -8.881784197001252323E-16, 1.570796326794896558 ),
 .UNSPECIFIED. ) 
 CURVE ( )  GEOMETRIC_REPRESENTATION_ITEM ( )  RATIONAL_B_SPLINE_CURVE ( ( 1.000000000000000000, 0.8047378541243648264, 0.8047378541243648264, 1.000000000000000000 ) ) 
 REPRESENTATION_ITEM ( '' )  );
#12003=CARTESIAN_POINT ( 'NONE',  ( 30.87500000054622618, 20.00000000000000355, 83.50966788445364841 ) ) ;
#12006=CARTESIAN_POINT ( 'NONE',  ( 40.67500000054622689, 15.71886984736413773, 84.90069139318163138 ) ) ;
#12007=CARTESIAN_POINT ( 'NONE',  ( 35.09999999999998721, 22.43689772174679575, 83.29316153445363113 ) ) ;
#12008=CARTESIAN_POINT ( 'NONE',  ( 43.17500000054622689, 26.92701409722686634, 88.54243821818162985 ) ) ;
#12010=CARTESIAN_POINT ( 'NONE',  ( 22.65000000109246514, 20.00000000000000355, 83.29316153445364534 ) ) ;
#12016=LINE ( 'NONE', #7894, #7280 ) ;
#12019=CARTESIAN_POINT ( 'NONE',  ( 25.59999999999998721, 27.13292387221364876, 93.11078899226573924 ) ) ;
#12020=CARTESIAN_POINT ( 'NONE',  ( 31.97500000054623470, 15.71886984736413417, 96.68563167572563088 ) ) ;
#12021=CARTESIAN_POINT ( 'NONE',  ( 22.47500000054622404, 13.07298590277314432, 88.54243821818161564 ) ) ;
#12022=ADVANCED_FACE ( 'NONE', ( #3978 ), #9063, .F. ) ;
#12024=CARTESIAN_POINT ( 'NONE',  ( 49.93750000027311131, 20.00000000000000355, 98.18490835945361539 ) ) ;
#12025=CARTESIAN_POINT ( 'NONE',  ( -2.000000000000015543, 20.00000000000000355, 83.29316153445364534 ) ) ;
#12026=ORIENTED_EDGE ( 'NONE', *, *, #11635, .T. ) ;
#12027=CARTESIAN_POINT ( 'NONE',  ( 44.75000000109245946, 22.43689772174679575, 83.29316153445363113 ) ) ;
#12029=ORIENTED_EDGE ( 'NONE', *, *, #1952, .F. ) ;
#12039=CARTESIAN_POINT ( 'NONE',  ( -6.999999999999999112, 77.00000000000000000, 146.8533255156881978 ) ) ;
#12049=EDGE_CURVE ( 'NONE', #949, #10115, #8802, .T. ) ;
#12054=CARTESIAN_POINT ( 'NONE',  ( 45.27500000054622831, 26.92701409722686634, 88.54243821818162985 ) ) ;
#12055=CARTESIAN_POINT ( 'NONE',  ( 26.87500000054622618, 22.36655054427230382, 83.50966788445364841 ) ) ;
#12057=DIRECTION ( 'NONE',  ( -1.000000000000000000, 0.000000000000000000, 0.000000000000000000 ) ) ;
#12058=CARTESIAN_POINT ( 'NONE',  ( 35.29999999999998295, 26.37988106264029398, 86.15790661882942914 ) ) ;
#12059=CARTESIAN_POINT ( 'NONE',  ( -111.8465843842649292, 77.00000000000000000, 101.8533255156881978 ) ) ;
#12067=CARTESIAN_POINT ( 'NONE',  ( 28.97500000054622404, 22.36655054427230382, 83.50966788445364841 ) ) ;
#12069=CARTESIAN_POINT ( 'NONE',  ( 46.47500000054623115, 13.80429023900056684, 86.29171490190961435 ) ) ;
#12070=CARTESIAN_POINT ( 'NONE',  ( 31.17500000054621978, 26.19570976099943493, 86.29171490190961435 ) ) ;
#12071=CARTESIAN_POINT ( 'NONE',  ( 34.99999999999999289, 20.00000000000000355, 83.29316153445364534 ) ) ;
#12072=CARTESIAN_POINT ( 'NONE',  ( 43.97500000054623115, 15.71886984736413417, 96.68563167572563088 ) ) ;
#12074=CARTESIAN_POINT ( 'NONE',  ( 23.05000000109246372, 27.13292387221364876, 88.47553407664153724 ) ) ;
#12077=DIRECTION ( 'NONE',  ( 1.000000000000000000, -0.000000000000000000, -0.000000000000000000 ) ) ;
#12079=ORIENTED_EDGE ( 'NONE', *, *, #6207, .T. ) ;
#12082=CARTESIAN_POINT ( 'NONE',  ( 35.85000000109246798, 15.59161060780645691, 96.86078899226572503 ) ) ;
#12085=CARTESIAN_POINT ( 'NONE',  ( 22.67500000054622333, 17.63344945572770328, 83.50966788445364841 ) ) ;
#12086=CARTESIAN_POINT ( 'NONE',  ( 25.27500000054622475, 26.92701409722686634, 88.54243821818162985 ) ) ;
#12087=LINE ( 'NONE', #3206, #3127 ) ;
#12090=CARTESIAN_POINT ( 'NONE',  ( 41.55000000109246372, 22.43689772174679575, 98.29316153445363113 ) ) ;
#12093=CARTESIAN_POINT ( 'NONE',  ( 47.69999999999999574, 26.37988106264029398, 95.42841645007781892 ) ) ;
#12094=ORIENTED_EDGE ( 'NONE', *, *, #11782, .T. ) ;
#12098=CARTESIAN_POINT ( 'NONE',  ( 25.65000000109246514, 20.00000000000000355, 98.29316153445363113 ) ) ;
#12099=CARTESIAN_POINT ( 'NONE',  ( 20.87500000054622973, 22.36655054427230382, 83.50966788445364841 ) ) ;
#12102=EDGE_CURVE ( 'NONE', #8208, #5738, #9124, .T. ) ;
#12114=CARTESIAN_POINT ( 'NONE',  ( 44.67500000054621978, 15.71886984736413773, 84.90069139318163138 ) ) ;
#12115=CARTESIAN_POINT ( 'NONE',  ( 23.67500000054622333, 22.36655054427230027, 98.07665518445361386 ) ) ;
#12118=DIRECTION ( 'NONE',  ( 1.000000000000000000, -0.000000000000000000, -0.000000000000000000 ) ) ;
#12119=CARTESIAN_POINT ( 'NONE',  ( 33.69999999999998153, 26.37988106264029398, 95.42841645007781892 ) ) ;
#12121=ORIENTED_EDGE ( 'NONE', *, *, #1399, .T. ) ;
#12122=CARTESIAN_POINT ( 'NONE',  ( 23.55000000109246017, 22.43689772174679575, 98.29316153445363113 ) ) ;
#12123=DIRECTION ( 'NONE',  ( 0.4999999999999892308, 0.000000000000000000, 0.8660254037844448138 ) ) ;
#12127=CARTESIAN_POINT ( 'NONE',  ( 30.97500000054622404, 22.36655054427230382, 83.50966788445364841 ) ) ;
#12129=CARTESIAN_POINT ( 'NONE',  ( 44.17500000054622689, 13.07298590277314254, 93.04388485072563242 ) ) ;
#12130=CARTESIAN_POINT ( 'NONE',  ( 32.37500000054621552, 12.34168156654572535, 90.79316153445363113 ) ) ;
#12131=CARTESIAN_POINT ( 'NONE',  ( 35.59999999999998721, 27.13292387221364876, 93.11078899226573924 ) ) ;
#12133=CARTESIAN_POINT ( 'NONE',  ( 48.47500000054623115, 13.80429023900056684, 86.29171490190961435 ) ) ;
#12134=EDGE_LOOP ( 'NONE', ( #6743, #11857, #12137, #1053 ) ) ;
#12135=CARTESIAN_POINT ( 'NONE',  ( 23.65000000109246514, 20.00000000000000355, 98.29316153445363113 ) ) ;
#12137=ORIENTED_EDGE ( 'NONE', *, *, #6410, .T. ) ;
#12139=FACE_OUTER_BOUND ( 'NONE', #7942, .T. ) ;
#12141=CARTESIAN_POINT ( 'NONE',  ( 19.87500000054622262, 20.00000000000000355, 98.07665518445361386 ) ) ;
#12143=CARTESIAN_POINT ( 'NONE',  ( 35.65000000109246514, 20.00000000000000355, 98.29316153445363113 ) ) ;
#12146=CARTESIAN_POINT ( 'NONE',  ( 26.77500000054622831, 20.00000000000000355, 83.50966788445364841 ) ) ;
#12147=CARTESIAN_POINT ( 'NONE',  ( 22.37500000054622262, 12.34168156654572535, 90.79316153445363113 ) ) ;
#12150=CARTESIAN_POINT ( 'NONE',  ( 22.55000000109246017, 17.56310227825320425, 83.29316153445363113 ) ) ;
#12151=VERTEX_POINT ( 'NONE', #4606 ) ;
#12152=CARTESIAN_POINT ( 'NONE',  ( 41.25000000109246656, 27.13292387221364876, 93.11078899226573924 ) ) ;
#12154=ORIENTED_EDGE ( 'NONE', *, *, #3973, .T. ) ;
#12155=CARTESIAN_POINT ( 'NONE',  ( 30.45000000109246585, 15.59161060780646046, 84.72553407664153724 ) ) ;
#12157=EDGE_CURVE ( 'NONE', #10127, #949, #931, .T. ) ;
#12164=CARTESIAN_POINT ( 'NONE',  ( 49.99999999999998579, 20.00000000000000000, 137.5000000000000000 ) ) ;
#12170=ORIENTED_EDGE ( 'NONE', *, *, #10950, .F. ) ;
#12172=FACE_OUTER_BOUND ( 'NONE', #12385, .T. ) ;
#12175=CARTESIAN_POINT ( 'NONE',  ( 39.77500000054621410, 22.36655054427230027, 98.07665518445361386 ) ) ;
#12176=CARTESIAN_POINT ( 'NONE',  ( 26.17500000054623044, 13.07298590277314254, 93.04388485072563242 ) ) ;
#12177=CARTESIAN_POINT ( 'NONE',  ( 6.629305964221016367, 12.51308527848402896, 90.28034961326086716 ) ) ;
#12178=CARTESIAN_POINT ( 'NONE',  ( -50.00000000000001421, 0.000000000000000000, 169.9999999999999716 ) ) ;
#12180=EDGE_CURVE ( 'NONE', #10115, #8484, #7595, .T. ) ;
#12181=CARTESIAN_POINT ( 'NONE',  ( 35.39999999999998437, 27.13292387221364876, 88.47553407664153724 ) ) ;
#12182=CARTESIAN_POINT ( 'NONE',  ( 31.49999999999997868, 27.88596668178699645, 90.79316153445363113 ) ) ;
#12189=CARTESIAN_POINT ( 'NONE',  ( 30.67500000054622333, 15.71886984736413773, 84.90069139318163138 ) ) ;
#12191=CARTESIAN_POINT ( 'NONE',  ( 43.27500000054622831, 27.65831843345427998, 90.79316153445363113 ) ) ;
#12192=CARTESIAN_POINT ( 'NONE',  ( 34.49999999999998579, 12.11403331821300533, 90.79316153445363113 ) ) ;
#12193=EDGE_CURVE ( 'NONE', #1317, #4704, #997, .T. ) ;
#12194=LINE ( 'NONE', #3614, #6662 ) ;
#12195=CARTESIAN_POINT ( 'NONE',  ( 38.97500000054622404, 24.28113015263587471, 84.90069139318163138 ) ) ;
#12196=ORIENTED_EDGE ( 'NONE', *, *, #5914, .T. ) ;
#12197=CARTESIAN_POINT ( 'NONE',  ( 45.77500000054622831, 20.00000000000000355, 98.07665518445361386 ) ) ;
#12199=ORIENTED_EDGE ( 'NONE', *, *, #9618, .F. ) ;
#12206=CARTESIAN_POINT ( 'NONE',  ( 31.75000000109246656, 17.56310227825320425, 98.29316153445363113 ) ) ;
#12207=CARTESIAN_POINT ( 'NONE',  ( 21.27500000054622831, 27.65831843345427998, 90.79316153445363113 ) ) ;
#12208=CARTESIAN_POINT ( 'NONE',  ( 27.27500000054622475, 26.92701409722686634, 88.54243821818162985 ) ) ;
#12209=DIRECTION ( 'NONE',  ( 1.000000000000000000, 0.000000000000000000, 0.000000000000000000 ) ) ;
#12210=LINE ( 'NONE', #11442, #11922 ) ;
#12212=CARTESIAN_POINT ( 'NONE',  ( 42.15000000109246514, 12.11403331821300533, 90.79316153445363113 ) ) ;
#12214=ORIENTED_EDGE ( 'NONE', *, *, #2850, .F. ) ;
#12215=CARTESIAN_POINT ( 'NONE',  ( 47.29999999999997584, 26.37988106264029398, 86.15790661882942914 ) ) ;
#12216=VERTEX_POINT ( 'NONE', #9499 ) ;
#12226=CARTESIAN_POINT ( 'NONE',  ( 27.47500000054622404, 26.19570976099943493, 95.29460816699764791 ) ) ;
#12233=CARTESIAN_POINT ( 'NONE',  ( -50.00000000000001421, 22.00000000000000000, 188.4007504869563263 ) ) ;
#12234=CARTESIAN_POINT ( 'NONE',  ( 39.87500000054622262, 17.63344945572769973, 98.07665518445361386 ) ) ;
#12235=CARTESIAN_POINT ( 'NONE',  ( 35.47500000054622404, 26.92701409722686634, 93.04388485072563242 ) ) ;
#12237=CARTESIAN_POINT ( 'NONE',  ( 29.57500000054622546, 24.28113015263587116, 96.68563167572563088 ) ) ;
#12238=ADVANCED_FACE ( 'NONE', ( #9623 ), #1809, .T. ) ;
#12247=PLANE ( 'NONE',  #9694 ) ;
#12248=CARTESIAN_POINT ( 'NONE',  ( 34.87500000054622262, 20.00000000000000355, 83.50966788445364841 ) ) ;
#12250=CARTESIAN_POINT ( 'NONE',  ( 48.57500000054623257, 15.71886984736413773, 84.90069139318163138 ) ) ;
#12251=CARTESIAN_POINT ( 'NONE',  ( 33.27500000054622831, 26.92701409722686634, 88.54243821818162985 ) ) ;
#12252=CARTESIAN_POINT ( 'NONE',  ( 30.39999999999998792, 12.86707612778636012, 93.11078899226572503 ) ) ;
#12255=CARTESIAN_POINT ( 'NONE',  ( 37.27500000054622831, 27.65831843345427998, 90.79316153445363113 ) ) ;
#12258=CARTESIAN_POINT ( 'NONE',  ( 47.07500000054622546, 26.19570976099943493, 86.29171490190961435 ) ) ;
#12261=VECTOR ( 'NONE', #10812, 1000.000000000000000 ) ;
#12263=VERTEX_POINT ( 'NONE', #8601 ) ;
#12264=CARTESIAN_POINT ( 'NONE',  ( 42.55000000109246372, 17.56310227825321491, 83.29316153445364534 ) ) ;
#12265=CARTESIAN_POINT ( 'NONE',  ( -50.00000000000001421, 92.00000000000000000, 166.8533255156881694 ) ) ;
#12271=CARTESIAN_POINT ( 'NONE',  ( 25.57500000054622546, 24.28113015263587116, 96.68563167572563088 ) ) ;
#12272=CARTESIAN_POINT ( 'NONE',  ( 26.87500000054622618, 20.00000000000000355, 83.50966788445364841 ) ) ;
#12273=CARTESIAN_POINT ( 'NONE',  ( 41.39999999999999147, 27.13292387221364876, 88.47553407664153724 ) ) ;
#12276=EDGE_LOOP ( 'NONE', ( #7831, #5868, #2891, #4317 ) ) ;
#12277=VECTOR ( 'NONE', #1508, 1000.000000000000000 ) ;
#12278=CARTESIAN_POINT ( 'NONE',  ( 35.85000000109246798, 15.59161060780645691, 96.86078899226572503 ) ) ;
#12279=CARTESIAN_POINT ( 'NONE',  ( 24.79999999999999005, 15.59161060780646046, 84.72553407664153724 ) ) ;
#12280=ORIENTED_EDGE ( 'NONE', *, *, #10783, .T. ) ;
#12281=CARTESIAN_POINT ( 'NONE',  ( 47.89999999999997726, 22.43689772174681707, 98.29316153445361692 ) ) ;
#12287=CARTESIAN_POINT ( 'NONE',  ( 27.69999999999998508, 26.37988106264029398, 95.42841645007781892 ) ) ;
#12289=CYLINDRICAL_SURFACE ( 'NONE', #4116, 10.00000000000000355 ) ;
#12290=CARTESIAN_POINT ( 'NONE',  ( 20.97500000054622760, 24.28113015263587471, 84.90069139318163138 ) ) ;
#12293=ORIENTED_EDGE ( 'NONE', *, *, #7144, .T. ) ;
#12295=DIRECTION ( 'NONE',  ( 0.000000000000000000, 0.000000000000000000, 1.000000000000000000 ) ) ;
#12297=CARTESIAN_POINT ( 'NONE',  ( 34.67500000054621268, 17.63344945572770328, 83.50966788445364841 ) ) ;
#12298=CARTESIAN_POINT ( 'NONE',  ( 37.87500000054622262, 20.00000000000000355, 98.07665518445361386 ) ) ;
#12303=CARTESIAN_POINT ( 'NONE',  ( -36.00000000000001421, 77.00000000000000000, 154.3533255156881978 ) ) ;
#12305=ORIENTED_EDGE ( 'NONE', *, *, #11312, .F. ) ;
#12309=CARTESIAN_POINT ( 'NONE',  ( 25.77500000054622475, 22.36655054427230027, 98.07665518445361386 ) ) ;
#12310=CARTESIAN_POINT ( 'NONE',  ( 28.75000000109245946, 22.43689772174679575, 83.29316153445363113 ) ) ;
#12312=CARTESIAN_POINT ( 'NONE',  ( 47.57500000054622546, 24.28113015263587116, 96.68563167572563088 ) ) ;
#12313=CARTESIAN_POINT ( 'NONE',  ( 26.37500000054622618, 12.34168156654572535, 90.79316153445363113 ) ) ;
#12314=CARTESIAN_POINT ( 'NONE',  ( 27.39999999999998792, 27.13292387221364876, 88.47553407664153724 ) ) ;
#12316=CARTESIAN_POINT ( 'NONE',  ( 36.47500000054622404, 13.80429023900056684, 86.29171490190961435 ) ) ;
#12318=CARTESIAN_POINT ( 'NONE',  ( 48.77500000054622831, 20.00000000000000355, 83.50966788445364841 ) ) ;
#12322=ORIENTED_EDGE ( 'NONE', *, *, #4904, .F. ) ;
#12325=DIRECTION ( 'NONE',  ( 1.000000000000000000, 0.000000000000000000, 0.000000000000000000 ) ) ;
#12326=PLANE ( 'NONE',  #3796 ) ;
#12328=DIRECTION ( 'NONE',  ( -1.000000000000000000, 0.000000000000000000, 0.000000000000000000 ) ) ;
#12330=CARTESIAN_POINT ( 'NONE',  ( 24.97500000054622760, 24.28113015263587471, 84.90069139318163138 ) ) ;
#12331=CARTESIAN_POINT ( 'NONE',  ( 20.37500000054621907, 12.34168156654572535, 90.79316153445363113 ) ) ;
#12333=( BOUNDED_CURVE ( )  B_SPLINE_CURVE ( 2, ( #1405, #4561, #9204, #3544, #5270, #12182, #11287, #7351, #6402, #10267, #2350 ),
 .UNSPECIFIED., .F., .F. ) 
 B_SPLINE_CURVE_WITH_KNOTS ( ( 3, 2, 2, 2, 2, 3 ),
 ( 0.5999999999999999778, 0.6066666666666666874, 0.6133333333333332860, 0.6199999999999999956, 0.6266666666666667052, 0.6333333333333333037 ),
 .UNSPECIFIED. ) 
 CURVE ( )  GEOMETRIC_REPRESENTATION_ITEM ( )  RATIONAL_B_SPLINE_CURVE ( ( 1.000000000000000000, 0.9510565162951535312, 1.000000000000000000, 0.9510565162951535312, 1.000000000000000000, 0.9510565162951535312, 1.000000000000000000, 0.9510565162951535312, 1.000000000000000000, 0.9510565162951535312, 1.000000000000000000 ) ) 
 REPRESENTATION_ITEM ( '' )  );
#12337=CARTESIAN_POINT ( 'NONE',  ( 38.05000000109246372, 12.86707612778636012, 93.11078899226572503 ) ) ;
#12338=CARTESIAN_POINT ( 'NONE',  ( 24.69999999999998508, 13.62011893735970958, 86.15790661882942914 ) ) ;
#12340=CARTESIAN_POINT ( 'NONE',  ( -36.00000000000001421, 77.00000000000000000, 166.8533255156881694 ) ) ;
#12347=DIRECTION ( 'NONE',  ( 0.000000000000000000, -1.000000000000000000, 0.000000000000000000 ) ) ;
#12348=EDGE_LOOP ( 'NONE', ( #5866, #8221, #9755, #6691, #3348 ) ) ;
#12350=EDGE_CURVE ( 'NONE', #10641, #10590, #7335, .T. ) ;
#12352=CARTESIAN_POINT ( 'NONE',  ( 19.87500000054622973, 17.63344945572769973, 98.07665518445361386 ) ) ;
#12355=VERTEX_POINT ( 'NONE', #12141 ) ;
#12356=ORIENTED_EDGE ( 'NONE', *, *, #7359, .T. ) ;
#12361=CARTESIAN_POINT ( 'NONE',  ( 38.97500000054623115, 22.36655054427230382, 83.50966788445364841 ) ) ;
#12362=CARTESIAN_POINT ( 'NONE',  ( 21.37500000054622618, 26.92701409722686634, 93.04388485072563242 ) ) ;
#12373=CARTESIAN_POINT ( 'NONE',  ( 26.67500000054622333, 15.71886984736413773, 84.90069139318163138 ) ) ;
#12374=CARTESIAN_POINT ( 'NONE',  ( 29.65000000109246514, 20.00000000000000355, 98.29316153445363113 ) ) ;
#12375=CARTESIAN_POINT ( 'NONE',  ( 40.97500000054622404, 24.28113015263587471, 84.90069139318163138 ) ) ;
#12376=CARTESIAN_POINT ( 'NONE',  ( 28.77500000054622831, 17.63344945572770328, 83.50966788445364841 ) ) ;
#12377=CARTESIAN_POINT ( 'NONE',  ( 30.79999999999998650, 15.59161060780646046, 84.72553407664153724 ) ) ;
#12379=CARTESIAN_POINT ( 'NONE',  ( 30.49999999999998934, 12.11403331821300533, 90.79316153445363113 ) ) ;
#12381=CARTESIAN_POINT ( 'NONE',  ( 37.77500000054623541, 20.00000000000000355, 98.07665518445361386 ) ) ;
#12383=CARTESIAN_POINT ( 'NONE',  ( 21.05000000109246727, 27.13292387221364876, 88.47553407664153724 ) ) ;
#12385=EDGE_LOOP ( 'NONE', ( #11384, #1904 ) ) ;
#12386=CARTESIAN_POINT ( 'NONE',  ( -50.00000000000001421, 84.49999999999998579, 146.8533255156881978 ) ) ;
#12388=LINE ( 'NONE', #1845, #11440 ) ;
#12389=CARTESIAN_POINT ( 'NONE',  ( 43.99999999999999289, 20.00000000000000355, 98.29316153445363113 ) ) ;
#12391=CARTESIAN_POINT ( 'NONE',  ( 42.27500000054622120, 13.07298590277314254, 93.04388485072563242 ) ) ;
#12392=DIRECTION ( 'NONE',  ( 0.000000000000000000, 0.000000000000000000, -1.000000000000000000 ) ) ;
#12393=CARTESIAN_POINT ( 'NONE',  ( 21.57500000054622546, 26.19570976099943493, 95.29460816699764791 ) ) ;
#12397=CARTESIAN_POINT ( 'NONE',  ( 40.65000000109246514, 20.00000000000000355, 83.29316153445364534 ) ) ;
#12398=DIRECTION ( 'NONE',  ( -0.000000000000000000, 0.7071067811865511255, 0.7071067811865440200 ) ) ;
#12400=LINE ( 'NONE', #10607, #10837 ) ;
#12401=EDGE_CURVE ( 'NONE', #8586, #10504, #6009, .T. ) ;
#12402=VERTEX_POINT ( 'NONE', #8858 ) ;
#12403=CARTESIAN_POINT ( 'NONE',  ( -2.000000000000015543, 20.00000000000000355, 83.29316153445364534 ) ) ;
#12404=CARTESIAN_POINT ( 'NONE',  ( 30.85000000109246443, 24.40838939219355197, 84.72553407664153724 ) ) ;
#12405=DIRECTION ( 'NONE',  ( 1.000000000000000000, -0.000000000000000000, -0.000000000000000000 ) ) ;
#12406=( BOUNDED_CURVE ( )  B_SPLINE_CURVE ( 2, ( #8675, #1009, #4613, #8735, #11593, #1751, #48, #3911, #11528, #10694, #8551 ),
 .UNSPECIFIED., .F., .F. ) 
 B_SPLINE_CURVE_WITH_KNOTS ( ( 3, 2, 2, 2, 2, 3 ),
 ( 0.1999999999999999278, 0.2066666666666665819, 0.2133333333333332915, 0.2199999999999999456, 0.2266666666666666274, 0.2333333333333333093 ),
 .UNSPECIFIED. ) 
 CURVE ( )  GEOMETRIC_REPRESENTATION_ITEM ( )  RATIONAL_B_SPLINE_CURVE ( ( 1.000000000000000666, 0.9510565162951528650, 1.000000000000000000, 0.9510565162951535312, 1.000000000000000000, 0.9510565162951535312, 1.000000000000000000, 0.9510565162951535312, 1.000000000000000000, 0.9510565162951537532, 0.9999999999999997780 ) ) 
 REPRESENTATION_ITEM ( '' )  );
#12409=ORIENTED_EDGE ( 'NONE', *, *, #737, .F. ) ;
#12411=DIRECTION ( 'NONE',  ( -1.000000000000000000, 0.000000000000000000, 0.000000000000000000 ) ) ;
#12412=CARTESIAN_POINT ( 'NONE',  ( 23.47500000054623115, 26.19570976099943493, 95.29460816699764791 ) ) ;
#12415=ORIENTED_EDGE ( 'NONE', *, *, #9869, .F. ) ;
#12416=VERTEX_POINT ( 'NONE', #2489 ) ;
#12418=CYLINDRICAL_SURFACE ( 'NONE', #10868, 7.499999999999978684 ) ;
#12419=ADVANCED_FACE ( 'NONE', ( #11778 ), #533, .F. ) ;
#12420=CARTESIAN_POINT ( 'NONE',  ( -50.00000000000001421, 20.00000000000000000, 137.5000000000000000 ) ) ;
#12422=CARTESIAN_POINT ( 'NONE',  ( 28.65000000109246514, 20.00000000000000355, 83.29316153445364534 ) ) ;
#12428=CARTESIAN_POINT ( 'NONE',  ( -50.00000000000001421, 18.00000000000000355, 152.2284161474004520 ) ) ;
#12433=AXIS2_PLACEMENT_3D ( 'NONE', #6670, #5672, #719 ) ;
#12434=CARTESIAN_POINT ( 'NONE',  ( 28.57500000054622191, 13.80429023900056684, 86.29171490190961435 ) ) ;
#12435=CARTESIAN_POINT ( 'NONE',  ( 36.69999999999999574, 13.62011893735970958, 86.15790661882942914 ) ) ;
#12437=CARTESIAN_POINT ( 'NONE',  ( 36.47500000054622404, 13.80429023900056684, 86.29171490190961435 ) ) ;
#12438=CARTESIAN_POINT ( 'NONE',  ( 30.07500000054622546, 15.71886984736413417, 96.68563167572563088 ) ) ;
#12439=CARTESIAN_POINT ( 'NONE',  ( 30.59999999999998721, 12.86707612778636012, 88.47553407664152303 ) ) ;
#12440=CARTESIAN_POINT ( 'NONE',  ( 29.99999999999998934, 20.00000000000000355, 98.29316153445363113 ) ) ;
#12441=CARTESIAN_POINT ( 'NONE',  ( 40.17500000054623399, 13.07298590277314254, 93.04388485072563242 ) ) ;
#12442=ORIENTED_EDGE ( 'NONE', *, *, #10633, .T. ) ;
#12443=CARTESIAN_POINT ( 'NONE',  ( 47.97500000054622404, 15.71886984736413417, 96.68563167572563088 ) ) ;
#12445=ORIENTED_EDGE ( 'NONE', *, *, #4626, .T. ) ;
#12448=CARTESIAN_POINT ( 'NONE',  ( 41.95000000109246230, 13.62011893735970958, 95.42841645007781892 ) ) ;
#12451=CARTESIAN_POINT ( 'NONE',  ( 46.37500000054621552, 12.34168156654572357, 90.79316153445363113 ) ) ;
#12452=CARTESIAN_POINT ( 'NONE',  ( 20.79999999999999005, 15.59161060780646046, 84.72553407664153724 ) ) ;
#12454=CARTESIAN_POINT ( 'NONE',  ( 46.09999999999998010, 17.56310227825320425, 98.29316153445363113 ) ) ;
#12455=CARTESIAN_POINT ( 'NONE',  ( 41.29999999999999005, 26.37988106264029398, 86.15790661882942914 ) ) ;
#12456=LINE ( 'NONE', #9423, #9895 ) ;
#12457=VERTEX_POINT ( 'NONE', #3084 ) ;
#12458=CARTESIAN_POINT ( 'NONE',  ( 38.15000000109245804, 12.11403331821300533, 90.79316153445363113 ) ) ;
#12460=EDGE_LOOP ( 'NONE', ( #4915, #6699, #8791, #10606 ) ) ;
#12465=ADVANCED_FACE ( 'NONE', ( #10233 ), #1545, .F. ) ;
#12466=LINE ( 'NONE', #4792, #4327 ) ;
#12467=VECTOR ( 'NONE', #556, 1000.000000000000000 ) ;
#12469=CARTESIAN_POINT ( 'NONE',  ( 27.79999999999998650, 24.40838939219354842, 96.86078899226572503 ) ) ;
#12470=ORIENTED_EDGE ( 'NONE', *, *, #10824, .T. ) ;
#12472=DIRECTION ( 'NONE',  ( -0.000000000000000000, 1.000000000000000000, 0.000000000000000000 ) ) ;
#12473=CARTESIAN_POINT ( 'NONE',  ( 23.07500000054622902, 26.19570976099943493, 86.29171490190961435 ) ) ;
#12478=ORIENTED_EDGE ( 'NONE', *, *, #8470, .T. ) ;
#12482=CARTESIAN_POINT ( 'NONE',  ( 22.07500000054622191, 13.80429023900056507, 95.29460816699764791 ) ) ;
#12485=CARTESIAN_POINT ( 'NONE',  ( -50.00000000000001421, 77.00000000000000000, 146.8533255156881978 ) ) ;
#12488=CARTESIAN_POINT ( 'NONE',  ( -20.27158385259951956, 18.00000000000000355, 169.9999999999999716 ) ) ;
#12489=ORIENTED_EDGE ( 'NONE', *, *, #9053, .F. ) ;
#12490=CARTESIAN_POINT ( 'NONE',  ( 19.99999999999999645, 20.00000000000000355, 99.99999999999997158 ) ) ;
#12493=CARTESIAN_POINT ( 'NONE',  ( 27.37500000054622262, 27.65831843345427998, 90.79316153445363113 ) ) ;
#12496=CARTESIAN_POINT ( 'NONE',  ( 40.67500000054623399, 17.63344945572770328, 83.50966788445364841 ) ) ;
#12497=CARTESIAN_POINT ( 'NONE',  ( 25.17500000054622689, 26.19570976099943493, 86.29171490190961435 ) ) ;
#12498=CARTESIAN_POINT ( 'NONE',  ( 32.49999999999997868, 12.11403331821300533, 90.79316153445363113 ) ) ;
#12499=CARTESIAN_POINT ( 'NONE',  ( 30.59999999999998721, 12.86707612778636012, 88.47553407664152303 ) ) ;
#12500=CARTESIAN_POINT ( 'NONE',  ( 32.37500000054622973, 13.07298590277314432, 88.54243821818161564 ) ) ;
#12502=EDGE_CURVE ( 'NONE', #12216, #7706, #11715, .T. ) ;
#12503=CARTESIAN_POINT ( 'NONE',  ( -6.999999999999999112, 92.00000000000000000, 69.99999999999998579 ) ) ;
#12504=AXIS2_PLACEMENT_3D ( 'NONE', #8397, #10413, #1727 ) ;
#12510=FACE_OUTER_BOUND ( 'NONE', #9782, .T. ) ;
#12512=CARTESIAN_POINT ( 'NONE',  ( 46.87500000054622262, 20.00000000000000355, 83.50966788445364841 ) ) ;
#12515=CARTESIAN_POINT ( 'NONE',  ( -2.000000000000015543, 20.00000000000000355, 98.29316153445363113 ) ) ;
#12516=CARTESIAN_POINT ( 'NONE',  ( 46.07500000054622546, 15.71886984736413417, 96.68563167572563088 ) ) ;
#12517=CARTESIAN_POINT ( 'NONE',  ( 46.49999999999999289, 12.11403331821300533, 90.79316153445363113 ) ) ;
#12519=CARTESIAN_POINT ( 'NONE',  ( 49.37500000054622973, 26.92701409722686634, 93.04388485072563242 ) ) ;
#12521=CARTESIAN_POINT ( 'NONE',  ( 36.25000000109246656, 12.86707612778636012, 88.47553407664152303 ) ) ;
#12522=EDGE_LOOP ( 'NONE', ( #7001, #4034, #7967, #8855 ) ) ;
#12523=PLANE ( 'NONE',  #3540 ) ;
#12529=CARTESIAN_POINT ( 'NONE',  ( 37.17500000054622689, 26.92701409722686634, 88.54243821818162985 ) ) ;
#12531=CARTESIAN_POINT ( 'NONE',  ( 31.65000000109246514, 20.00000000000000355, 98.29316153445363113 ) ) ;
#12532=ORIENTED_EDGE ( 'NONE', *, *, #10684, .F. ) ;
#12534=CYLINDRICAL_SURFACE ( 'NONE', #11016, 7.499999999999992895 ) ;
#12535=CARTESIAN_POINT ( 'NONE',  ( 21.07500000054622546, 26.19570976099943493, 86.29171490190961435 ) ) ;
#12538=UNCERTAINTY_MEASURE_WITH_UNIT (LENGTH_MEASURE( 1.000000000000000082E-05 ), #11679, 'distance_accuracy_value', 'NONE');
#12539=DIRECTION ( 'NONE',  ( 0.000000000000000000, 0.000000000000000000, -1.000000000000000000 ) ) ;
#12541=EDGE_CURVE ( 'NONE', #1127, #5241, #12388, .T. ) ;
#12578=COLOUR_RGB('Grey',0.48,0.52,0.57);
#12579=FILL_AREA_STYLE_COLOUR('',#12578);
#12580=FILL_AREA_STYLE('',(#12579));
#12581=SURFACE_STYLE_FILL_AREA(#12580);
#12582=SURFACE_SIDE_STYLE('',(#12581));
#12583=SURFACE_STYLE_USAGE(.BOTH.,#12582);
#12584=PRESENTATION_STYLE_ASSIGNMENT((#12583));
ENDSEC;
END-ISO-10303-21;
